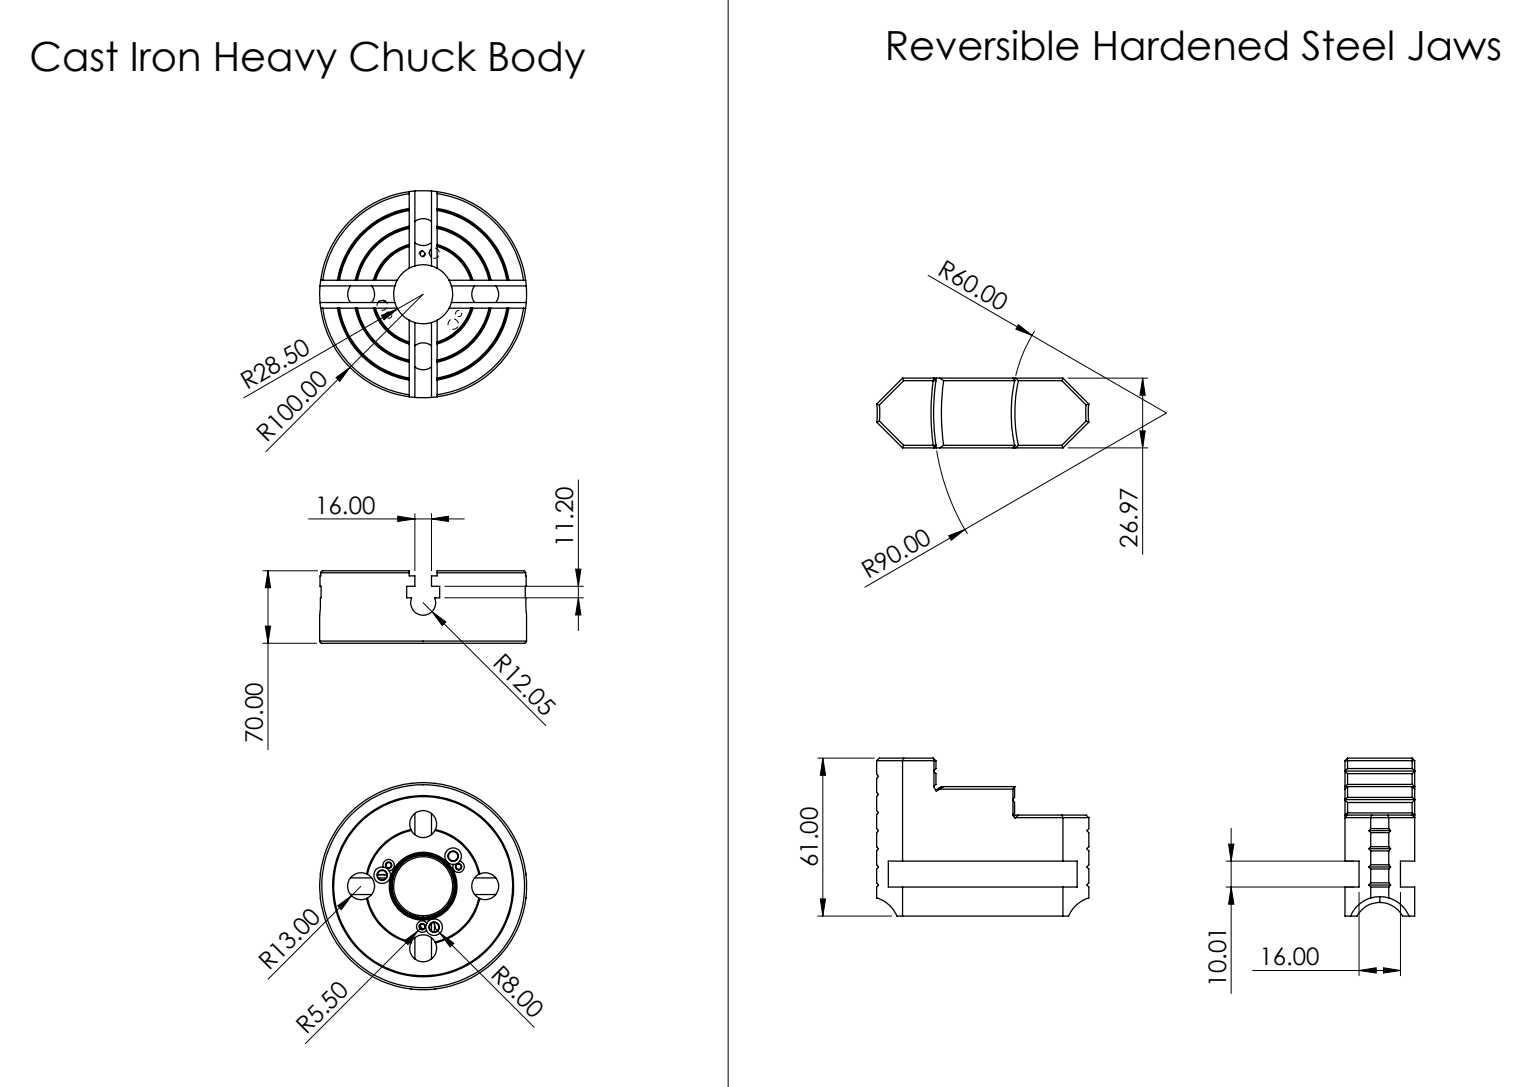
ISO-10303-21;
HEADER;
FILE_DESCRIPTION (('STEP AP214'),
    '1' );
FILE_NAME ('Cast Iron Heavy Chuck Body.step',
    '2026-10-09T08:48:44',
    ( '' ),
    ( '' ),
    'SwSTEP 2.0',
    'SolidWorks 2026',
    '' );
FILE_SCHEMA (( 'AUTOMOTIVE_DESIGN' ));
ENDSEC;

DATA;
#17=CARTESIAN_POINT ( 'NONE',  ( 3.210901138312283187, 2.729659904327170317, 0.5314960629921260393 ) ) ;
#22=EDGE_CURVE ( 'NONE', #75161, #32355, #82357, .T. ) ;
#61=ORIENTED_EDGE ( 'NONE', *, *, #30614, .T. ) ;
#78=FACE_OUTER_BOUND ( 'NONE', #30932, .T. ) ;
#83=ORIENTED_EDGE ( 'NONE', *, *, #43269, .T. ) ;
#95=CARTESIAN_POINT ( 'NONE',  ( 2.362204724409448620, 1.724409448818897461, 8.247593713802677664E-15 ) ) ;
#97=CARTESIAN_POINT ( 'NONE',  ( 3.935554666754304876, 1.075197191891656523, -0.1080298857917176142 ) ) ;
#98=EDGE_LOOP ( 'NONE', ( #67193, #53701, #56792, #76408 ) ) ;
#137=CARTESIAN_POINT ( 'NONE',  ( 1.067341128551216878, 1.212753000281105331, 0.3462674622822208836 ) ) ;
#152=CIRCLE ( 'NONE', #29714, 0.3149606299212598381 ) ;
#153=EDGE_CURVE ( 'NONE', #58154, #38787, #62911, .T. ) ;
#192=CIRCLE ( 'NONE', #6913, 0.3149606299212597826 ) ;
#213=ORIENTED_EDGE ( 'NONE', *, *, #72282, .F. ) ;
#238=EDGE_CURVE ( 'NONE', #62570, #82725, #55742, .T. ) ;
#251=AXIS2_PLACEMENT_3D ( 'NONE', #31198, #57691, #45055 ) ;
#278=EDGE_LOOP ( 'NONE', ( #70982, #45636, #76392, #46329 ) ) ;
#294=ORIENTED_EDGE ( 'NONE', *, *, #5614, .T. ) ;
#302=EDGE_CURVE ( 'NONE', #13567, #50475, #28771, .T. ) ;
#303=LINE ( 'NONE', #76901, #13349 ) ;
#312=VERTEX_POINT ( 'NONE', #80938 ) ;
#316=TOROIDAL_SURFACE ( 'NONE', #58028, 1.178877988035069047, 0.01968503937007873988 ) ;
#321=CARTESIAN_POINT ( 'NONE',  ( 2.165589143934496530, 1.494558157769224405, 0.4725443725032424380 ) ) ;
#334=CARTESIAN_POINT ( 'NONE',  ( -0.09693039542137318887, 1.072949718929360641, -1.590986883761158932 ) ) ;
#346=CARTESIAN_POINT ( 'NONE',  ( -1.024276469446319116, 1.664626768191372896, -0.4581463608586889835 ) ) ;
#368=ORIENTED_EDGE ( 'NONE', *, *, #43225, .F. ) ;
#369=CARTESIAN_POINT ( 'NONE',  ( 0.3149606299212637239, 2.165354330708661568, -1.076935383196056417 ) ) ;
#374=DIRECTION ( 'NONE',  ( 0.000000000000000000, -0.000000000000000000, 1.000000000000000000 ) ) ;
#377=CARTESIAN_POINT ( 'NONE',  ( 0.06179655389848991154, 1.065998012190817246, -3.936642156184892105 ) ) ;
#381=ORIENTED_EDGE ( 'NONE', *, *, #63426, .T. ) ;
#397=ORIENTED_EDGE ( 'NONE', *, *, #78869, .T. ) ;
#429=VECTOR ( 'NONE', #73458, 39.37007874015748143 ) ;
#436=DIRECTION ( 'NONE',  ( 0.000000000000000000, 1.000000000000000000, 0.000000000000000000 ) ) ;
#459=CARTESIAN_POINT ( 'NONE',  ( 0.4359958488159310086, 1.724409448818897461, 3.912791665790203766 ) ) ;
#472=CARTESIAN_POINT ( 'NONE',  ( -0.6299212598425164567, 2.165354330708661568, -0.9285414500055735321 ) ) ;
#483=CIRCLE ( 'NONE', #78489, 0.3149606299212597271 ) ;
#491=DIRECTION ( 'NONE',  ( 0.000000000000000000, 0.000000000000000000, -1.000000000000000000 ) ) ;
#502=CARTESIAN_POINT ( 'NONE',  ( -0.4477342634306575864, 1.379855024864608204, -2.114057166015708589 ) ) ;
#511=EDGE_CURVE ( 'NONE', #3191, #62716, #18015, .T. ) ;
#523=ORIENTED_EDGE ( 'NONE', *, *, #53975, .F. ) ;
#619=EDGE_LOOP ( 'NONE', ( #4517, #46542, #69561, #51297 ) ) ;
#623=DIRECTION ( 'NONE',  ( 0.000000000000000000, 1.000000000000000000, 0.000000000000000000 ) ) ;
#635=CARTESIAN_POINT ( 'NONE',  ( 0.1273213304869930951, 0.1377952755905511861, -1.680969278250197707 ) ) ;
#641=CARTESIAN_POINT ( 'NONE',  ( 0.000000000000000000, 2.677165354330708791, 0.000000000000000000 ) ) ;
#685=CARTESIAN_POINT ( 'NONE',  ( 0.4602852883866460076, 1.653403552777538366, 2.586150256253575197 ) ) ;
#697=ORIENTED_EDGE ( 'NONE', *, *, #58155, .F. ) ;
#698=ORIENTED_EDGE ( 'NONE', *, *, #49898, .F. ) ;
#712=VERTEX_POINT ( 'NONE', #12515 ) ;
#714=ORIENTED_EDGE ( 'NONE', *, *, #48541, .F. ) ;
#716=CONICAL_SURFACE ( 'NONE', #24907, 0.1771653543307085410, 1.029744258676653645 ) ;
#723=CARTESIAN_POINT ( 'NONE',  ( 3.224202737261815166, 2.716535433070866645, 0.5314960629921260393 ) ) ;
#725=AXIS2_PLACEMENT_3D ( 'NONE', #34776, #73071, #41496 ) ;
#733=EDGE_CURVE ( 'NONE', #7205, #57884, #50385, .T. ) ;
#741=CARTESIAN_POINT ( 'NONE',  ( -2.152447471807442891, 1.622068519643041551, 0.4668652553835654917 ) ) ;
#743=DIRECTION ( 'NONE',  ( 0.000000000000000000, 0.000000000000000000, 1.000000000000000000 ) ) ;
#754=CARTESIAN_POINT ( 'NONE',  ( 1.141392835773559211, 1.299212598425196985, 0.9642274814428540841 ) ) ;
#766=PLANE ( 'NONE',  #65364 ) ;
#772=DIRECTION ( 'NONE',  ( 0.000000000000000000, 0.000000000000000000, 1.000000000000000000 ) ) ;
#779=VECTOR ( 'NONE', #35095, 39.37007874015748143 ) ;
#790=ADVANCED_FACE ( 'NONE', ( #76083 ), #69761, .F. ) ;
#803=ORIENTED_EDGE ( 'NONE', *, *, #65634, .F. ) ;
#805=ORIENTED_EDGE ( 'NONE', *, *, #65450, .T. ) ;
#822=AXIS2_PLACEMENT_3D ( 'NONE', #34394, #67220, #78191 ) ;
#825=AXIS2_PLACEMENT_3D ( 'NONE', #7918, #52916, #78631 ) ;
#828=CARTESIAN_POINT ( 'NONE',  ( 2.750540364621160361, 1.199841186584418518, -0.3336616047370271065 ) ) ;
#858=CARTESIAN_POINT ( 'NONE',  ( -0.5314960629921122726, 2.755905511811024056, -3.937007874015763687 ) ) ;
#876=DIRECTION ( 'NONE',  ( -0.000000000000000000, -1.000000000000000000, 0.000000000000000000 ) ) ;
#884=AXIS2_PLACEMENT_3D ( 'NONE', #26992, #71617, #52655 ) ;
#886=AXIS2_PLACEMENT_3D ( 'NONE', #7786, #38921, #40179 ) ;
#890=EDGE_CURVE ( 'NONE', #78998, #7122, #78646, .T. ) ;
#901=CARTESIAN_POINT ( 'NONE',  ( 0.4359958488159797474, 1.724409448818897905, -2.094141031014984833 ) ) ;
#929=ORIENTED_EDGE ( 'NONE', *, *, #10585, .T. ) ;
#932=EDGE_LOOP ( 'NONE', ( #23051, #15115, #31365, #8595 ) ) ;
#945=CARTESIAN_POINT ( 'NONE',  ( -0.5314960629921398061, 2.687614851728676424, 3.900966923095589234 ) ) ;
#946=CONICAL_SURFACE ( 'NONE', #61424, 1.250000000000000000, 0.1221730476396033355 ) ;
#948=DIRECTION ( 'NONE',  ( -0.000000000000000000, -1.000000000000000000, -0.000000000000000000 ) ) ;
#950=AXIS2_PLACEMENT_3D ( 'NONE', #7471, #12953, #25977 ) ;
#962=DIRECTION ( 'NONE',  ( 0.000000000000000000, 0.000000000000000000, -1.000000000000000000 ) ) ;
#984=B_SPLINE_CURVE_WITH_KNOTS ( 'NONE', 3,
 ( #68449, #81500, #10385, #37680, #36449, #62954, #50304, #24225, #61714, #57026, #56618, #36863 ),
 .UNSPECIFIED., .F., .F.,
 ( 4, 2, 2, 2, 2, 4 ),
 ( 0.007992874908875213444, 0.009303755029337302043, 0.01061463514979939064, 0.01192551527026147924, 0.01258095533049252354, 0.01323639539072356784 ),
 .UNSPECIFIED. ) ;
#986=CARTESIAN_POINT ( 'NONE',  ( 1.019692277575655615, 1.459399361446979126, -0.4682193611689622892 ) ) ;
#989=CARTESIAN_POINT ( 'NONE',  ( 0.4116877677584974138, 1.299622705822838453, 3.915462153828698888 ) ) ;
#995=ADVANCED_FACE ( 'NONE', ( #71847 ), #78589, .F. ) ;
#1024=CARTESIAN_POINT ( 'NONE',  ( 4.821444151489972621E-16, 1.062992125984252745, 3.937007874015748143 ) ) ;
#1043=ORIENTED_EDGE ( 'NONE', *, *, #78852, .T. ) ;
#1046=DIRECTION ( 'NONE',  ( 0.000000000000000000, -0.000000000000000000, 1.000000000000000000 ) ) ;
#1047=DIRECTION ( 'NONE',  ( 1.492469013153037857E-17, -0.9925461516413219831, 0.1218693434051477398 ) ) ;
#1048=FACE_OUTER_BOUND ( 'NONE', #12186, .T. ) ;
#1052=CARTESIAN_POINT ( 'NONE',  ( 0.4711392887345147162, 1.601500657493326152, -3.908721069869979026 ) ) ;
#1055=VERTEX_POINT ( 'NONE', #7876 ) ;
#1092=FACE_OUTER_BOUND ( 'NONE', #21318, .T. ) ;
#1095=CARTESIAN_POINT ( 'NONE',  ( 0.000000000000000000, 2.755905511811024056, 0.000000000000000000 ) ) ;
#1124=ORIENTED_EDGE ( 'NONE', *, *, #39342, .F. ) ;
#1130=DIRECTION ( 'NONE',  ( 0.000000000000000000, -0.6427876096865366984, -0.7660444431189802339 ) ) ;
#1139=ORIENTED_EDGE ( 'NONE', *, *, #22849, .T. ) ;
#1159=ORIENTED_EDGE ( 'NONE', *, *, #69637, .F. ) ;
#1166=LINE ( 'NONE', #52475, #66762 ) ;
#1174=DIRECTION ( 'NONE',  ( -0.000000000000000000, 1.734723475976808327E-16, 1.000000000000000000 ) ) ;
#1187=B_SPLINE_CURVE_WITH_KNOTS ( 'NONE', 3,
 ( #54995, #8742, #74380, #67239 ),
 .UNSPECIFIED., .F., .F.,
 ( 4, 4 ),
 ( 0.1688788475280605661, 0.1702663099542993941 ),
 .UNSPECIFIED. ) ;
#1196=CARTESIAN_POINT ( 'NONE',  ( 3.937007874015748143, 2.559055118110236560, 0.5314960629921260393 ) ) ;
#1207=CARTESIAN_POINT ( 'NONE',  ( -3.937007874015748143, 1.537401574803149984, -2.901595197523589142E-16 ) ) ;
#1214=FACE_BOUND ( 'NONE', #26809, .T. ) ;
#1220=FACE_OUTER_BOUND ( 'NONE', #57084, .T. ) ;
#1221=EDGE_CURVE ( 'NONE', #16864, #33327, #33540, .T. ) ;
#1224=CARTESIAN_POINT ( 'NONE',  ( 0.4622706148242299307, 1.429654486764701193, -3.909775711958814348 ) ) ;
#1240=EDGE_CURVE ( 'NONE', #12200, #44534, #303, .T. ) ;
#1245=ORIENTED_EDGE ( 'NONE', *, *, #82772, .T. ) ;
#1248=CARTESIAN_POINT ( 'NONE',  ( 2.759994995438110443, 1.188885443925058238, 0.3231744412229853869 ) ) ;
#1287=DIRECTION ( 'NONE',  ( -1.000000000000000000, -0.000000000000000000, -0.000000000000000000 ) ) ;
#1306=DIRECTION ( 'NONE',  ( 0.000000000000000000, 0.000000000000000000, -1.000000000000000000 ) ) ;
#1318=CARTESIAN_POINT ( 'NONE',  ( 0.5314960629921156032, 0.000000000000000000, 0.9881811337016697117 ) ) ;
#1323=CARTESIAN_POINT ( 'NONE',  ( 1.348312163386739426, 1.062992125984252079, 0.7386866130305692613 ) ) ;
#1327=ORIENTED_EDGE ( 'NONE', *, *, #22709, .T. ) ;
#1330=ORIENTED_EDGE ( 'NONE', *, *, #56817, .F. ) ;
#1345=EDGE_LOOP ( 'NONE', ( #66456, #45202, #47720, #72344 ) ) ;
#1362=CARTESIAN_POINT ( 'NONE',  ( 3.915483736577200613, 1.300266479744685899, -0.4111838468780947276 ) ) ;
#1367=CARTESIAN_POINT ( 'NONE',  ( 0.6299212598425235621, 0.000000000000000000, -0.9285414500055687581 ) ) ;
#1370=EDGE_CURVE ( 'NONE', #22431, #62933, #19231, .T. ) ;
#1388=CARTESIAN_POINT ( 'NONE',  ( 0.5314960629921070545, 2.755905511811024056, 1.813482582612299110 ) ) ;
#1433=CARTESIAN_POINT ( 'NONE',  ( -0.4724922890202599146, 1.580837543196282446, -2.165463280039293892 ) ) ;
#1456=DIRECTION ( 'NONE',  ( -1.687538997430237941E-14, 0.000000000000000000, -1.000000000000000000 ) ) ;
#1457=CARTESIAN_POINT ( 'NONE',  ( -0.008542603271839102619, 1.062992125984252301, 2.874015748031496731 ) ) ;
#1465=ORIENTED_EDGE ( 'NONE', *, *, #46764, .T. ) ;
#1468=CARTESIAN_POINT ( 'NONE',  ( -1.074107865122115868, 1.191152302059476087, -0.3246720348184669591 ) ) ;
#1477=CARTESIAN_POINT ( 'NONE',  ( -0.5314960629921193780, 2.755905511811024056, -1.895394334970793793 ) ) ;
#1494=FACE_OUTER_BOUND ( 'NONE', #73999, .T. ) ;
#1523=CARTESIAN_POINT ( 'NONE',  ( 0.2491324880211018833, 1.133662664435919787, -1.613879522126778543 ) ) ;
#1535=ORIENTED_EDGE ( 'NONE', *, *, #67469, .T. ) ;
#1542=CIRCLE ( 'NONE', #5549, 0.2165354330708660069 ) ;
#1551=ORIENTED_EDGE ( 'NONE', *, *, #64100, .T. ) ;
#1553=ORIENTED_EDGE ( 'NONE', *, *, #33853, .T. ) ;
#1559=CARTESIAN_POINT ( 'NONE',  ( 1.019861537960135234, 1.617630162216313172, -0.4678516549211681474 ) ) ;
#1565=CARTESIAN_POINT ( 'NONE',  ( 0.4706608522957150820, 1.597527518877488450, 2.161121219943100691 ) ) ;
#1571=VERTEX_POINT ( 'NONE', #58153 ) ;
#1578=CARTESIAN_POINT ( 'NONE',  ( -2.094141031015012366, 1.724409448818897905, 0.4359958488159718093 ) ) ;
#1585=CARTESIAN_POINT ( 'NONE',  ( 1.141392835773559211, 1.299212598425196985, 1.318558190104271333 ) ) ;
#1601=CARTESIAN_POINT ( 'NONE',  ( 0.000000000000000000, 0.03937007874015747977, 0.000000000000000000 ) ) ;
#1618=CARTESIAN_POINT ( 'NONE',  ( 0.5314960629920926216, 2.755905511811024056, 3.184294706754636106 ) ) ;
#1630=CARTESIAN_POINT ( 'NONE',  ( 0.3567317632078913503, 1.224270319509463301, -3.920825516433590785 ) ) ;
#1634=ORIENTED_EDGE ( 'NONE', *, *, #46015, .T. ) ;
#1656=FACE_OUTER_BOUND ( 'NONE', #7657, .T. ) ;
#1689=DIRECTION ( 'NONE',  ( -3.491481338843132961E-15, -0.000000000000000000, 1.000000000000000000 ) ) ;
#1700=CIRCLE ( 'NONE', #48719, 3.937007874015748143 ) ;
#1705=ADVANCED_FACE ( 'NONE', ( #45099, #71223 ), #51837, .T. ) ;
#1707=EDGE_CURVE ( 'NONE', #26586, #5038, #58582, .T. ) ;
#1733=FACE_OUTER_BOUND ( 'NONE', #53462, .T. ) ;
#1736=ORIENTED_EDGE ( 'NONE', *, *, #32413, .F. ) ;
#1745=CARTESIAN_POINT ( 'NONE',  ( -0.4562819726585397584, 1.668167360224330098, -2.594269413088675424 ) ) ;
#1769=CARTESIAN_POINT ( 'NONE',  ( -0.5314960629921394730, 2.739927440807262915, 3.869764100875847213 ) ) ;
#1770=ADVANCED_FACE ( 'NONE', ( #38806 ), #5298, .F. ) ;
#1776=CARTESIAN_POINT ( 'NONE',  ( -2.362204724409448620, 1.724409448818897905, -2.474278114140802984E-14 ) ) ;
#1782=DIRECTION ( 'NONE',  ( -0.000000000000000000, 1.000000000000000000, 0.000000000000000000 ) ) ;
#1803=AXIS2_PLACEMENT_3D ( 'NONE', #45032, #46717, #40005 ) ;
#1807=CARTESIAN_POINT ( 'NONE',  ( 1.087314056648182925, 1.152187173028865974, -0.2773278579668389532 ) ) ;
#1818=CIRCLE ( 'NONE', #70341, 0.3149606299212598381 ) ;
#1836=DIRECTION ( 'NONE',  ( -0.000000000000000000, -1.000000000000000000, -0.000000000000000000 ) ) ;
#1837=ADVANCED_FACE ( 'NONE', ( #71639 ), #72478, .F. ) ;
#1862=EDGE_CURVE ( 'NONE', #53393, #21631, #12276, .T. ) ;
#1866=ORIENTED_EDGE ( 'NONE', *, *, #27189, .T. ) ;
#1871=DIRECTION ( 'NONE',  ( -0.000000000000000000, -1.000000000000000000, -0.000000000000000000 ) ) ;
#1874=VECTOR ( 'NONE', #6880, 39.37007874015748143 ) ;
#1876=CARTESIAN_POINT ( 'NONE',  ( 0.4615285972131335512, 1.648351240186696431, -3.909863522152617232 ) ) ;
#1888=ORIENTED_EDGE ( 'NONE', *, *, #11147, .T. ) ;
#1890=CARTESIAN_POINT ( 'NONE',  ( -1.854472803289052507, 2.716535433070866645, 0.5314960629921260393 ) ) ;
#1933=EDGE_CURVE ( 'NONE', #33346, #9070, #6605, .T. ) ;
#1935=AXIS2_PLACEMENT_3D ( 'NONE', #68198, #57178, #10937 ) ;
#1937=CARTESIAN_POINT ( 'NONE',  ( 0.2565672512708053188, 1.138339430604204061, -1.632951123234252400 ) ) ;
#1962=ORIENTED_EDGE ( 'NONE', *, *, #9565, .T. ) ;
#1987=CARTESIAN_POINT ( 'NONE',  ( 1.851299440327910162, 1.063968899401424251, 0.03484477857460829137 ) ) ;
#1994=CARTESIAN_POINT ( 'NONE',  ( -1.559171609364246924, 0.3937007874015747699, 0.4177787735906735578 ) ) ;
#2011=CARTESIAN_POINT ( 'NONE',  ( 0.4437451894543472664, 1.369490053320156830, -1.614267692121933440 ) ) ;
#2013=DIRECTION ( 'NONE',  ( 0.000000000000000000, 0.000000000000000000, -1.000000000000000000 ) ) ;
#2017=DIRECTION ( 'NONE',  ( 0.000000000000000000, -1.000000000000000000, 0.000000000000000000 ) ) ;
#2019=DIRECTION ( 'NONE',  ( -1.000000000000000000, -0.000000000000000000, -0.000000000000000000 ) ) ;
#2027=LINE ( 'NONE', #8344, #38709 ) ;
#2034=CARTESIAN_POINT ( 'NONE',  ( -3.884512598959606322, 2.725419031863056230, -0.5314960629921259283 ) ) ;
#2042=DIRECTION ( 'NONE',  ( 8.673617379884022653E-16, -1.000000000000000000, 3.028377322213053966E-30 ) ) ;
#2043=CARTESIAN_POINT ( 'NONE',  ( 3.873860110281697189, 2.736617272820978553, 0.5314960629921261503 ) ) ;
#2045=EDGE_LOOP ( 'NONE', ( #714, #16160, #27121, #63760 ) ) ;
#2046=AXIS2_PLACEMENT_3D ( 'NONE', #6092, #12837, #33442 ) ;
#2048=ORIENTED_EDGE ( 'NONE', *, *, #25941, .F. ) ;
#2067=CARTESIAN_POINT ( 'NONE',  ( 2.565164815102312534, 1.469861850861822861, 0.4698711669589720197 ) ) ;
#2075=CARTESIAN_POINT ( 'NONE',  ( -2.554262525012342966, 1.537401574803149984, -0.4744094488188975722 ) ) ;
#2108=CARTESIAN_POINT ( 'NONE',  ( 0.5314960629920850721, 2.687524476698321507, 3.900447471620236861 ) ) ;
#2120=EDGE_CURVE ( 'NONE', #49642, #43005, #35002, .T. ) ;
#2133=CARTESIAN_POINT ( 'NONE',  ( 1.348312163386739426, 0.2755905511811023723, 0.5221511799597032821 ) ) ;
#2139=DIRECTION ( 'NONE',  ( -3.491481338843133355E-15, -0.000000000000000000, 1.000000000000000000 ) ) ;
#2145=AXIS2_PLACEMENT_3D ( 'NONE', #68264, #30762, #4670 ) ;
#2167=ORIENTED_EDGE ( 'NONE', *, *, #61841, .T. ) ;
#2182=CARTESIAN_POINT ( 'NONE',  ( 0.5314960629920847390, 2.755905511811024056, 3.937007874015794773 ) ) ;
#2184=CARTESIAN_POINT ( 'NONE',  ( -0.3149606299212733829, 2.559055118110236560, 3.924389226575467404 ) ) ;
#2187=CARTESIAN_POINT ( 'NONE',  ( 3.936627864294173218, 1.066117803576733358, -0.06254616550773663131 ) ) ;
#2210=AXIS2_PLACEMENT_3D ( 'NONE', #55831, #54600, #81949 ) ;
#2211=CIRCLE ( 'NONE', #886, 0.5118110236220471121 ) ;
#2212=FACE_OUTER_BOUND ( 'NONE', #52049, .T. ) ;
#2226=CARTESIAN_POINT ( 'NONE',  ( 0.1077486724431487297, 1.075126265569047890, 3.935562984763014249 ) ) ;
#2265=AXIS2_PLACEMENT_3D ( 'NONE', #17616, #80218, #81040 ) ;
#2295=VERTEX_POINT ( 'NONE', #38416 ) ;
#2297=CARTESIAN_POINT ( 'NONE',  ( -1.035641998995818547, 1.340358236468215392, -0.4318304824445497458 ) ) ;
#2299=CARTESIAN_POINT ( 'NONE',  ( 0.4177787735907000366, 1.299212598425196985, -1.736336963694947944 ) ) ;
#2304=ORIENTED_EDGE ( 'NONE', *, *, #153, .T. ) ;
#2306=FACE_OUTER_BOUND ( 'NONE', #9636, .T. ) ;
#2322=CIRCLE ( 'NONE', #27852, 0.1190944881889763746 ) ;
#2368=ORIENTED_EDGE ( 'NONE', *, *, #32892, .F. ) ;
#2386=VERTEX_POINT ( 'NONE', #1388 ) ;
#2403=ORIENTED_EDGE ( 'NONE', *, *, #16301, .F. ) ;
#2406=DIRECTION ( 'NONE',  ( 0.000000000000000000, 0.000000000000000000, 1.000000000000000000 ) ) ;
#2408=CARTESIAN_POINT ( 'NONE',  ( 1.863753233923691965, 1.077434660671932942, -0.1173752429317785756 ) ) ;
#2415=CARTESIAN_POINT ( 'NONE',  ( 0.4498537592782897998, 0.000000000000000000, 2.118110236220472675 ) ) ;
#2416=EDGE_CURVE ( 'NONE', #61855, #9282, #51866, .T. ) ;
#2443=EDGE_LOOP ( 'NONE', ( #26697, #75686, #7352, #68019 ) ) ;
#2447=CIRCLE ( 'NONE', #37334, 3.267716535433071279 ) ;
#2456=CARTESIAN_POINT ( 'NONE',  ( 0.4741627488320241390, 1.554989095716459380, -2.554874958603176704 ) ) ;
#2469=ORIENTED_EDGE ( 'NONE', *, *, #21253, .T. ) ;
#2488=CARTESIAN_POINT ( 'NONE',  ( 2.647175254740889105, 1.326002914239470920, 0.4256865378621380591 ) ) ;
#2494=CARTESIAN_POINT ( 'NONE',  ( 0.3149606299212185934, 2.755905511811024056, 3.924389226575471845 ) ) ;
#2523=DIRECTION ( 'NONE',  ( -0.000000000000000000, -1.000000000000000000, -0.000000000000000000 ) ) ;
#2529=CARTESIAN_POINT ( 'NONE',  ( -2.131037067002753194, 1.408244132531263570, -0.4567322424080928478 ) ) ;
#2567=ORIENTED_EDGE ( 'NONE', *, *, #11147, .F. ) ;
#2585=VERTEX_POINT ( 'NONE', #45972 ) ;
#2601=LINE ( 'NONE', #79218, #82724 ) ;
#2606=CARTESIAN_POINT ( 'NONE',  ( 3.936638708481129623, 1.066027760652975553, 0.06186723695104996007 ) ) ;
#2614=VECTOR ( 'NONE', #59202, 39.37007874015748143 ) ;
#2618=PLANE ( 'NONE',  #39133 ) ;
#2660=CARTESIAN_POINT ( 'NONE',  ( 2.138346301250393822, 1.653225543546886112, -0.4603267246303516802 ) ) ;
#2665=ORIENTED_EDGE ( 'NONE', *, *, #46607, .T. ) ;
#2678=CARTESIAN_POINT ( 'NONE',  ( -0.4732023222440167043, 1.572318554836807936, -2.167187561710682608 ) ) ;
#2694=DIRECTION ( 'NONE',  ( 1.000000000000000000, -0.000000000000000000, -0.000000000000000000 ) ) ;
#2696=EDGE_LOOP ( 'NONE', ( #66226, #52117, #33223, #17176, #68911, #34788, #10944, #71203, #15875, #69962, #67305, #18404, #77329, #39611 ) ) ;
#2701=DIRECTION ( 'NONE',  ( -0.000000000000000000, -1.000000000000000000, -0.000000000000000000 ) ) ;
#2702=FACE_OUTER_BOUND ( 'NONE', #52644, .T. ) ;
#2718=DIRECTION ( 'NONE',  ( -0.000000000000000000, -1.000000000000000000, -0.000000000000000000 ) ) ;
#2735=ADVANCED_FACE ( 'NONE', ( #14444 ), #65368, .F. ) ;
#2747=DIRECTION ( 'NONE',  ( -0.000000000000000000, -1.000000000000000000, -0.000000000000000000 ) ) ;
#2750=CARTESIAN_POINT ( 'NONE',  ( -1.854472803289052507, 2.716535433070866645, 0.5314960629921260393 ) ) ;
#2780=VERTEX_POINT ( 'NONE', #27879 ) ;
#2800=CARTESIAN_POINT ( 'NONE',  ( -1.496204327613243068, 1.365504603163548047, 0.4422373666565095895 ) ) ;
#2804=CARTESIAN_POINT ( 'NONE',  ( 1.028575266362749208, 1.695109487299528261, -0.4485632242333315589 ) ) ;
#2805=DIRECTION ( 'NONE',  ( -0.8660254037844431485, 0.000000000000000000, 0.4999999999999918954 ) ) ;
#2816=FACE_BOUND ( 'NONE', #44463, .T. ) ;
#2819=LINE ( 'NONE', #34387, #49252 ) ;
#2863=VECTOR ( 'NONE', #13796, 39.37007874015748143 ) ;
#2874=CARTESIAN_POINT ( 'NONE',  ( 3.881211926161857395, 2.729373344522950884, 0.5314960629921260393 ) ) ;
#2876=EDGE_CURVE ( 'NONE', #59294, #78599, #21767, .T. ) ;
#2896=ORIENTED_EDGE ( 'NONE', *, *, #31624, .T. ) ;
#2899=DIRECTION ( 'NONE',  ( 0.000000000000000000, -1.000000000000000000, 0.000000000000000000 ) ) ;
#2905=CARTESIAN_POINT ( 'NONE',  ( 0.000000000000000000, 2.755905511811024056, 0.000000000000000000 ) ) ;
#2910=VERTEX_POINT ( 'NONE', #48057 ) ;
#2935=CARTESIAN_POINT ( 'NONE',  ( -1.313877454013331780, 0.2755905511811023723, 0.6792347910202041206 ) ) ;
#2940=CARTESIAN_POINT ( 'NONE',  ( -2.058022911372341834, 1.301102360844738515, -0.4123394245947631376 ) ) ;
#2964=DIRECTION ( 'NONE',  ( -0.000000000000000000, -1.000000000000000000, -0.000000000000000000 ) ) ;
#2967=AXIS2_PLACEMENT_3D ( 'NONE', #5229, #75124, #23343 ) ;
#2974=DIRECTION ( 'NONE',  ( 0.000000000000000000, 0.000000000000000000, -1.000000000000000000 ) ) ;
#2982=ORIENTED_EDGE ( 'NONE', *, *, #64100, .F. ) ;
#3013=CARTESIAN_POINT ( 'NONE',  ( -0.5314960629921371416, 2.742783271717982974, 3.197598480811213673 ) ) ;
#3034=DIRECTION ( 'NONE',  ( 0.000000000000000000, 0.000000000000000000, -1.000000000000000000 ) ) ;
#3066=CARTESIAN_POINT ( 'NONE',  ( 0.000000000000000000, 0.03937007874015747977, 0.000000000000000000 ) ) ;
#3113=LINE ( 'NONE', #40166, #43760 ) ;
#3121=VERTEX_POINT ( 'NONE', #48465 ) ;
#3126=CARTESIAN_POINT ( 'NONE',  ( 0.000000000000000000, 2.165354330708661568, 0.000000000000000000 ) ) ;
#3131=CARTESIAN_POINT ( 'NONE',  ( -1.313877454013331780, 0.2755905511811023723, 0.7983292792091805090 ) ) ;
#3178=CIRCLE ( 'NONE', #34119, 3.937007874015748143 ) ;
#3190=ORIENTED_EDGE ( 'NONE', *, *, #52265, .T. ) ;
#3191=VERTEX_POINT ( 'NONE', #81725 ) ;
#3209=EDGE_LOOP ( 'NONE', ( #41488, #68601, #43311, #7771, #25736, #17193, #15767, #68017 ) ) ;
#3212=CARTESIAN_POINT ( 'NONE',  ( -1.576474796205048490, 1.384328893707485131, 0.4490365374974934487 ) ) ;
#3226=EDGE_LOOP ( 'NONE', ( #28969, #55849, #31093, #69712 ) ) ;
#3243=AXIS2_PLACEMENT_3D ( 'NONE', #4335, #3934, #28352 ) ;
#3247=UNCERTAINTY_MEASURE_WITH_UNIT (LENGTH_MEASURE( 1.000000000000000082E-05 ), #79023, 'distance_accuracy_value', 'NONE');
#3261=CARTESIAN_POINT ( 'NONE',  ( 3.937007874015748143, 2.559055118110236560, 0.3149606299212599492 ) ) ;
#3293=VECTOR ( 'NONE', #63232, 39.37007874015748143 ) ;
#3304=EDGE_LOOP ( 'NONE', ( #4196, #61026, #70766 ) ) ;
#3314=CARTESIAN_POINT ( 'NONE',  ( 0.4744094488188940750, 1.537401574803149984, 1.016821367227985329 ) ) ;
#3319=EDGE_LOOP ( 'NONE', ( #38671, #58428, #41407 ) ) ;
#3348=CARTESIAN_POINT ( 'NONE',  ( -1.916165371950965257, 1.134815007188454627, -0.2514610820057113783 ) ) ;
#3376=CARTESIAN_POINT ( 'NONE',  ( 3.937007874015748143, 2.559055118110236560, -0.3149606299212596716 ) ) ;
#3377=VERTEX_POINT ( 'NONE', #75808 ) ;
#3381=CARTESIAN_POINT ( 'NONE',  ( 0.2893625497513035438, 1.161323636346416777, -1.436460574497700371 ) ) ;
#3387=FACE_OUTER_BOUND ( 'NONE', #20860, .T. ) ;
#3406=CARTESIAN_POINT ( 'NONE',  ( 0.1341302950245132075, 1.082049466318357300, -2.856398576552468427 ) ) ;
#3468=CARTESIAN_POINT ( 'NONE',  ( 1.895394334970792016, 2.755905511811024056, 0.5314960629921260393 ) ) ;
#3477=DIRECTION ( 'NONE',  ( 0.000000000000000000, 1.000000000000000000, -0.000000000000000000 ) ) ;
#3479=DIRECTION ( 'NONE',  ( -0.000000000000000000, 1.000000000000000000, -0.000000000000000000 ) ) ;
#3481=CARTESIAN_POINT ( 'NONE',  ( 1.348312163386739426, 1.062992125984252079, 0.7386866130305692613 ) ) ;
#3522=CIRCLE ( 'NONE', #25000, 0.1190944881889763746 ) ;
#3526=CONICAL_SURFACE ( 'NONE', #50531, 1.889763779527559251, 0.7853981633974500554 ) ;
#3527=DIRECTION ( 'NONE',  ( -1.000000000000000000, -8.326672684688674053E-16, 0.000000000000000000 ) ) ;
#3530=DIRECTION ( 'NONE',  ( -0.000000000000000000, -1.000000000000000000, -0.000000000000000000 ) ) ;
#3546=VECTOR ( 'NONE', #11617, 39.37007874015748143 ) ;
#3552=EDGE_CURVE ( 'NONE', #23894, #61368, #47286, .T. ) ;
#3574=CARTESIAN_POINT ( 'NONE',  ( 0.4698793137518422203, 1.469922167998567897, 2.159263675096192436 ) ) ;
#3583=AXIS2_PLACEMENT_3D ( 'NONE', #3131, #56113, #9860 ) ;
#3624=ORIENTED_EDGE ( 'NONE', *, *, #22798, .T. ) ;
#3629=CARTESIAN_POINT ( 'NONE',  ( 0.1406185367545949305, 0.1377952755905511861, -1.409564117849439802 ) ) ;
#3643=AXIS2_PLACEMENT_3D ( 'NONE', #28529, #34855, #29357 ) ;
#3645=CARTESIAN_POINT ( 'NONE',  ( 1.852066570651488719, 1.064797240280316748, -0.04222672046128581047 ) ) ;
#3652=CONICAL_SURFACE ( 'NONE', #14421, 3.307086614173228689, 0.7853981633974500554 ) ;
#3653=CIRCLE ( 'NONE', #62764, 1.122047244094488194 ) ;
#3676=CARTESIAN_POINT ( 'NONE',  ( -3.900966923095589678, 2.755905511811024056, -0.5314960629921260393 ) ) ;
#3698=CARTESIAN_POINT ( 'NONE',  ( -3.908814775713581824, 1.601606672327087644, 0.4703198478456566689 ) ) ;
#3729=LINE ( 'NONE', #15961, #52508 ) ;
#3737=ORIENTED_EDGE ( 'NONE', *, *, #58775, .T. ) ;
#3739=CARTESIAN_POINT ( 'NONE',  ( 0.000000000000000000, 1.724409448818897461, 0.000000000000000000 ) ) ;
#3757=CARTESIAN_POINT ( 'NONE',  ( -3.184294706754630777, 2.755905511811024056, -0.5314960629921260393 ) ) ;
#3761=CIRCLE ( 'NONE', #13197, 1.122047244094488194 ) ;
#3763=CARTESIAN_POINT ( 'NONE',  ( -1.854728618660363759, 1.067671560069311854, -0.06860298820093484184 ) ) ;
#3772=FACE_OUTER_BOUND ( 'NONE', #65740, .T. ) ;
#3774=EDGE_CURVE ( 'NONE', #41297, #24318, #70174, .T. ) ;
#3777=EDGE_CURVE ( 'NONE', #24500, #32357, #56713, .T. ) ;
#3790=CARTESIAN_POINT ( 'NONE',  ( -2.543486866223389153, 2.716535433070866645, 0.5314960629921260393 ) ) ;
#3791=ORIENTED_EDGE ( 'NONE', *, *, #67416, .F. ) ;
#3796=LINE ( 'NONE', #60621, #21602 ) ;
#3802=EDGE_CURVE ( 'NONE', #17115, #33549, #49990, .T. ) ;
#3805=ORIENTED_EDGE ( 'NONE', *, *, #36169, .T. ) ;
#3819=CARTESIAN_POINT ( 'NONE',  ( 0.4102808022082889416, 1.299212598425196985, -1.382164990278189398 ) ) ;
#3827=VECTOR ( 'NONE', #51170, 39.37007874015748143 ) ;
#3861=CARTESIAN_POINT ( 'NONE',  ( -0.4682236582119034263, 1.459426199372924948, -1.019690296884233849 ) ) ;
#3882=CARTESIAN_POINT ( 'NONE',  ( 0.000000000000000000, 2.755905511811024056, 0.000000000000000000 ) ) ;
#3893=EDGE_CURVE ( 'NONE', #60217, #66675, #29271, .T. ) ;
#3895=DIRECTION ( 'NONE',  ( 0.000000000000000000, -1.000000000000000000, 0.000000000000000000 ) ) ;
#3897=CARTESIAN_POINT ( 'NONE',  ( 2.130163876374006282, 1.668131542012052826, -0.4562955581495580781 ) ) ;
#3907=PLANE ( 'NONE',  #56060 ) ;
#3908=CARTESIAN_POINT ( 'NONE',  ( 0.5314960629921371416, 2.729659904327171205, -3.210901138312280523 ) ) ;
#3923=VECTOR ( 'NONE', #23902, 39.37007874015748143 ) ;
#3934=DIRECTION ( 'NONE',  ( -0.000000000000000000, -1.000000000000000000, 0.000000000000000000 ) ) ;
#3943=FACE_OUTER_BOUND ( 'NONE', #54517, .T. ) ;
#3955=DIRECTION ( 'NONE',  ( 0.000000000000000000, 1.000000000000000000, -8.673617379884024625E-16 ) ) ;
#3987=CARTESIAN_POINT ( 'NONE',  ( 0.4725553370316598056, 1.494684982616659275, 2.165615670503216794 ) ) ;
#4040=CARTESIAN_POINT ( 'NONE',  ( -0.5314960629921324786, 2.716535433070866645, 1.854472803289050509 ) ) ;
#4041=DIRECTION ( 'NONE',  ( 0.000000000000000000, -1.000000000000000000, -1.408710688920637755E-15 ) ) ;
#4042=CARTESIAN_POINT ( 'NONE',  ( 0.9285414500055708675, 0.000000000000000000, 0.6299212598425202314 ) ) ;
#4078=CARTESIAN_POINT ( 'NONE',  ( 3.197598479107677694, 2.742783273398275767, -0.5314960629921260393 ) ) ;
#4095=AXIS2_PLACEMENT_3D ( 'NONE', #22085, #78520, #66295 ) ;
#4102=EDGE_CURVE ( 'NONE', #59692, #37337, #74231, .T. ) ;
#4111=ORIENTED_EDGE ( 'NONE', *, *, #15570, .T. ) ;
#4112=EDGE_CURVE ( 'NONE', #40260, #33327, #71513, .T. ) ;
#4129=DIRECTION ( 'NONE',  ( 0.000000000000000000, -1.000000000000000000, 0.000000000000000000 ) ) ;
#4135=DIRECTION ( 'NONE',  ( 1.047444401652940007E-14, -0.000000000000000000, -1.000000000000000000 ) ) ;
#4140=VERTEX_POINT ( 'NONE', #23240 ) ;
#4142=DIRECTION ( 'NONE',  ( -3.491481338843132961E-15, -0.000000000000000000, 1.000000000000000000 ) ) ;
#4143=ORIENTED_EDGE ( 'NONE', *, *, #24144, .T. ) ;
#4145=DIRECTION ( 'NONE',  ( 0.000000000000000000, 1.000000000000000000, -0.000000000000000000 ) ) ;
#4149=CARTESIAN_POINT ( 'NONE',  ( -0.06215213303350786145, 1.066820816534554961, 3.936548056194433265 ) ) ;
#4176=ADVANCED_FACE ( 'NONE', ( #74192 ), #33900, .T. ) ;
#4189=FACE_OUTER_BOUND ( 'NONE', #46215, .T. ) ;
#4195=DIRECTION ( 'NONE',  ( -0.000000000000000000, -1.000000000000000000, -0.000000000000000000 ) ) ;
#4196=ORIENTED_EDGE ( 'NONE', *, *, #45967, .F. ) ;
#4211=EDGE_LOOP ( 'NONE', ( #5382, #28024, #47075, #2567 ) ) ;
#4225=EDGE_LOOP ( 'NONE', ( #17684, #71836, #29859, #26567, #54119, #10477, #4938, #19031, #39331, #65925, #4973, #83294, #3190, #37449 ) ) ;
#4257=CARTESIAN_POINT ( 'NONE',  ( 0.5314960629920847390, 2.755905511811024056, 3.937007874015794773 ) ) ;
#4264=CARTESIAN_POINT ( 'NONE',  ( -2.869792031447830905, 1.067551433859863952, -0.06782095098395297950 ) ) ;
#4265=EDGE_CURVE ( 'NONE', #40586, #9070, #17368, .T. ) ;
#4271=EDGE_CURVE ( 'NONE', #27584, #5989, #60717, .T. ) ;
#4286=CARTESIAN_POINT ( 'NONE',  ( -0.5314960629921171575, 2.742784562772121681, -2.516666329989062145 ) ) ;
#4298=CARTESIAN_POINT ( 'NONE',  ( -1.701219675563209410, 1.179744462059445720, 0.3117399229855621900 ) ) ;
#4299=CARTESIAN_POINT ( 'NONE',  ( -0.5314960629921350321, 2.755905511811024056, 2.583694225513478937 ) ) ;
#4335=CARTESIAN_POINT ( 'NONE',  ( -1.313877454013331780, 0.2755905511811023723, 0.7983292792091805090 ) ) ;
#4337=CIRCLE ( 'NONE', #36587, 2.165354330708661568 ) ;
#4340=ORIENTED_EDGE ( 'NONE', *, *, #63554, .F. ) ;
#4344=CARTESIAN_POINT ( 'NONE',  ( -1.024573275495623381, 1.664102502641003678, 0.4574570760746348719 ) ) ;
#4345=DIRECTION ( 'NONE',  ( 0.000000000000000000, -1.000000000000000000, 1.408710688920637755E-15 ) ) ;
#4348=CARTESIAN_POINT ( 'NONE',  ( 0.4498537592782897998, 0.000000000000000000, -2.118110236220472675 ) ) ;
#4371=ADVANCED_FACE ( 'NONE', ( #22007, #80105 ), #73783, .T. ) ;
#4380=CARTESIAN_POINT ( 'NONE',  ( -0.4581164262379261443, 1.664773289199195538, -1.024290093949186131 ) ) ;
#4386=EDGE_CURVE ( 'NONE', #15857, #38086, #25224, .T. ) ;
#4394=CARTESIAN_POINT ( 'NONE',  ( 0.000000000000000000, 0.000000000000000000, 0.000000000000000000 ) ) ;
#4397=EDGE_CURVE ( 'NONE', #61855, #58782, #63453, .T. ) ;
#4399=EDGE_LOOP ( 'NONE', ( #74766, #18773, #7781, #26371, #1245, #28539, #69012, #59812, #71586, #59665 ) ) ;
#4418=EDGE_CURVE ( 'NONE', #39102, #22351, #4337, .T. ) ;
#4425=CARTESIAN_POINT ( 'NONE',  ( 0.6299212598425235621, 1.724409448818898127, -0.9285414500055687581 ) ) ;
#4434=AXIS2_PLACEMENT_3D ( 'NONE', #45455, #876, #27360 ) ;
#4444=VERTEX_POINT ( 'NONE', #29554 ) ;
#4452=FACE_OUTER_BOUND ( 'NONE', #4211, .T. ) ;
#4453=PLANE ( 'NONE',  #33840 ) ;
#4465=DIRECTION ( 'NONE',  ( -0.000000000000000000, 1.000000000000000000, -0.000000000000000000 ) ) ;
#4483=B_SPLINE_CURVE_WITH_KNOTS ( 'NONE', 3,
 ( #44127, #70221, #12577, #38234, #63912, #6248, #51680, #38654 ),
 .UNSPECIFIED., .F., .F.,
 ( 4, 2, 2, 4 ),
 ( 0.05229140441945555329, 0.05473522118133025000, 0.05595712956226760182, 0.05717903794320495364 ),
 .UNSPECIFIED. ) ;
#4484=EDGE_CURVE ( 'NONE', #65458, #3121, #22831, .T. ) ;
#4490=CARTESIAN_POINT ( 'NONE',  ( 3.184294706754630777, 2.755905511811024056, -0.5314960629921260393 ) ) ;
#4501=FACE_OUTER_BOUND ( 'NONE', #77542, .T. ) ;
#4517=ORIENTED_EDGE ( 'NONE', *, *, #74844, .F. ) ;
#4519=ORIENTED_EDGE ( 'NONE', *, *, #38868, .F. ) ;
#4533=ORIENTED_EDGE ( 'NONE', *, *, #25905, .F. ) ;
#4567=AXIS2_PLACEMENT_3D ( 'NONE', #22833, #22009, #68296 ) ;
#4577=DIRECTION ( 'NONE',  ( 0.000000000000000000, 1.000000000000000000, 0.000000000000000000 ) ) ;
#4594=CARTESIAN_POINT ( 'NONE',  ( -3.908320185825792326, 1.537401574803149984, 0.4744094488188970171 ) ) ;
#4600=ORIENTED_EDGE ( 'NONE', *, *, #43269, .F. ) ;
#4601=CIRCLE ( 'NONE', #44948, 3.937007874015748143 ) ;
#4606=FACE_OUTER_BOUND ( 'NONE', #8364, .T. ) ;
#4613=ORIENTED_EDGE ( 'NONE', *, *, #4271, .F. ) ;
#4628=CARTESIAN_POINT ( 'NONE',  ( 1.912049360642951330E-20, 1.062992125984252745, -2.874015748031495843 ) ) ;
#4631=ORIENTED_EDGE ( 'NONE', *, *, #45026, .F. ) ;
#4634=ORIENTED_EDGE ( 'NONE', *, *, #66088, .F. ) ;
#4664=LINE ( 'NONE', #50100, #18420 ) ;
#4667=CARTESIAN_POINT ( 'NONE',  ( -2.554262525012222174, 1.537401574803149984, 0.4744094488188970171 ) ) ;
#4670=DIRECTION ( 'NONE',  ( -1.224646799147349509E-16, 0.000000000000000000, -1.000000000000000000 ) ) ;
#4673=ADVANCED_FACE ( 'NONE', ( #68294 ), #15109, .F. ) ;
#4686=CARTESIAN_POINT ( 'NONE',  ( 0.3635331417845804602, 1.231226750417219851, -2.000933467513867470 ) ) ;
#4697=EDGE_CURVE ( 'NONE', #75845, #16450, #47346, .T. ) ;
#4702=CARTESIAN_POINT ( 'NONE',  ( -1.667080261987974543, 1.152314991887330997, 0.2771243236687696010 ) ) ;
#4705=DIRECTION ( 'NONE',  ( 1.049727191138618079E-16, -0.5150380749100549327, 0.8571673007021117785 ) ) ;
#4711=EDGE_LOOP ( 'NONE', ( #70240, #18438, #36585, #7340 ) ) ;
#4728=LINE ( 'NONE', #37953, #11362 ) ;
#4746=CARTESIAN_POINT ( 'NONE',  ( 3.911381074053594809, 1.694895442417441167, -0.4486550326265806854 ) ) ;
#4753=CARTESIAN_POINT ( 'NONE',  ( -1.031215834252966479, 1.709707895510313325, 0.4423016570855548002 ) ) ;
#4754=DIRECTION ( 'NONE',  ( 0.000000000000000000, -1.000000000000000000, -0.000000000000000000 ) ) ;
#4757=CARTESIAN_POINT ( 'NONE',  ( 3.937007874015748143, 1.724409448818897905, 0.4359958488159722534 ) ) ;
#4773=FACE_OUTER_BOUND ( 'NONE', #39205, .T. ) ;
#4780=DIRECTION ( 'NONE',  ( -0.000000000000000000, -1.000000000000000000, -0.000000000000000000 ) ) ;
#4788=CARTESIAN_POINT ( 'NONE',  ( 2.630268417803937719, 1.724409448818898127, 0.4359958488159723644 ) ) ;
#4801=CARTESIAN_POINT ( 'NONE',  ( 0.1179898944395467303, 1.077592634160696505, 1.863899027365439443 ) ) ;
#4804=ADVANCED_FACE ( 'NONE', ( #77070 ), #316, .F. ) ;
#4820=CARTESIAN_POINT ( 'NONE',  ( -0.5314960629921196000, 2.729664732663033888, -1.840814918237481113 ) ) ;
#4827=ADVANCED_FACE ( 'NONE', ( #44227 ), #70330, .T. ) ;
#4854=ORIENTED_EDGE ( 'NONE', *, *, #63459, .F. ) ;
#4855=CARTESIAN_POINT ( 'NONE',  ( 0.000000000000000000, 0.04488074079120789317, 0.000000000000000000 ) ) ;
#4856=AXIS2_PLACEMENT_3D ( 'NONE', #56095, #4345, #75067 ) ;
#4859=LINE ( 'NONE', #68024, #26333 ) ;
#4860=CARTESIAN_POINT ( 'NONE',  ( 1.141392835773559211, 0.3937007874015748254, 1.318558190104271333 ) ) ;
#4866=EDGE_CURVE ( 'NONE', #23166, #80344, #43250, .T. ) ;
#4880=VERTEX_POINT ( 'NONE', #69917 ) ;
#4897=AXIS2_PLACEMENT_3D ( 'NONE', #65315, #53901, #45919 ) ;
#4899=AXIS2_PLACEMENT_3D ( 'NONE', #46645, #47054, #52534 ) ;
#4924=CARTESIAN_POINT ( 'NONE',  ( 0.1656725442894022571, 1.091696002692744250, 2.847499275411782715 ) ) ;
#4925=CARTESIAN_POINT ( 'NONE',  ( -3.912791665790199769, 1.724409448818897905, 0.4359958488159718093 ) ) ;
#4934=B_SPLINE_CURVE_WITH_KNOTS ( 'NONE', 3,
 ( #32380, #7980, #44991, #52145 ),
 .UNSPECIFIED., .F., .F.,
 ( 4, 4 ),
 ( 0.1307222445546316614, 0.1321409493595269991 ),
 .UNSPECIFIED. ) ;
#4938=ORIENTED_EDGE ( 'NONE', *, *, #80939, .F. ) ;
#4953=AXIS2_PLACEMENT_3D ( 'NONE', #39750, #27536, #65446 ) ;
#4954=EDGE_LOOP ( 'NONE', ( #61444, #23136, #36130, #74334 ) ) ;
#4956=AXIS2_PLACEMENT_3D ( 'NONE', #30902, #44748, #12384 ) ;
#4959=CARTESIAN_POINT ( 'NONE',  ( -0.3149606299212459048, 2.559055118110236560, -3.924389226575469625 ) ) ;
#4962=CARTESIAN_POINT ( 'NONE',  ( 2.543486866223389153, 2.716535433070866645, -0.5314960629921260393 ) ) ;
#4964=CARTESIAN_POINT ( 'NONE',  ( -0.4422811034547447506, 1.709755814870675072, -3.912091310349552931 ) ) ;
#4966=CARTESIAN_POINT ( 'NONE',  ( -0.6299212598425059095, 2.165354330708661568, -3.937007874015764131 ) ) ;
#4970=EDGE_CURVE ( 'NONE', #14187, #15098, #5125, .T. ) ;
#4971=CARTESIAN_POINT ( 'NONE',  ( 3.908320185825792770, 1.506033013147133115, 0.4744094488188977388 ) ) ;
#4973=ORIENTED_EDGE ( 'NONE', *, *, #14716, .T. ) ;
#4982=CARTESIAN_POINT ( 'NONE',  ( -0.4323474733757479704, 1.341489562532706792, 3.913201052770269861 ) ) ;
#5000=CARTESIAN_POINT ( 'NONE',  ( -2.170146923806675510, 1.537401574803149984, 0.4744094488188970171 ) ) ;
#5013=VECTOR ( 'NONE', #6228, 39.37007874015748143 ) ;
#5020=CARTESIAN_POINT ( 'NONE',  ( -3.935120607642087709, 1.078895829074301593, -0.1227907875732516252 ) ) ;
#5031=CARTESIAN_POINT ( 'NONE',  ( 0.000000000000000000, 0.03937007874015747977, 0.000000000000000000 ) ) ;
#5034=DIRECTION ( 'NONE',  ( 0.000000000000000000, -0.000000000000000000, 1.000000000000000000 ) ) ;
#5038=VERTEX_POINT ( 'NONE', #75837 ) ;
#5047=CARTESIAN_POINT ( 'NONE',  ( -6.686372609646914991E-25, 1.062992125984252745, 1.850393700787401619 ) ) ;
#5050=CARTESIAN_POINT ( 'NONE',  ( 0.5314960629921294810, 2.559055118110236560, -0.9881811337016621621 ) ) ;
#5061=ADVANCED_FACE ( 'NONE', ( #82971 ), #81751, .F. ) ;
#5084=FACE_OUTER_BOUND ( 'NONE', #51511, .T. ) ;
#5085=DIMENSIONAL_EXPONENTS ( 1.000000000000000000, 0.000000000000000000, 0.000000000000000000, 0.000000000000000000, 0.000000000000000000, 0.000000000000000000, 0.000000000000000000 ) ;
#5091=CARTESIAN_POINT ( 'NONE',  ( -2.565212732165802478, 1.469708627452555261, 0.4698506773045482698 ) ) ;
#5105=CARTESIAN_POINT ( 'NONE',  ( 0.4436778669133205066, 1.368715629171030512, -1.030622242485704110 ) ) ;
#5108=DIRECTION ( 'NONE',  ( -0.000000000000000000, -1.000000000000000000, -0.000000000000000000 ) ) ;
#5113=CARTESIAN_POINT ( 'NONE',  ( -0.4256046601534574925, 1.327241662710675119, -3.913942542435401961 ) ) ;
#5125=LINE ( 'NONE', #24062, #9694 ) ;
#5129=VECTOR ( 'NONE', #11670, 39.37007874015748143 ) ;
#5154=ORIENTED_EDGE ( 'NONE', *, *, #20936, .T. ) ;
#5158=EDGE_CURVE ( 'NONE', #80251, #12202, #35238, .T. ) ;
#5167=DIRECTION ( 'NONE',  ( 0.000000000000000000, 0.000000000000000000, -1.000000000000000000 ) ) ;
#5171=EDGE_LOOP ( 'NONE', ( #79814, #50362, #35809, #23877 ) ) ;
#5174=DIRECTION ( 'NONE',  ( -1.000000000000000000, -0.000000000000000000, -0.000000000000000000 ) ) ;
#5193=CARTESIAN_POINT ( 'NONE',  ( -0.4744094488189045666, 1.537401574803149984, 2.170146923806632877 ) ) ;
#5200=CARTESIAN_POINT ( 'NONE',  ( 0.000000000000000000, 2.165354330708661568, 0.000000000000000000 ) ) ;
#5208=CARTESIAN_POINT ( 'NONE',  ( 1.115258233734506055, 1.079260963165236342, 0.1241637467760029201 ) ) ;
#5211=CARTESIAN_POINT ( 'NONE',  ( 0.4744094488188841385, 1.506018186285911442, 3.908320185825793658 ) ) ;
#5229=CARTESIAN_POINT ( 'NONE',  ( 0.000000000000000000, 0.07874015748031502893, 0.000000000000000000 ) ) ;
#5237=CARTESIAN_POINT ( 'NONE',  ( -0.4024773509250166303, 1.285781980195177532, 1.047418557759479008 ) ) ;
#5266=ORIENTED_EDGE ( 'NONE', *, *, #64961, .F. ) ;
#5273=CARTESIAN_POINT ( 'NONE',  ( 3.264097702071373064, 2.755905511811024056, -0.5314960629921260393 ) ) ;
#5284=ORIENTED_EDGE ( 'NONE', *, *, #20936, .F. ) ;
#5287=PLANE ( 'NONE',  #33955 ) ;
#5296=DIRECTION ( 'NONE',  ( 0.000000000000000000, 1.000000000000000000, -0.000000000000000000 ) ) ;
#5298=CONICAL_SURFACE ( 'NONE', #34865, 0.1190944881889763746, 0.8726646259971682085 ) ;
#5299=CARTESIAN_POINT ( 'NONE',  ( -0.5314960629921371416, 2.755905511811024056, 3.184294706754628557 ) ) ;
#5310=EDGE_CURVE ( 'NONE', #63414, #42276, #8047, .T. ) ;
#5330=CYLINDRICAL_SURFACE ( 'NONE', #2210, 0.1771653543307085410 ) ;
#5335=CARTESIAN_POINT ( 'NONE',  ( 0.2422408962274362754, 1.129482473309794788, -1.586876790830786588 ) ) ;
#5349=ORIENTED_EDGE ( 'NONE', *, *, #50488, .F. ) ;
#5361=VERTEX_POINT ( 'NONE', #32445 ) ;
#5363=ORIENTED_EDGE ( 'NONE', *, *, #18680, .T. ) ;
#5370=DIRECTION ( 'NONE',  ( -0.000000000000000000, -1.000000000000000000, -0.000000000000000000 ) ) ;
#5382=ORIENTED_EDGE ( 'NONE', *, *, #53323, .T. ) ;
#5388=CARTESIAN_POINT ( 'NONE',  ( -0.1528522289550877378, 1.087215528301579193, 3.934144666135135360 ) ) ;
#5407=CARTESIAN_POINT ( 'NONE',  ( 0.5314960629920991719, 2.729656616209943376, 2.556891461833393553 ) ) ;
#5413=MECHANICAL_DESIGN_GEOMETRIC_PRESENTATION_REPRESENTATION('',(#56467),#14986);
#5426=CARTESIAN_POINT ( 'NONE',  ( 1.150409065943327258, 0.000000000000000000, 0.8265612839971842041 ) ) ;
#5428=ADVANCED_FACE ( 'NONE', ( #34125 ), #17812, .F. ) ;
#5431=CARTESIAN_POINT ( 'NONE',  ( 0.000000000000000000, 1.929133858267716661, 2.362204724409448620 ) ) ;
#5432=VERTEX_POINT ( 'NONE', #52633 ) ;
#5433=EDGE_CURVE ( 'NONE', #40470, #7361, #16503, .T. ) ;
#5434=DIRECTION ( 'NONE',  ( 1.000000000000000000, 0.000000000000000000, 3.455050906509825972E-15 ) ) ;
#5439=DIRECTION ( 'NONE',  ( 0.000000000000000000, -1.000000000000000000, 0.000000000000000000 ) ) ;
#5448=ORIENTED_EDGE ( 'NONE', *, *, #50835, .F. ) ;
#5461=ORIENTED_EDGE ( 'NONE', *, *, #20213, .F. ) ;
#5463=ORIENTED_EDGE ( 'NONE', *, *, #40392, .T. ) ;
#5465=CARTESIAN_POINT ( 'NONE',  ( 2.857004350179362273, 1.081388112195868390, -0.1351566381870096811 ) ) ;
#5477=AXIS2_PLACEMENT_3D ( 'NONE', #24719, #17608, #62623 ) ;
#5495=CARTESIAN_POINT ( 'NONE',  ( 0.4702623840880357786, 1.602034772339061552, -1.018747574612956619 ) ) ;
#5518=LINE ( 'NONE', #6759, #49471 ) ;
#5549=AXIS2_PLACEMENT_3D ( 'NONE', #58593, #52269, #962 ) ;
#5558=DIRECTION ( 'NONE',  ( 0.000000000000000000, 1.000000000000000000, 0.000000000000000000 ) ) ;
#5559=ORIENTED_EDGE ( 'NONE', *, *, #30484, .F. ) ;
#5574=DIRECTION ( 'NONE',  ( 0.000000000000000000, 0.000000000000000000, 1.000000000000000000 ) ) ;
#5600=CARTESIAN_POINT ( 'NONE',  ( 3.937007874015748143, 2.755905511811024056, -0.5314960629921260393 ) ) ;
#5614=EDGE_CURVE ( 'NONE', #25547, #69342, #35597, .T. ) ;
#5615=CARTESIAN_POINT ( 'NONE',  ( 1.116867003146159609, 1.075369016579923676, 0.1087923042922196853 ) ) ;
#5632=ORIENTED_EDGE ( 'NONE', *, *, #56851, .T. ) ;
#5644=CARTESIAN_POINT ( 'NONE',  ( -0.2386152867011636369, 1.127078383925389504, 1.096469326408681999 ) ) ;
#5662=CARTESIAN_POINT ( 'NONE',  ( -0.5314960629921348101, 2.729661060880496759, 2.530077729939674835 ) ) ;
#5673=VERTEX_POINT ( 'NONE', #9926 ) ;
#5678=CARTESIAN_POINT ( 'NONE',  ( 0.000000000000000000, 0.4374015748031496176, 0.000000000000000000 ) ) ;
#5688=CARTESIAN_POINT ( 'NONE',  ( 1.912049360642951330E-20, 1.062992125984252745, -2.874015748031495843 ) ) ;
#5705=AXIS2_PLACEMENT_3D ( 'NONE', #56863, #24473, #63605 ) ;
#5718=FACE_OUTER_BOUND ( 'NONE', #76006, .T. ) ;
#5722=ORIENTED_EDGE ( 'NONE', *, *, #11555, .F. ) ;
#5735=CARTESIAN_POINT ( 'NONE',  ( 0.2639696576368102954, 1.142922413699645645, 2.800935327256448559 ) ) ;
#5750=ORIENTED_EDGE ( 'NONE', *, *, #47538, .T. ) ;
#5752=CIRCLE ( 'NONE', #66284, 3.937007874015748143 ) ;
#5765=ORIENTED_EDGE ( 'NONE', *, *, #70822, .F. ) ;
#5767=ORIENTED_EDGE ( 'NONE', *, *, #27454, .T. ) ;
#5777=PLANE ( 'NONE',  #79402 ) ;
#5786=ORIENTED_EDGE ( 'NONE', *, *, #51527, .T. ) ;
#5806=AXIS2_PLACEMENT_3D ( 'NONE', #82537, #44206, #38321 ) ;
#5821=CARTESIAN_POINT ( 'NONE',  ( 0.5314960629921349211, 2.716535433070866645, -2.543486866223387377 ) ) ;
#5830=FACE_OUTER_BOUND ( 'NONE', #54401, .T. ) ;
#5836=ORIENTED_EDGE ( 'NONE', *, *, #82874, .F. ) ;
#5837=LINE ( 'NONE', #64334, #33788 ) ;
#5845=DIRECTION ( 'NONE',  ( 0.000000000000000000, 0.000000000000000000, -1.000000000000000000 ) ) ;
#5862=CARTESIAN_POINT ( 'NONE',  ( 0.4117837489889513702, 1.301386200251873682, -2.666378553117691563 ) ) ;
#5865=ORIENTED_EDGE ( 'NONE', *, *, #47465, .F. ) ;
#5872=ADVANCED_FACE ( 'NONE', ( #78018 ), #39702, .F. ) ;
#5874=VECTOR ( 'NONE', #57715, 39.37007874015748143 ) ;
#5896=EDGE_CURVE ( 'NONE', #82375, #62933, #50042, .T. ) ;
#5902=CARTESIAN_POINT ( 'NONE',  ( -2.630268417803964809, 1.724409448818898127, -0.4359958488159723089 ) ) ;
#5905=CARTESIAN_POINT ( 'NONE',  ( -2.723203318070452017, 1.231544801320239024, 0.3638227417423900434 ) ) ;
#5917=CARTESIAN_POINT ( 'NONE',  ( 0.3564806704966359541, 1.223997042866947993, -1.063963581927926283 ) ) ;
#5922=CARTESIAN_POINT ( 'NONE',  ( 0.3336463653988042677, 1.199832043049261721, -1.973860402524058255 ) ) ;
#5927=CARTESIAN_POINT ( 'NONE',  ( -0.3133043865842751186, 1.179792816808425737, -3.924584650684677101 ) ) ;
#5943=DIRECTION ( 'NONE',  ( 0.000000000000000000, 1.000000000000000000, 0.000000000000000000 ) ) ;
#5958=DIRECTION ( 'NONE',  ( 0.000000000000000000, 1.000000000000000000, 0.000000000000000000 ) ) ;
#5968=CARTESIAN_POINT ( 'NONE',  ( -0.5314960629921325896, 2.729653112494254685, 1.868118600343975588 ) ) ;
#5972=ORIENTED_EDGE ( 'NONE', *, *, #23961, .T. ) ;
#5981=( GEOMETRIC_REPRESENTATION_CONTEXT ( 3 ) GLOBAL_UNCERTAINTY_ASSIGNED_CONTEXT ( ( #3247 ) ) GLOBAL_UNIT_ASSIGNED_CONTEXT ( ( #79023, #60050, #39867 ) ) REPRESENTATION_CONTEXT ( 'NONE', 'WORKASPACE' ) );
#5985=DIRECTION ( 'NONE',  ( -0.000000000000000000, -1.000000000000000000, -0.000000000000000000 ) ) ;
#5989=VERTEX_POINT ( 'NONE', #7299 ) ;
#5997=EDGE_CURVE ( 'NONE', #76797, #34953, #68869, .T. ) ;
#6014=CARTESIAN_POINT ( 'NONE',  ( -0.06791843738634079086, 1.067571514150118084, 1.854636000526581840 ) ) ;
#6019=FACE_OUTER_BOUND ( 'NONE', #57602, .T. ) ;
#6026=B_SPLINE_CURVE_WITH_KNOTS ( 'NONE', 3,
 ( #57440, #70078, #25868, #12431 ),
 .UNSPECIFIED., .F., .F.,
 ( 4, 4 ),
 ( 0.0005422360305776403313, 0.001226984380451624388 ),
 .UNSPECIFIED. ) ;
#6028=CARTESIAN_POINT ( 'NONE',  ( 2.586063147568535836, 1.653225543546883891, 0.4603267246303527904 ) ) ;
#6058=CARTESIAN_POINT ( 'NONE',  ( 3.908721163486909234, 1.601505345183718676, 0.4711385086307711689 ) ) ;
#6084=ORIENTED_EDGE ( 'NONE', *, *, #80096, .F. ) ;
#6086=ORIENTED_EDGE ( 'NONE', *, *, #79452, .T. ) ;
#6087=CARTESIAN_POINT ( 'NONE',  ( 0.4177787735906999811, 1.312623414240995157, -1.714017618091133288 ) ) ;
#6092=CARTESIAN_POINT ( 'NONE',  ( 0.000000000000000000, 2.755905511811024056, 0.000000000000000000 ) ) ;
#6112=CARTESIAN_POINT ( 'NONE',  ( 1.348312163386739426, 0.2755905511811023723, 0.7386866130305692613 ) ) ;
#6132=DIRECTION ( 'NONE',  ( 0.000000000000000000, -1.000000000000000000, 0.000000000000000000 ) ) ;
#6136=ORIENTED_EDGE ( 'NONE', *, *, #67416, .T. ) ;
#6151=CARTESIAN_POINT ( 'NONE',  ( 0.4255991402441264837, 1.325803004855074407, 2.647315919250823768 ) ) ;
#6164=ORIENTED_EDGE ( 'NONE', *, *, #35750, .T. ) ;
#6175=EDGE_CURVE ( 'NONE', #34953, #76797, #13784, .T. ) ;
#6178=ORIENTED_EDGE ( 'NONE', *, *, #57803, .T. ) ;
#6196=ORIENTED_EDGE ( 'NONE', *, *, #40336, .F. ) ;
#6204=DIRECTION ( 'NONE',  ( 0.000000000000000000, 0.000000000000000000, 1.000000000000000000 ) ) ;
#6206=VECTOR ( 'NONE', #59638, 39.37007874015748143 ) ;
#6210=CIRCLE ( 'NONE', #35856, 0.5118110236220471121 ) ;
#6225=AXIS2_PLACEMENT_3D ( 'NONE', #17119, #4465, #30548 ) ;
#6228=DIRECTION ( 'NONE',  ( 1.000000000000000000, -0.000000000000000000, -0.000000000000000000 ) ) ;
#6243=CARTESIAN_POINT ( 'NONE',  ( -3.936548249448418080, 1.066819220836087379, -0.06211919455352141878 ) ) ;
#6248=CARTESIAN_POINT ( 'NONE',  ( -0.4735970878719478194, 1.569539909699054325, 1.017201612406801070 ) ) ;
#6250=ORIENTED_EDGE ( 'NONE', *, *, #56357, .F. ) ;
#6251=CYLINDRICAL_SURFACE ( 'NONE', #29748, 0.4744094488188972947 ) ;
#6259=LINE ( 'NONE', #83288, #50328 ) ;
#6260=AXIS2_PLACEMENT_3D ( 'NONE', #33780, #45971, #52701 ) ;
#6265=VERTEX_POINT ( 'NONE', #36285 ) ;
#6284=ORIENTED_EDGE ( 'NONE', *, *, #53723, .F. ) ;
#6287=CARTESIAN_POINT ( 'NONE',  ( 2.847313777101087240, 1.091897865355356601, -0.1662078246829617190 ) ) ;
#6314=CARTESIAN_POINT ( 'NONE',  ( -2.554262525012342966, 1.554943921348592273, -0.4744094488188976277 ) ) ;
#6316=EDGE_CURVE ( 'NONE', #27965, #69251, #40309, .T. ) ;
#6327=VECTOR ( 'NONE', #46784, 39.37007874015748143 ) ;
#6328=VECTOR ( 'NONE', #58066, 39.37007874015748143 ) ;
#6347=CARTESIAN_POINT ( 'NONE',  ( -0.1528381195902957790, 1.087211650537911245, -3.934145130003242397 ) ) ;
#6368=VERTEX_POINT ( 'NONE', #35462 ) ;
#6384=CARTESIAN_POINT ( 'NONE',  ( 0.5314960629921294810, 2.755905511811024056, -0.9881811337016621621 ) ) ;
#6385=CARTESIAN_POINT ( 'NONE',  ( -0.5314960629921325896, 2.742776589945747467, 1.881759001202176318 ) ) ;
#6386=VERTEX_POINT ( 'NONE', #11032 ) ;
#6391=EDGE_CURVE ( 'NONE', #80751, #26586, #62364, .T. ) ;
#6404=CARTESIAN_POINT ( 'NONE',  ( 3.934067344273005418, 1.088024857645069288, -0.1528641246056967884 ) ) ;
#6405=ORIENTED_EDGE ( 'NONE', *, *, #83038, .F. ) ;
#6414=B_SPLINE_CURVE_WITH_KNOTS ( 'NONE', 3,
 ( #60719, #61961, #73363, #22426, #23241, #54816, #73785, #2660, #3897, #42595, #16539, #53980 ),
 .UNSPECIFIED., .F., .F.,
 ( 4, 2, 2, 2, 2, 4 ),
 ( 0.05454303362711762637, 0.05585633982237121070, 0.05651299291999801327, 0.05716964601762482279, 0.05848295221287842793, 0.05979625840813203308 ),
 .UNSPECIFIED. ) ;
#6432=CARTESIAN_POINT ( 'NONE',  ( -0.4255991402441413052, 1.325803004855072187, 2.077093529568096120 ) ) ;
#6437=DIRECTION ( 'NONE',  ( 0.000000000000000000, 0.000000000000000000, -1.000000000000000000 ) ) ;
#6445=CARTESIAN_POINT ( 'NONE',  ( 1.022505811683676713, 1.428663316172101627, 0.4620424953995453943 ) ) ;
#6475=DIRECTION ( 'NONE',  ( 0.000000000000000000, -1.000000000000000000, 0.000000000000000000 ) ) ;
#6477=EDGE_CURVE ( 'NONE', #8202, #1055, #56763, .T. ) ;
#6503=ORIENTED_EDGE ( 'NONE', *, *, #83098, .F. ) ;
#6506=B_SPLINE_CURVE_WITH_KNOTS ( 'NONE', 3,
 ( #5193, #57762, #37997, #38415, #19057, #82225, #18246, #37586, #64096, #56523, #25363, #6432, #70834, #64511, #18651, #13182, #38832, #11521, #75907, #51026, #76725, #57344, #31267, #6848, #26202, #25779, #6014, #82629, #69170, #24943 ),
 .UNSPECIFIED., .F., .F.,
 ( 4, 2, 2, 2, 2, 2, 2, 2, 2, 2, 2, 2, 2, 2, 4 ),
 ( 0.01323639539072392693, 0.01388240907739107452, 0.01452842276405822385, 0.01582045013739251382, 0.01711247751072680900, 0.01840450488406109725, 0.02098855963072968414, 0.02357261437739826757, 0.02486464175073256622, 0.02615666912406686487, 0.02744869649740116352, 0.02874072387073546564, 0.03132477861740406294, 0.03261680599073836506, 0.03390883336407266024 ),
 .UNSPECIFIED. ) ;
#6520=EDGE_LOOP ( 'NONE', ( #40258, #20988, #10021, #31875 ) ) ;
#6555=ORIENTED_EDGE ( 'NONE', *, *, #31362, .F. ) ;
#6570=LINE ( 'NONE', #32241, #39923 ) ;
#6596=ORIENTED_EDGE ( 'NONE', *, *, #26135, .F. ) ;
#6605=CIRCLE ( 'NONE', #56351, 1.122047244094488194 ) ;
#6615=ORIENTED_EDGE ( 'NONE', *, *, #78384, .T. ) ;
#6622=CARTESIAN_POINT ( 'NONE',  ( -0.4591639709769206878, 1.414133617986971458, 3.910145371492633970 ) ) ;
#6646=CARTESIAN_POINT ( 'NONE',  ( -1.559171609364246924, 0.3937007874015747699, 0.6156134192599649335 ) ) ;
#6668=EDGE_CURVE ( 'NONE', #20489, #78980, #42000, .T. ) ;
#6671=DIRECTION ( 'NONE',  ( -3.491481338843133355E-15, -0.000000000000000000, 1.000000000000000000 ) ) ;
#6676=CARTESIAN_POINT ( 'NONE',  ( 0.000000000000000000, 2.755905511811024056, 0.000000000000000000 ) ) ;
#6701=ORIENTED_EDGE ( 'NONE', *, *, #38498, .F. ) ;
#6705=CARTESIAN_POINT ( 'NONE',  ( 2.554854094587847513, 1.520093187801265566, -0.4741711390158123707 ) ) ;
#6733=CARTESIAN_POINT ( 'NONE',  ( -2.170146923806675510, 1.537401574803149984, 0.4744094488188970171 ) ) ;
#6736=CARTESIAN_POINT ( 'NONE',  ( 1.348312163386739426, 0.2755905511811023723, 0.5221511799597032821 ) ) ;
#6750=FACE_OUTER_BOUND ( 'NONE', #24618, .T. ) ;
#6759=CARTESIAN_POINT ( 'NONE',  ( -0.03443470937339728616, 0.2755905511811023723, -1.635441089090149402 ) ) ;
#6772=CARTESIAN_POINT ( 'NONE',  ( 0.4697362858027160915, 1.605934398054998935, -2.158929595217815578 ) ) ;
#6791=EDGE_CURVE ( 'NONE', #65941, #26273, #32031, .T. ) ;
#6793=AXIS2_PLACEMENT_3D ( 'NONE', #76903, #75265, #18017 ) ;
#6800=CARTESIAN_POINT ( 'NONE',  ( -0.3635064842674102237, 1.231191414405744977, -2.000903845782021850 ) ) ;
#6804=ORIENTED_EDGE ( 'NONE', *, *, #19351, .F. ) ;
#6815=VECTOR ( 'NONE', #51789, 39.37007874015748143 ) ;
#6848=CARTESIAN_POINT ( 'NONE',  ( -0.1656725442894096123, 1.091696002692741141, 1.876910173407116966 ) ) ;
#6852=CARTESIAN_POINT ( 'NONE',  ( -0.4469586986359131431, 1.697151583350148263, 2.112655059233961907 ) ) ;
#6860=CARTESIAN_POINT ( 'NONE',  ( 1.096606552046649030, 1.126456178498281613, -0.2390280536361044927 ) ) ;
#6863=DIRECTION ( 'NONE',  ( 0.000000000000000000, 1.000000000000000000, 0.000000000000000000 ) ) ;
#6880=DIRECTION ( 'NONE',  ( -0.000000000000000000, 1.000000000000000000, -0.000000000000000000 ) ) ;
#6913=AXIS2_PLACEMENT_3D ( 'NONE', #43870, #69569, #31251 ) ;
#6918=ORIENTED_EDGE ( 'NONE', *, *, #26633, .F. ) ;
#6920=VERTEX_POINT ( 'NONE', #69916 ) ;
#6933=VERTEX_POINT ( 'NONE', #57272 ) ;
#6934=CARTESIAN_POINT ( 'NONE',  ( -1.121710378714982248, 1.063787285278161798, -0.03163150153590546521 ) ) ;
#6941=EDGE_LOOP ( 'NONE', ( #43411, #49100, #7440, #82792 ) ) ;
#6942=DIRECTION ( 'NONE',  ( 0.000000000000000000, 0.000000000000000000, 1.000000000000000000 ) ) ;
#6944=EDGE_CURVE ( 'NONE', #44534, #71433, #82970, .T. ) ;
#6951=EDGE_CURVE ( 'NONE', #30815, #19015, #26558, .T. ) ;
#6971=AXIS2_PLACEMENT_3D ( 'NONE', #37107, #43811, #24474 ) ;
#6973=EDGE_CURVE ( 'NONE', #11714, #13837, #49389, .T. ) ;
#6986=EDGE_CURVE ( 'NONE', #30609, #61385, #59369, .T. ) ;
#6988=CARTESIAN_POINT ( 'NONE',  ( 0.4359958488159444423, 1.724409448818900570, 2.630268417803970138 ) ) ;
#6995=EDGE_CURVE ( 'NONE', #68098, #24318, #52632, .T. ) ;
#7002=VERTEX_POINT ( 'NONE', #472 ) ;
#7016=ORIENTED_EDGE ( 'NONE', *, *, #48672, .F. ) ;
#7018=ORIENTED_EDGE ( 'NONE', *, *, #79927, .T. ) ;
#7029=DIRECTION ( 'NONE',  ( -0.000000000000000000, -1.000000000000000000, -0.000000000000000000 ) ) ;
#7036=VERTEX_POINT ( 'NONE', #7195 ) ;
#7044=CARTESIAN_POINT ( 'NONE',  ( 0.000000000000000000, 2.755905511811024056, 0.000000000000000000 ) ) ;
#7088=CARTESIAN_POINT ( 'NONE',  ( 0.4177787735907000366, 1.299212598425196985, -1.382006255033530806 ) ) ;
#7091=ORIENTED_EDGE ( 'NONE', *, *, #28945, .T. ) ;
#7097=LINE ( 'NONE', #7525, #63291 ) ;
#7100=CARTESIAN_POINT ( 'NONE',  ( 0.1818635362617186391, 1.098419255088208812, -3.932883114322541118 ) ) ;
#7104=ORIENTED_EDGE ( 'NONE', *, *, #16133, .F. ) ;
#7122=VERTEX_POINT ( 'NONE', #58535 ) ;
#7124=CARTESIAN_POINT ( 'NONE',  ( 2.585397804484631745, 1.422882880004780581, -0.4606469518571244537 ) ) ;
#7150=EDGE_CURVE ( 'NONE', #49578, #9799, #39601, .T. ) ;
#7158=CARTESIAN_POINT ( 'NONE',  ( -2.554859668665151240, 1.520054044952884098, -0.4741688556381182251 ) ) ;
#7165=DIRECTION ( 'NONE',  ( 1.047444401652940007E-14, -0.000000000000000000, -1.000000000000000000 ) ) ;
#7188=ORIENTED_EDGE ( 'NONE', *, *, #6175, .F. ) ;
#7195=CARTESIAN_POINT ( 'NONE',  ( 0.5314960629921372526, 2.716535433070866645, -3.224202737261813834 ) ) ;
#7200=CARTESIAN_POINT ( 'NONE',  ( 0.000000000000000000, 2.165354330708661568, 0.000000000000000000 ) ) ;
#7205=VERTEX_POINT ( 'NONE', #13944 ) ;
#7223=CARTESIAN_POINT ( 'NONE',  ( -0.3811282389481102650, 1.253478596003495094, -2.019714574425724773 ) ) ;
#7224=ORIENTED_EDGE ( 'NONE', *, *, #62746, .F. ) ;
#7243=EDGE_LOOP ( 'NONE', ( #13850, #31758, #70154, #14288 ) ) ;
#7256=VECTOR ( 'NONE', #23687, 39.37007874015748143 ) ;
#7270=DIRECTION ( 'NONE',  ( -3.491481338843132961E-15, 0.000000000000000000, 1.000000000000000000 ) ) ;
#7273=AXIS2_PLACEMENT_3D ( 'NONE', #67879, #55219, #80926 ) ;
#7275=CARTESIAN_POINT ( 'NONE',  ( -0.4741686481756466343, 1.554815631980117185, 2.169549097624130951 ) ) ;
#7298=SHAPE_REPRESENTATION ( 'Cast Iron Heavy Chuck Body', ( #22098 ), #5981 ) ;
#7299=CARTESIAN_POINT ( 'NONE',  ( 0.9881811337016640495, 2.559055118110236560, 0.5314960629921260393 ) ) ;
#7310=AXIS2_PLACEMENT_3D ( 'NONE', #58276, #26719, #70497 ) ;
#7320=FACE_OUTER_BOUND ( 'NONE', #72274, .T. ) ;
#7326=AXIS2_PLACEMENT_3D ( 'NONE', #42206, #54000, #22028 ) ;
#7340=ORIENTED_EDGE ( 'NONE', *, *, #10682, .F. ) ;
#7352=ORIENTED_EDGE ( 'NONE', *, *, #40191, .F. ) ;
#7354=CARTESIAN_POINT ( 'NONE',  ( -1.057085711732377087, 1.247373137590361836, -0.3766906164242062038 ) ) ;
#7357=CARTESIAN_POINT ( 'NONE',  ( 3.937007874015748143, 1.724409448818897905, 0.4359958488159722534 ) ) ;
#7361=VERTEX_POINT ( 'NONE', #20668 ) ;
#7362=DIRECTION ( 'NONE',  ( -0.000000000000000000, -1.000000000000000000, -0.000000000000000000 ) ) ;
#7363=LINE ( 'NONE', #52374, #66737 ) ;
#7396=ORIENTED_EDGE ( 'NONE', *, *, #37360, .T. ) ;
#7406=EDGE_CURVE ( 'NONE', #19993, #64046, #31183, .T. ) ;
#7412=CARTESIAN_POINT ( 'NONE',  ( 1.033875059083676717, 1.724409448818897905, 0.4359958488159722534 ) ) ;
#7431=DIRECTION ( 'NONE',  ( 0.000000000000000000, 0.000000000000000000, -1.000000000000000000 ) ) ;
#7440=ORIENTED_EDGE ( 'NONE', *, *, #45360, .F. ) ;
#7444=VECTOR ( 'NONE', #36869, 39.37007874015748143 ) ;
#7454=DIRECTION ( 'NONE',  ( 0.000000000000000000, 0.000000000000000000, -1.000000000000000000 ) ) ;
#7460=ORIENTED_EDGE ( 'NONE', *, *, #27456, .F. ) ;
#7468=ADVANCED_FACE ( 'NONE', ( #14370 ), #65715, .F. ) ;
#7471=CARTESIAN_POINT ( 'NONE',  ( 1.403614904275686858E-14, 1.537401574803149984, -3.937007874015761910 ) ) ;
#7487=PRODUCT_DEFINITION_CONTEXT ( 'detailed design', #15402, 'design' ) ;
#7492=EDGE_CURVE ( 'NONE', #21709, #29467, #60600, .T. ) ;
#7495=CARTESIAN_POINT ( 'NONE',  ( 1.348312163386739426, 1.062992125984252079, 0.7386866130305692613 ) ) ;
#7510=VECTOR ( 'NONE', #60353, 39.37007874015748143 ) ;
#7515=CARTESIAN_POINT ( 'NONE',  ( -2.170146923806554273, 1.537401574803149984, -0.4744094488188975722 ) ) ;
#7525=CARTESIAN_POINT ( 'NONE',  ( 0.6299212598425100174, 0.000000000000000000, 0.9285414500055778619 ) ) ;
#7528=CARTESIAN_POINT ( 'NONE',  ( 0.4262761708485561241, 1.326877055403132388, -3.913880873785005488 ) ) ;
#7529=CYLINDRICAL_SURFACE ( 'NONE', #4899, 0.4744094488188972947 ) ;
#7531=EDGE_CURVE ( 'NONE', #82661, #79084, #3796, .T. ) ;
#7535=ORIENTED_EDGE ( 'NONE', *, *, #66936, .T. ) ;
#7550=AXIS2_PLACEMENT_3D ( 'NONE', #1994, #7901, #34816 ) ;
#7553=VECTOR ( 'NONE', #36566, 39.37007874015748143 ) ;
#7555=CARTESIAN_POINT ( 'NONE',  ( 2.822823420596364929, 1.118719813955008524, 0.2236424093447139938 ) ) ;
#7562=CARTESIAN_POINT ( 'NONE',  ( 0.4359958488159797474, 1.724409448818897905, -2.094141031014984833 ) ) ;
#7608=CONICAL_SURFACE ( 'NONE', #58717, 1.968503937007874072, 0.7853981633974500554 ) ;
#7611=AXIS2_PLACEMENT_3D ( 'NONE', #53753, #2017, #16316 ) ;
#7613=CIRCLE ( 'NONE', #61371, 0.5118110236220471121 ) ;
#7615=CARTESIAN_POINT ( 'NONE',  ( 1.141392835773559211, 0.3937007874015747699, 1.141392835773562764 ) ) ;
#7620=CARTESIAN_POINT ( 'NONE',  ( 1.854472803289052507, 2.716535433070866645, 0.5314960629921260393 ) ) ;
#7639=ORIENTED_EDGE ( 'NONE', *, *, #55316, .T. ) ;
#7642=ORIENTED_EDGE ( 'NONE', *, *, #21253, .F. ) ;
#7648=DIRECTION ( 'NONE',  ( 0.000000000000000000, 0.000000000000000000, -1.000000000000000000 ) ) ;
#7656=DIRECTION ( 'NONE',  ( 0.000000000000000000, 0.000000000000000000, -1.000000000000000000 ) ) ;
#7657=EDGE_LOOP ( 'NONE', ( #44643, #65213, #39862, #19626 ) ) ;
#7660=ORIENTED_EDGE ( 'NONE', *, *, #71659, .F. ) ;
#7678=AXIS2_PLACEMENT_3D ( 'NONE', #81376, #29594, #35088 ) ;
#7683=CARTESIAN_POINT ( 'NONE',  ( 2.142213561789876319, 0.02617651024168224372, -0.4623158380715471361 ) ) ;
#7688=DIRECTION ( 'NONE',  ( -0.000000000000000000, -1.000000000000000000, -0.000000000000000000 ) ) ;
#7703=CARTESIAN_POINT ( 'NONE',  ( 1.348312163386739426, 0.2755905511811023723, 0.7386866130305692613 ) ) ;
#7706=CARTESIAN_POINT ( 'NONE',  ( -0.4744094488189045666, 1.537401574803149984, 2.170146923806632877 ) ) ;
#7712=FACE_OUTER_BOUND ( 'NONE', #35981, .T. ) ;
#7731=CIRCLE ( 'NONE', #65534, 1.122047244094488194 ) ;
#7735=VECTOR ( 'NONE', #74110, 39.37007874015748143 ) ;
#7741=EDGE_CURVE ( 'NONE', #36894, #26552, #70016, .T. ) ;
#7751=CARTESIAN_POINT ( 'NONE',  ( 0.4744094488188940750, 1.506013545763978945, 1.016821367227985551 ) ) ;
#7771=ORIENTED_EDGE ( 'NONE', *, *, #49802, .T. ) ;
#7772=CYLINDRICAL_SURFACE ( 'NONE', #43520, 0.09842519685039351207 ) ;
#7775=CARTESIAN_POINT ( 'NONE',  ( -0.4567729623170651010, 1.408376684009858826, 2.593294524635601395 ) ) ;
#7781=ORIENTED_EDGE ( 'NONE', *, *, #37866, .F. ) ;
#7783=CARTESIAN_POINT ( 'NONE',  ( -1.022510163891046098, 1.428599907254325618, -0.4620330969692038603 ) ) ;
#7786=CARTESIAN_POINT ( 'NONE',  ( 0.000000000000000000, 0.000000000000000000, -2.362204724409448620 ) ) ;
#7791=ORIENTED_EDGE ( 'NONE', *, *, #42337, .T. ) ;
#7798=EDGE_CURVE ( 'NONE', #74653, #57006, #16281, .T. ) ;
#7836=CARTESIAN_POINT ( 'NONE',  ( 1.016821367227983774, 1.553651517367183654, 0.4744094488188976277 ) ) ;
#7849=ORIENTED_EDGE ( 'NONE', *, *, #37212, .T. ) ;
#7858=EDGE_CURVE ( 'NONE', #28229, #61385, #152, .T. ) ;
#7861=ADVANCED_FACE ( 'NONE', ( #49220 ), #47568, .F. ) ;
#7875=CARTESIAN_POINT ( 'NONE',  ( -1.313877454013332224, 1.122131950691689140, 0.7983292792091805090 ) ) ;
#7876=CARTESIAN_POINT ( 'NONE',  ( -2.503252890251015828, 2.755905511811024056, -0.5314960629921260393 ) ) ;
#7878=DIRECTION ( 'NONE',  ( 1.047444401652940007E-14, -0.000000000000000000, -1.000000000000000000 ) ) ;
#7884=ORIENTED_EDGE ( 'NONE', *, *, #48595, .F. ) ;
#7888=EDGE_CURVE ( 'NONE', #13837, #1571, #55231, .T. ) ;
#7892=DIRECTION ( 'NONE',  ( -0.000000000000000000, -1.000000000000000000, -0.000000000000000000 ) ) ;
#7893=ADVANCED_FACE ( 'NONE', ( #73686 ), #47193, .T. ) ;
#7901=DIRECTION ( 'NONE',  ( -0.000000000000000000, -1.000000000000000000, -0.000000000000000000 ) ) ;
#7916=CARTESIAN_POINT ( 'NONE',  ( -0.4678516549211644837, 1.617630162216313172, -1.019861537960136566 ) ) ;
#7918=CARTESIAN_POINT ( 'NONE',  ( 0.000000000000000000, 0.000000000000000000, 0.000000000000000000 ) ) ;
#7940=DIRECTION ( 'NONE',  ( -0.000000000000000000, -1.000000000000000000, -0.000000000000000000 ) ) ;
#7955=EDGE_LOOP ( 'NONE', ( #82606, #18516, #31125, #82166 ) ) ;
#7968=ORIENTED_EDGE ( 'NONE', *, *, #9731, .T. ) ;
#7973=CARTESIAN_POINT ( 'NONE',  ( 2.808613111760720926, 1.134406187872319505, 0.2508088161067695276 ) ) ;
#7980=CARTESIAN_POINT ( 'NONE',  ( 0.5314960629921348101, 2.742784437388869900, -2.516666458167339471 ) ) ;
#8016=EDGE_CURVE ( 'NONE', #11783, #12200, #28217, .T. ) ;
#8032=DIRECTION ( 'NONE',  ( -0.000000000000000000, -1.000000000000000000, -0.000000000000000000 ) ) ;
#8043=ADVANCED_FACE ( 'NONE', ( #75741 ), #31100, .F. ) ;
#8047=LINE ( 'NONE', #72433, #37908 ) ;
#8054=ORIENTED_EDGE ( 'NONE', *, *, #7798, .T. ) ;
#8064=CARTESIAN_POINT ( 'NONE',  ( 0.04057826866093373203, 1.064724180150604216, -1.477648957518036710 ) ) ;
#8072=CARTESIAN_POINT ( 'NONE',  ( -0.4734688692632945672, 1.503144958756605698, -2.167784222423876805 ) ) ;
#8073=ORIENTED_EDGE ( 'NONE', *, *, #52442, .T. ) ;
#8088=CARTESIAN_POINT ( 'NONE',  ( -0.5314960629921395840, 2.716830163678111365, 3.890345922373657839 ) ) ;
#8114=DIRECTION ( 'NONE',  ( 0.000000000000000000, 1.000000000000000000, 0.000000000000000000 ) ) ;
#8117=ADVANCED_FACE ( 'NONE', ( #24782 ), #42899, .F. ) ;
#8126=CARTESIAN_POINT ( 'NONE',  ( -3.937007874015748143, 1.537401574803149984, -2.901595197523589142E-16 ) ) ;
#8142=CARTESIAN_POINT ( 'NONE',  ( 1.403614904275686858E-14, 1.537401574803149984, -3.937007874015761910 ) ) ;
#8161=CARTESIAN_POINT ( 'NONE',  ( 4.194656359284241426E-16, 0.03937007874015747977, 3.405511811023621771 ) ) ;
#8178=ORIENTED_EDGE ( 'NONE', *, *, #42409, .T. ) ;
#8184=CARTESIAN_POINT ( 'NONE',  ( -0.4741693035498695252, 1.520070061304625408, 2.554858552206048738 ) ) ;
#8191=ORIENTED_EDGE ( 'NONE', *, *, #7492, .F. ) ;
#8192=AXIS2_PLACEMENT_3D ( 'NONE', #30838, #56094, #62415 ) ;
#8199=EDGE_CURVE ( 'NONE', #32861, #44548, #39071, .T. ) ;
#8202=VERTEX_POINT ( 'NONE', #69827 ) ;
#8215=AXIS2_PLACEMENT_3D ( 'NONE', #23552, #79591, #61860 ) ;
#8250=LINE ( 'NONE', #40231, #37397 ) ;
#8252=VECTOR ( 'NONE', #78653, 39.37007874015748143 ) ;
#8262=ORIENTED_EDGE ( 'NONE', *, *, #22956, .T. ) ;
#8263=ORIENTED_EDGE ( 'NONE', *, *, #80947, .F. ) ;
#8295=CARTESIAN_POINT ( 'NONE',  ( 0.5314960629921394730, 2.736617272820978108, -3.873860110281695412 ) ) ;
#8302=CARTESIAN_POINT ( 'NONE',  ( 1.857294464233405273, 1.070443199938752699, 0.08545185031211080529 ) ) ;
#8303=ADVANCED_FACE ( 'NONE', ( #68593 ), #12176, .F. ) ;
#8315=DIRECTION ( 'NONE',  ( 1.408710688920637755E-15, -1.000000000000000000, 4.918487082195260922E-30 ) ) ;
#8318=COLOUR_RGB ( '', 0.72549020, 0.75294118, 0.79215686) ;
#8327=CARTESIAN_POINT ( 'NONE',  ( 0.4492688262921352149, 1.384998324914241019, -1.544058616794434791 ) ) ;
#8333=FACE_OUTER_BOUND ( 'NONE', #43661, .T. ) ;
#8344=CARTESIAN_POINT ( 'NONE',  ( -0.3149606299212460159, 2.755905511811024056, -3.924389226575469625 ) ) ;
#8350=CARTESIAN_POINT ( 'NONE',  ( 0.4670044181572728936, 1.622388320715301147, -2.571776478002881561 ) ) ;
#8356=ADVANCED_FACE ( 'NONE', ( #4606 ), #43094, .F. ) ;
#8360=CARTESIAN_POINT ( 'NONE',  ( 3.898836503597932435, 2.697992270790282365, 0.5314960629921259283 ) ) ;
#8364=EDGE_LOOP ( 'NONE', ( #21501, #34901, #37005 ) ) ;
#8379=EDGE_LOOP ( 'NONE', ( #39070, #16362, #34965, #30302 ) ) ;
#8381=EDGE_LOOP ( 'NONE', ( #22954, #58872, #54936, #35606 ) ) ;
#8384=CARTESIAN_POINT ( 'NONE',  ( -1.559171609364246924, 0.3937007874015748254, 0.4177787735906735578 ) ) ;
#8390=CARTESIAN_POINT ( 'NONE',  ( -3.937007874015748143, 2.165354330708661568, -0.3149606299212600047 ) ) ;
#8396=CARTESIAN_POINT ( 'NONE',  ( -2.554262525012223062, 1.546132656481030043, 0.4744094488188971837 ) ) ;
#8416=LINE ( 'NONE', #2935, #69540 ) ;
#8422=CARTESIAN_POINT ( 'NONE',  ( -1.850419646634100301, 1.063020117359136263, -0.01785754392578375524 ) ) ;
#8432=EDGE_CURVE ( 'NONE', #36021, #65941, #31015, .T. ) ;
#8448=ORIENTED_EDGE ( 'NONE', *, *, #24627, .T. ) ;
#8453=CARTESIAN_POINT ( 'NONE',  ( -1.076935383196057749, -5.463695987328518425E-17, 0.3149606299212591720 ) ) ;
#8460=EDGE_CURVE ( 'NONE', #5432, #36021, #7097, .T. ) ;
#8479=CARTESIAN_POINT ( 'NONE',  ( -0.5314960629921122726, 2.755905511811024056, -3.937007874015763687 ) ) ;
#8485=ORIENTED_EDGE ( 'NONE', *, *, #75428, .F. ) ;
#8502=CARTESIAN_POINT ( 'NONE',  ( -0.5314960629921395840, 2.729373344522950440, 3.881211926161856507 ) ) ;
#8505=CARTESIAN_POINT ( 'NONE',  ( 3.929929591340561856, 1.125488309886446991, 0.2373865333886654438 ) ) ;
#8508=DIRECTION ( 'NONE',  ( 0.000000000000000000, 0.000000000000000000, -1.000000000000000000 ) ) ;
#8523=ADVANCED_FACE ( 'NONE', ( #1220 ), #58434, .T. ) ;
#8527=CARTESIAN_POINT ( 'NONE',  ( -0.4498537592782897998, 0.000000000000000000, -2.118110236220472675 ) ) ;
#8550=AXIS2_PLACEMENT_3D ( 'NONE', #25731, #51392, #38368 ) ;
#8566=CARTESIAN_POINT ( 'NONE',  ( 3.861376881555339757, 2.746034003362845866, -0.5314960629921258173 ) ) ;
#8593=VERTEX_POINT ( 'NONE', #38817 ) ;
#8595=ORIENTED_EDGE ( 'NONE', *, *, #57961, .F. ) ;
#8599=DIRECTION ( 'NONE',  ( 0.000000000000000000, -1.000000000000000000, -0.000000000000000000 ) ) ;
#8600=CARTESIAN_POINT ( 'NONE',  ( -0.5314960629921294810, 0.000000000000000000, 0.9881811337016621621 ) ) ;
#8602=AXIS2_PLACEMENT_3D ( 'NONE', #33269, #1287, #20636 ) ;
#8609=CARTESIAN_POINT ( 'NONE',  ( -1.109428599580102537, 1.093625931280370001, -0.1684409714770037092 ) ) ;
#8618=DIRECTION ( 'NONE',  ( 0.8660254037844361541, 0.000000000000000000, 0.5000000000000043299 ) ) ;
#8644=FACE_OUTER_BOUND ( 'NONE', #51295, .T. ) ;
#8663=CONICAL_SURFACE ( 'NONE', #82613, 3.444881889763779625, 0.7853981633974500554 ) ;
#8674=DIRECTION ( 'NONE',  ( 0.000000000000000000, 0.000000000000000000, -1.000000000000000000 ) ) ;
#8676=EDGE_CURVE ( 'NONE', #26273, #44534, #27067, .T. ) ;
#8677=ORIENTED_EDGE ( 'NONE', *, *, #14300, .F. ) ;
#8695=VERTEX_POINT ( 'NONE', #64495 ) ;
#8702=PLANE ( 'NONE',  #14134 ) ;
#8710=CARTESIAN_POINT ( 'NONE',  ( 0.5314960629921394730, 2.739927440807262915, -3.869764100875847213 ) ) ;
#8716=CARTESIAN_POINT ( 'NONE',  ( 1.854617417371074772, 1.067551433859868615, -0.06782095098398562005 ) ) ;
#8726=AXIS2_PLACEMENT_3D ( 'NONE', #13333, #65093, #7431 ) ;
#8742=CARTESIAN_POINT ( 'NONE',  ( -2.556891458315154519, 2.729656612766095947, 0.5314960629921260393 ) ) ;
#8746=DIRECTION ( 'NONE',  ( -0.000000000000000000, -1.000000000000000000, -0.000000000000000000 ) ) ;
#8748=FACE_OUTER_BOUND ( 'NONE', #40960, .T. ) ;
#8761=CARTESIAN_POINT ( 'NONE',  ( -3.900966923095589678, 2.687614851728675092, -0.5314960629921259283 ) ) ;
#8771=CARTESIAN_POINT ( 'NONE',  ( 3.831845081856512181, 2.755400581649067426, 0.5314960629921259283 ) ) ;
#8773=ORIENTED_EDGE ( 'NONE', *, *, #25189, .F. ) ;
#8774=VECTOR ( 'NONE', #29278, 39.37007874015748143 ) ;
#8790=ORIENTED_EDGE ( 'NONE', *, *, #44899, .T. ) ;
#8795=CARTESIAN_POINT ( 'NONE',  ( -1.491404278319911736, 1.136671166205875716, 0.2539434599294014827 ) ) ;
#8801=DIRECTION ( 'NONE',  ( 0.000000000000000000, -8.673617379884024625E-16, 1.000000000000000000 ) ) ;
#8806=ORIENTED_EDGE ( 'NONE', *, *, #13185, .T. ) ;
#8843=CARTESIAN_POINT ( 'NONE',  ( 0.000000000000000000, 0.04488074079120461107, -1.244489337948955221 ) ) ;
#8859=DIRECTION ( 'NONE',  ( -0.000000000000000000, -1.000000000000000000, -0.000000000000000000 ) ) ;
#8865=DIRECTION ( 'NONE',  ( 0.000000000000000000, 0.000000000000000000, -1.000000000000000000 ) ) ;
#8868=CARTESIAN_POINT ( 'NONE',  ( 0.000000000000000000, 2.755905511811024056, 0.000000000000000000 ) ) ;
#8869=CARTESIAN_POINT ( 'NONE',  ( -0.5314960629921122726, 2.755905511811024056, -3.937007874015763687 ) ) ;
#8884=DIRECTION ( 'NONE',  ( 0.000000000000000000, 0.000000000000000000, -1.000000000000000000 ) ) ;
#8893=ORIENTED_EDGE ( 'NONE', *, *, #15339, .T. ) ;
#8898=CIRCLE ( 'NONE', #66700, 0.1190944881889763746 ) ;
#8910=ADVANCED_FACE ( 'NONE', ( #65350 ), #16332, .F. ) ;
#8916=EDGE_CURVE ( 'NONE', #64866, #31453, #1542, .T. ) ;
#8920=CARTESIAN_POINT ( 'NONE',  ( -0.4623158380715545746, 0.02617651024168223331, 2.142213561789874543 ) ) ;
#8926=CARTESIAN_POINT ( 'NONE',  ( -0.5314960629921122726, 2.755905511811024056, -3.937007874015763687 ) ) ;
#8942=DIRECTION ( 'NONE',  ( 0.000000000000000000, -1.000000000000000000, -0.000000000000000000 ) ) ;
#8954=VECTOR ( 'NONE', #38090, 39.37007874015748143 ) ;
#8974=EDGE_CURVE ( 'NONE', #41616, #66374, #33355, .T. ) ;
#8979=ORIENTED_EDGE ( 'NONE', *, *, #57961, .T. ) ;
#8993=DIRECTION ( 'NONE',  ( 0.000000000000000000, 0.000000000000000000, 1.000000000000000000 ) ) ;
#8994=CIRCLE ( 'NONE', #6260, 3.228346456692913424 ) ;
#9011=CARTESIAN_POINT ( 'NONE',  ( -3.937007874015748143, 1.537401574803149984, 0.4744094488188970171 ) ) ;
#9018=DIRECTION ( 'NONE',  ( -0.8660254037844433705, 0.000000000000000000, 0.4999999999999920064 ) ) ;
#9035=DIRECTION ( 'NONE',  ( 0.000000000000000000, 0.000000000000000000, -1.000000000000000000 ) ) ;
#9042=DIRECTION ( 'NONE',  ( -0.000000000000000000, 1.000000000000000000, -0.000000000000000000 ) ) ;
#9050=VECTOR ( 'NONE', #11045, 39.37007874015748143 ) ;
#9052=CARTESIAN_POINT ( 'NONE',  ( 0.000000000000000000, 1.724409448818897905, 0.000000000000000000 ) ) ;
#9057=ADVANCED_FACE ( 'NONE', ( #55583 ), #73744, .F. ) ;
#9068=CARTESIAN_POINT ( 'NONE',  ( 1.403614904275686858E-14, 1.537401574803149984, -3.937007874015761910 ) ) ;
#9070=VERTEX_POINT ( 'NONE', #21965 ) ;
#9114=VERTEX_POINT ( 'NONE', #80065 ) ;
#9117=CARTESIAN_POINT ( 'NONE',  ( -1.600194884102785764, 1.375860811871311373, 0.4460756753617342030 ) ) ;
#9118=AXIS2_PLACEMENT_3D ( 'NONE', #80440, #66551, #8884 ) ;
#9125=CARTESIAN_POINT ( 'NONE',  ( -1.076935383196057305, 2.559055118110236560, -0.3149606299212599492 ) ) ;
#9136=CARTESIAN_POINT ( 'NONE',  ( 0.000000000000000000, 0.000000000000000000, 0.000000000000000000 ) ) ;
#9138=CARTESIAN_POINT ( 'NONE',  ( 1.882930639362819347, 1.098283573398303403, -0.1802708669123839202 ) ) ;
#9160=EDGE_CURVE ( 'NONE', #28368, #3377, #48571, .T. ) ;
#9162=CARTESIAN_POINT ( 'NONE',  ( -3.937007874015748143, 1.537401574803149984, -2.901595197523589142E-16 ) ) ;
#9169=EDGE_LOOP ( 'NONE', ( #16679, #10460, #9228, #11234 ) ) ;
#9181=FACE_BOUND ( 'NONE', #58252, .T. ) ;
#9189=CARTESIAN_POINT ( 'NONE',  ( -3.908320185825792326, 1.537401574803149984, 0.4744094488188970171 ) ) ;
#9211=ORIENTED_EDGE ( 'NONE', *, *, #61964, .F. ) ;
#9214=CARTESIAN_POINT ( 'NONE',  ( 2.869792031447826908, 1.067551433859866616, 0.06782095098396989652 ) ) ;
#9225=ORIENTED_EDGE ( 'NONE', *, *, #69615, .T. ) ;
#9228=ORIENTED_EDGE ( 'NONE', *, *, #53323, .F. ) ;
#9254=ADVANCED_FACE ( 'NONE', ( #22383 ), #52586, .F. ) ;
#9256=CARTESIAN_POINT ( 'NONE',  ( 0.5314960629920859603, 2.755905511811024056, 3.821484228344198986 ) ) ;
#9265=DIRECTION ( 'NONE',  ( 1.000000000000000000, 0.000000000000000000, -0.000000000000000000 ) ) ;
#9275=LINE ( 'NONE', #41257, #44043 ) ;
#9282=VERTEX_POINT ( 'NONE', #60268 ) ;
#9290=DIRECTION ( 'NONE',  ( 0.000000000000000000, -1.000000000000000000, 0.000000000000000000 ) ) ;
#9309=CARTESIAN_POINT ( 'NONE',  ( 0.1180926326102879620, 1.077616795999332133, -2.860488110875698542 ) ) ;
#9368=CARTESIAN_POINT ( 'NONE',  ( 0.5314960629921396951, 2.755905511811024056, -3.937007874015760578 ) ) ;
#9376=EDGE_CURVE ( 'NONE', #51564, #6368, #44798, .T. ) ;
#9379=CARTESIAN_POINT ( 'NONE',  ( -1.713362436456637550, 1.196869643373675407, 0.3303709977379641893 ) ) ;
#9381=CARTESIAN_POINT ( 'NONE',  ( 0.000000000000000000, 0.000000000000000000, 0.000000000000000000 ) ) ;
#9399=EDGE_CURVE ( 'NONE', #78980, #67465, #35125, .T. ) ;
#9416=CARTESIAN_POINT ( 'NONE',  ( -0.2248261898302304773, 1.118407866122133276, -2.823087432092973081 ) ) ;
#9418=DIRECTION ( 'NONE',  ( -3.491481338843132961E-15, -0.000000000000000000, 1.000000000000000000 ) ) ;
#9419=EDGE_CURVE ( 'NONE', #44018, #69029, #41725, .T. ) ;
#9421=ORIENTED_EDGE ( 'NONE', *, *, #16548, .F. ) ;
#9426=DIRECTION ( 'NONE',  ( 0.000000000000000000, 0.000000000000000000, -1.000000000000000000 ) ) ;
#9427=LINE ( 'NONE', #72984, #81312 ) ;
#9428=CARTESIAN_POINT ( 'NONE',  ( -0.03443470937339728616, 0.2755905511811023723, -1.537015892239756099 ) ) ;
#9434=ORIENTED_EDGE ( 'NONE', *, *, #69637, .T. ) ;
#9437=DIRECTION ( 'NONE',  ( 0.000000000000000000, -1.000000000000000000, 0.000000000000000000 ) ) ;
#9440=DIRECTION ( 'NONE',  ( -0.000000000000000000, -1.000000000000000000, 0.000000000000000000 ) ) ;
#9443=CARTESIAN_POINT ( 'NONE',  ( 0.000000000000000000, 2.755905511811024056, 0.000000000000000000 ) ) ;
#9450=CARTESIAN_POINT ( 'NONE',  ( 2.557182324916567495, 1.572090529166660922, -0.4732185887570796723 ) ) ;
#9472=ADVANCED_FACE ( 'NONE', ( #15667 ), #2618, .F. ) ;
#9473=CARTESIAN_POINT ( 'NONE',  ( -1.291027602697912169, 0.1377952755905511861, 0.5830028338522512676 ) ) ;
#9493=CARTESIAN_POINT ( 'NONE',  ( 4.218763579739897660E-16, 0.000000000000000000, 3.444881889763779625 ) ) ;
#9504=VERTEX_POINT ( 'NONE', #15250 ) ;
#9513=CARTESIAN_POINT ( 'NONE',  ( 3.924389226575468737, 2.755905511811024056, 0.3149606299212598381 ) ) ;
#9516=AXIS2_PLACEMENT_3D ( 'NONE', #49779, #62840, #9838 ) ;
#9524=ORIENTED_EDGE ( 'NONE', *, *, #65450, .F. ) ;
#9529=CARTESIAN_POINT ( 'NONE',  ( 1.854472803289052507, 2.716535433070866645, -0.5314960629921260393 ) ) ;
#9532=ADVANCED_FACE ( 'NONE', ( #16497 ), #28274, .F. ) ;
#9540=VECTOR ( 'NONE', #69101, 39.37007874015748143 ) ;
#9565=EDGE_CURVE ( 'NONE', #9606, #7036, #30669, .T. ) ;
#9604=EDGE_LOOP ( 'NONE', ( #75883, #39629, #28440, #67089, #1139, #78158 ) ) ;
#9606=VERTEX_POINT ( 'NONE', #29514 ) ;
#9628=EDGE_CURVE ( 'NONE', #56091, #63201, #69474, .T. ) ;
#9636=EDGE_LOOP ( 'NONE', ( #65638, #34482, #32642, #31123 ) ) ;
#9637=AXIS2_PLACEMENT_3D ( 'NONE', #22880, #28780, #47296 ) ;
#9658=DIRECTION ( 'NONE',  ( 0.000000000000000000, -1.601283208593975810E-15, -1.000000000000000000 ) ) ;
#9667=CARTESIAN_POINT ( 'NONE',  ( 0.5314960629920849611, 2.697625129285034618, 3.898413161119336223 ) ) ;
#9694=VECTOR ( 'NONE', #5943, 39.37007874015748143 ) ;
#9696=CARTESIAN_POINT ( 'NONE',  ( 0.2981046825593872684, 1.168156273747579688, -1.428012540953041976 ) ) ;
#9706=EDGE_LOOP ( 'NONE', ( #61651, #70902, #69739, #73099, #58548, #48638, #35177 ) ) ;
#9709=VERTEX_POINT ( 'NONE', #42955 ) ;
#9715=CARTESIAN_POINT ( 'NONE',  ( -0.4741708390789116656, 1.554782515222133510, -2.554855015577685240 ) ) ;
#9720=CARTESIAN_POINT ( 'NONE',  ( 0.06818963398612189197, 1.067605756753703172, -2.869741741654902256 ) ) ;
#9726=ORIENTED_EDGE ( 'NONE', *, *, #5310, .F. ) ;
#9731=EDGE_CURVE ( 'NONE', #65535, #64697, #30334, .T. ) ;
#9752=DIRECTION ( 'NONE',  ( -1.000000000000000000, 0.000000000000000000, -3.491481338843132961E-15 ) ) ;
#9775=CARTESIAN_POINT ( 'NONE',  ( -2.630268417803885317, 1.724409448818897905, 0.4359958488159718093 ) ) ;
#9792=CARTESIAN_POINT ( 'NONE',  ( 0.000000000000000000, 2.165354330708661568, 0.000000000000000000 ) ) ;
#9793=DIRECTION ( 'NONE',  ( -0.000000000000000000, -1.000000000000000000, -0.000000000000000000 ) ) ;
#9799=VERTEX_POINT ( 'NONE', #33148 ) ;
#9806=CARTESIAN_POINT ( 'NONE',  ( -0.01585754980764347150, 1.062992125984252745, 1.122047244094488638 ) ) ;
#9822=ADVANCED_FACE ( 'NONE', ( #5084 ), #17730, .F. ) ;
#9830=CARTESIAN_POINT ( 'NONE',  ( -0.6299212598425230070, 0.000000000000000000, 0.9285414500055690912 ) ) ;
#9834=VERTEX_POINT ( 'NONE', #43358 ) ;
#9835=ORIENTED_EDGE ( 'NONE', *, *, #67540, .T. ) ;
#9838=DIRECTION ( 'NONE',  ( 0.000000000000000000, 0.000000000000000000, -1.000000000000000000 ) ) ;
#9839=CARTESIAN_POINT ( 'NONE',  ( -3.237502116762790205, 2.729657714433391114, -0.5314960629921260393 ) ) ;
#9847=VECTOR ( 'NONE', #27578, 39.37007874015748143 ) ;
#9850=ORIENTED_EDGE ( 'NONE', *, *, #10428, .F. ) ;
#9852=CARTESIAN_POINT ( 'NONE',  ( -1.044082653748674261, 1.299084363779800411, 0.4113579841234183410 ) ) ;
#9854=DIRECTION ( 'NONE',  ( 0.000000000000000000, 0.000000000000000000, 1.000000000000000000 ) ) ;
#9857=CARTESIAN_POINT ( 'NONE',  ( 1.840814949217404406, 2.729664702882089067, 0.5314960629921260393 ) ) ;
#9859=CARTESIAN_POINT ( 'NONE',  ( -1.559171609364246924, 0.3937007874015748254, 0.4177787735906735578 ) ) ;
#9860=DIRECTION ( 'NONE',  ( 0.000000000000000000, 0.000000000000000000, -1.000000000000000000 ) ) ;
#9887=CARTESIAN_POINT ( 'NONE',  ( 0.2642730939577003224, 1.143123705106234622, 1.923655279115566996 ) ) ;
#9892=VERTEX_POINT ( 'NONE', #81711 ) ;
#9901=DIRECTION ( 'NONE',  ( -0.000000000000000000, -1.000000000000000000, -0.000000000000000000 ) ) ;
#9926=CARTESIAN_POINT ( 'NONE',  ( 1.016821367227983552, 1.537401574803149984, 0.4744094488188975722 ) ) ;
#9937=DIRECTION ( 'NONE',  ( 0.000000000000000000, -0.5150380749100564870, -0.8571673007021107793 ) ) ;
#9951=VERTEX_POINT ( 'NONE', #71031 ) ;
#9953=B_SPLINE_CURVE_WITH_KNOTS ( 'NONE', 3,
 ( #3757, #37797, #48772, #62656 ),
 .UNSPECIFIED., .F., .F.,
 ( 4, 4 ),
 ( 0.2160131946215620991, 0.2174264745397616883 ),
 .UNSPECIFIED. ) ;
#9958=CARTESIAN_POINT ( 'NONE',  ( 1.915796337058191412, 1.134406187872327054, -0.2508088161067802413 ) ) ;
#9959=EDGE_CURVE ( 'NONE', #19993, #312, #74981, .T. ) ;
#9964=DIRECTION ( 'NONE',  ( -0.000000000000000000, -1.000000000000000000, 0.000000000000000000 ) ) ;
#9965=CARTESIAN_POINT ( 'NONE',  ( -0.4359958488159811907, 1.724409448818897905, 2.630268417803910186 ) ) ;
#9991=PLANE ( 'NONE',  #42565 ) ;
#9992=DIRECTION ( 'NONE',  ( 0.000000000000000000, 1.000000000000000000, 0.000000000000000000 ) ) ;
#10021=ORIENTED_EDGE ( 'NONE', *, *, #15160, .F. ) ;
#10025=AXIS2_PLACEMENT_3D ( 'NONE', #641, #7362, #20827 ) ;
#10031=EDGE_CURVE ( 'NONE', #76587, #75749, #43153, .T. ) ;
#10035=VERTEX_POINT ( 'NONE', #37480 ) ;
#10045=CIRCLE ( 'NONE', #57050, 1.122047244094488194 ) ;
#10047=LINE ( 'NONE', #61380, #41761 ) ;
#10055=EDGE_LOOP ( 'NONE', ( #66268, #12524, #70904, #21274 ) ) ;
#10082=DIRECTION ( 'NONE',  ( 1.000000000000000000, 0.000000000000000000, 3.491481338843135327E-15 ) ) ;
#10103=PLANE ( 'NONE',  #29293 ) ;
#10108=AXIS2_PLACEMENT_3D ( 'NONE', #15336, #41001, #28361 ) ;
#10112=ORIENTED_EDGE ( 'NONE', *, *, #43446, .F. ) ;
#10125=ORIENTED_EDGE ( 'NONE', *, *, #38297, .F. ) ;
#10140=DIRECTION ( 'NONE',  ( -3.491481338843132961E-15, -0.000000000000000000, 1.000000000000000000 ) ) ;
#10144=ORIENTED_EDGE ( 'NONE', *, *, #22709, .F. ) ;
#10175=CARTESIAN_POINT ( 'NONE',  ( 0.5314960629921372526, 2.716535433070866645, -3.224202737261813834 ) ) ;
#10182=CARTESIAN_POINT ( 'NONE',  ( -0.3251038240001069002, 1.191559816073523237, -1.073976752645962041 ) ) ;
#10213=CARTESIAN_POINT ( 'NONE',  ( -1.627024087650608131, 1.136692823381468598, 0.2539777673203736374 ) ) ;
#10218=VECTOR ( 'NONE', #68138, 39.37007874015748143 ) ;
#10222=ORIENTED_EDGE ( 'NONE', *, *, #16744, .T. ) ;
#10238=DIRECTION ( 'NONE',  ( -0.000000000000000000, -1.000000000000000000, -0.000000000000000000 ) ) ;
#10256=ORIENTED_EDGE ( 'NONE', *, *, #82229, .T. ) ;
#10257=CIRCLE ( 'NONE', #68057, 0.5118110236220472231 ) ;
#10260=AXIS2_PLACEMENT_3D ( 'NONE', #1601, #65991, #2013 ) ;
#10262=CARTESIAN_POINT ( 'NONE',  ( -1.017211938244154013, 1.569780109764696396, 0.4735748448513866782 ) ) ;
#10263=CARTESIAN_POINT ( 'NONE',  ( 2.554262525012302110, 1.537401574803149984, 0.4744094488188975722 ) ) ;
#10265=CARTESIAN_POINT ( 'NONE',  ( -0.03443470937339728616, 0.000000000000000000, -1.537015892239756099 ) ) ;
#10273=CARTESIAN_POINT ( 'NONE',  ( -1.084117400955593835, 1.161042249202826504, 0.2904890618464239238 ) ) ;
#10274=SHAPE_DEFINITION_REPRESENTATION ( #58731, #7298 ) ;
#10278=CARTESIAN_POINT ( 'NONE',  ( 1.854472803289052507, 2.716535433070866645, 0.5314960629921260393 ) ) ;
#10289=CARTESIAN_POINT ( 'NONE',  ( 2.554262525012262586, 1.537401574803149984, -0.4744094488188970171 ) ) ;
#10296=EDGE_CURVE ( 'NONE', #69029, #37547, #42495, .T. ) ;
#10303=CARTESIAN_POINT ( 'NONE',  ( -3.937007874015748143, 2.755905511811024056, -0.5314960629921260393 ) ) ;
#10311=CARTESIAN_POINT ( 'NONE',  ( 0.3234312996134217078, 1.189126250296160592, 1.964625460076719898 ) ) ;
#10314=CARTESIAN_POINT ( 'NONE',  ( 1.524059884292196751E-16, 0.04488074079120461107, 1.244489337948955221 ) ) ;
#10316=VERTEX_POINT ( 'NONE', #2415 ) ;
#10320=CIRCLE ( 'NONE', #57319, 2.637795275590551380 ) ;
#10321=DIRECTION ( 'NONE',  ( 0.000000000000000000, 1.000000000000000000, -0.000000000000000000 ) ) ;
#10373=ADVANCED_FACE ( 'NONE', ( #66812 ), #14290, .F. ) ;
#10381=CARTESIAN_POINT ( 'NONE',  ( 0.000000000000000000, 0.4374015748031496176, 0.000000000000000000 ) ) ;
#10383=AXIS2_PLACEMENT_3D ( 'NONE', #16024, #14780, #66116 ) ;
#10385=CARTESIAN_POINT ( 'NONE',  ( 2.112655059233934818, 1.697151583350148263, 0.4469586986359062042 ) ) ;
#10387=LINE ( 'NONE', #36044, #22396 ) ;
#10392=CARTESIAN_POINT ( 'NONE',  ( -0.4417575354491581896, 1.710976477253047801, 2.620897244026389572 ) ) ;
#10428=EDGE_CURVE ( 'NONE', #50308, #75749, #17721, .T. ) ;
#10439=AXIS2_PLACEMENT_3D ( 'NONE', #61565, #5958, #45913 ) ;
#10444=VERTEX_POINT ( 'NONE', #73112 ) ;
#10452=ADVANCED_FACE ( 'NONE', ( #79032 ), #78612, .F. ) ;
#10458=EDGE_LOOP ( 'NONE', ( #13975, #70018, #81969, #35058 ) ) ;
#10460=ORIENTED_EDGE ( 'NONE', *, *, #32216, .F. ) ;
#10476=FACE_OUTER_BOUND ( 'NONE', #13157, .T. ) ;
#10477=ORIENTED_EDGE ( 'NONE', *, *, #54568, .T. ) ;
#10483=CARTESIAN_POINT ( 'NONE',  ( -0.01548373826924297550, 1.062992125984252079, 3.937007874015748143 ) ) ;
#10511=DIRECTION ( 'NONE',  ( 1.000000000000000000, 1.387778780781445676E-15, 0.000000000000000000 ) ) ;
#10521=FACE_BOUND ( 'NONE', #76585, .T. ) ;
#10527=DIRECTION ( 'NONE',  ( 0.000000000000000000, 0.000000000000000000, -1.000000000000000000 ) ) ;
#10536=CARTESIAN_POINT ( 'NONE',  ( 0.000000000000000000, 0.000000000000000000, 0.000000000000000000 ) ) ;
#10543=EDGE_LOOP ( 'NONE', ( #46039, #64264, #80035, #68202 ) ) ;
#10568=EDGE_CURVE ( 'NONE', #49988, #76797, #52483, .T. ) ;
#10585=EDGE_CURVE ( 'NONE', #55865, #40881, #20698, .T. ) ;
#10597=CARTESIAN_POINT ( 'NONE',  ( -2.784923006909794996, 1.160811571118585572, 0.2889173282905625473 ) ) ;
#10630=DIRECTION ( 'NONE',  ( 0.000000000000000000, 0.000000000000000000, -1.000000000000000000 ) ) ;
#10631=DIRECTION ( 'NONE',  ( 0.000000000000000000, 1.000000000000000000, 8.673617379884024625E-16 ) ) ;
#10645=CARTESIAN_POINT ( 'NONE',  ( -0.07858598928476964729, 1.069287512630840764, 1.119396547425128841 ) ) ;
#10659=VECTOR ( 'NONE', #42839, 39.37007874015748143 ) ;
#10668=CARTESIAN_POINT ( 'NONE',  ( -0.4426497960380713637, 1.366130357955172014, -2.619358585163587438 ) ) ;
#10674=VERTEX_POINT ( 'NONE', #68860 ) ;
#10677=CARTESIAN_POINT ( 'NONE',  ( 3.937007874015748143, 1.724409448818897905, -0.6299212598425196763 ) ) ;
#10682=EDGE_CURVE ( 'NONE', #69303, #2585, #11577, .T. ) ;
#10689=CARTESIAN_POINT ( 'NONE',  ( -1.115269913029420135, 1.079232407413005523, 0.1240654315417908660 ) ) ;
#10697=CARTESIAN_POINT ( 'NONE',  ( -3.908320185825792326, 1.537401574803149984, -0.4744094488188975722 ) ) ;
#10704=DIRECTION ( 'NONE',  ( -0.8660254037844432595, 0.000000000000000000, 0.4999999999999918954 ) ) ;
#10733=CARTESIAN_POINT ( 'NONE',  ( -2.169549097624052791, 1.554815631980116297, -0.4741686481756397509 ) ) ;
#10771=CARTESIAN_POINT ( 'NONE',  ( -1.313877454013331780, 0.2755905511811023723, 0.8967544760595740350 ) ) ;
#10775=CARTESIAN_POINT ( 'NONE',  ( -0.5314960629921323676, 2.755905511811024056, 1.813482582612291560 ) ) ;
#10776=CARTESIAN_POINT ( 'NONE',  ( -0.5314960629921146040, 2.755905511811024056, -3.264097702071374840 ) ) ;
#10785=VERTEX_POINT ( 'NONE', #61720 ) ;
#10787=DIRECTION ( 'NONE',  ( 0.000000000000000000, -1.000000000000000000, 0.000000000000000000 ) ) ;
#10814=CARTESIAN_POINT ( 'NONE',  ( -3.884611959489589594, 2.725289161120230563, 0.5314960629921258173 ) ) ;
#10817=ORIENTED_EDGE ( 'NONE', *, *, #57389, .F. ) ;
#10825=CYLINDRICAL_SURFACE ( 'NONE', #11580, 0.4744094488188972947 ) ;
#10832=CONICAL_SURFACE ( 'NONE', #5477, 3.228346456692913424, 0.7853981633974500554 ) ;
#10860=ORIENTED_EDGE ( 'NONE', *, *, #1370, .F. ) ;
#10869=FACE_OUTER_BOUND ( 'NONE', #932, .T. ) ;
#10876=CARTESIAN_POINT ( 'NONE',  ( -3.184294706754630777, 2.755905511811024056, 0.5314960629921260393 ) ) ;
#10884=CARTESIAN_POINT ( 'NONE',  ( -0.3772065495488707287, 1.248034150500769046, 3.918934030054451512 ) ) ;
#10898=ADVANCED_FACE ( 'NONE', ( #22592 ), #75601, .F. ) ;
#10899=CONICAL_SURFACE ( 'NONE', #37796, 0.1771653543307085410, 1.029744258676653645 ) ;
#10908=LINE ( 'NONE', #42873, #7553 ) ;
#10912=CARTESIAN_POINT ( 'NONE',  ( 0.000000000000000000, 0.03937007874015747977, 0.000000000000000000 ) ) ;
#10937=DIRECTION ( 'NONE',  ( 0.000000000000000000, -0.000000000000000000, 1.000000000000000000 ) ) ;
#10944=ORIENTED_EDGE ( 'NONE', *, *, #51527, .F. ) ;
#10950=DIRECTION ( 'NONE',  ( 0.000000000000000000, 0.000000000000000000, -1.000000000000000000 ) ) ;
#10955=CARTESIAN_POINT ( 'NONE',  ( 2.554262525012262586, 1.537401574803149984, -0.4744094488188970171 ) ) ;
#10995=CARTESIAN_POINT ( 'NONE',  ( -2.846947862837596599, 1.092324130688937744, -0.1650676745531605427 ) ) ;
#11009=CYLINDRICAL_SURFACE ( 'NONE', #5806, 0.4744094488188972947 ) ;
#11015=CYLINDRICAL_SURFACE ( 'NONE', #35683, 0.4744094488188972947 ) ;
#11032=CARTESIAN_POINT ( 'NONE',  ( -1.519422763189357539, 0.000000000000000000, 0.7302211324797359682 ) ) ;
#11033=CARTESIAN_POINT ( 'NONE',  ( 0.000000000000000000, 2.677165354330708791, 0.000000000000000000 ) ) ;
#11040=VERTEX_POINT ( 'NONE', #18748 ) ;
#11045=DIRECTION ( 'NONE',  ( 9.381338752702735711E-17, -0.6427876096865389188, 0.7660444431189783465 ) ) ;
#11056=CARTESIAN_POINT ( 'NONE',  ( 0.000000000000000000, 2.755905511811024056, 0.000000000000000000 ) ) ;
#11057=CARTESIAN_POINT ( 'NONE',  ( -0.5314960629921325896, 2.755905511811024056, 1.895394334970790018 ) ) ;
#11058=ORIENTED_EDGE ( 'NONE', *, *, #82624, .F. ) ;
#11073=AXIS2_PLACEMENT_3D ( 'NONE', #8142, #33807, #39276 ) ;
#11074=DIRECTION ( 'NONE',  ( 0.000000000000000000, 1.000000000000000000, -0.000000000000000000 ) ) ;
#11078=ORIENTED_EDGE ( 'NONE', *, *, #15825, .T. ) ;
#11099=EDGE_CURVE ( 'NONE', #77311, #65182, #3522, .T. ) ;
#11104=CARTESIAN_POINT ( 'NONE',  ( -3.910251735077579838, 1.664246877830559024, -0.4582626050727204858 ) ) ;
#11119=CARTESIAN_POINT ( 'NONE',  ( 1.102321318565061548, 1.111600770690012840, 0.2114527220942730157 ) ) ;
#11133=CARTESIAN_POINT ( 'NONE',  ( 0.1807843743677491344, 1.098495470880705538, 1.883124800463723991 ) ) ;
#11137=ORIENTED_EDGE ( 'NONE', *, *, #76918, .T. ) ;
#11147=EDGE_CURVE ( 'NONE', #58782, #51415, #50310, .T. ) ;
#11150=CARTESIAN_POINT ( 'NONE',  ( -0.4744094488189006809, 1.506132068098321675, 1.016821367227982220 ) ) ;
#11151=CARTESIAN_POINT ( 'NONE',  ( 3.912088859918621431, 1.709704544164725615, 0.4423030945488138355 ) ) ;
#11172=AXIS2_PLACEMENT_3D ( 'NONE', #35556, #28823, #62056 ) ;
#11181=VERTEX_POINT ( 'NONE', #26299 ) ;
#11193=AXIS2_PLACEMENT_3D ( 'NONE', #3376, #68188, #54710 ) ;
#11199=ORIENTED_EDGE ( 'NONE', *, *, #24920, .F. ) ;
#11208=DIRECTION ( 'NONE',  ( 0.000000000000000000, 0.000000000000000000, 1.000000000000000000 ) ) ;
#11230=CARTESIAN_POINT ( 'NONE',  ( -3.870235431238101764, 2.740199102106095186, 0.5314960629921260393 ) ) ;
#11232=CONICAL_SURFACE ( 'NONE', #19260, 3.228346456692913424, 0.7853981633974500554 ) ;
#11234=ORIENTED_EDGE ( 'NONE', *, *, #4397, .F. ) ;
#11248=CARTESIAN_POINT ( 'NONE',  ( 0.4698424923132817899, 1.469648236684818476, 2.565231856145545830 ) ) ;
#11261=ORIENTED_EDGE ( 'NONE', *, *, #75321, .F. ) ;
#11289=AXIS2_PLACEMENT_3D ( 'NONE', #46326, #65295, #21910 ) ;
#11293=ORIENTED_EDGE ( 'NONE', *, *, #75428, .T. ) ;
#11296=VERTEX_POINT ( 'NONE', #57857 ) ;
#11298=CARTESIAN_POINT ( 'NONE',  ( 0.6299212598425341092, 1.724409448818898127, -3.937007874015759690 ) ) ;
#11302=CARTESIAN_POINT ( 'NONE',  ( -0.4029579088642626372, 1.286547554808001648, 3.916341449869456426 ) ) ;
#11321=CARTESIAN_POINT ( 'NONE',  ( -2.113943251734124118, 1.379671404989104122, 0.4476723508032736110 ) ) ;
#11333=EDGE_CURVE ( 'NONE', #66374, #21108, #81518, .T. ) ;
#11339=CARTESIAN_POINT ( 'NONE',  ( -3.934129746973768160, 1.087346627047580006, 0.1532148504152880952 ) ) ;
#11341=B_SPLINE_CURVE_WITH_KNOTS ( 'NONE', 3,
 ( #11057, #6385, #5968, #69541 ),
 .UNSPECIFIED., .F., .F.,
 ( 4, 4 ),
 ( 1.009076915740197753E-06, 0.001443158937089476486 ),
 .UNSPECIFIED. ) ;
#11356=DIRECTION ( 'NONE',  ( -3.491481338843132961E-15, -0.000000000000000000, 1.000000000000000000 ) ) ;
#11360=ORIENTED_EDGE ( 'NONE', *, *, #34082, .T. ) ;
#11362=VECTOR ( 'NONE', #75456, 39.37007874015748143 ) ;
#11364=ORIENTED_EDGE ( 'NONE', *, *, #22547, .F. ) ;
#11374=CARTESIAN_POINT ( 'NONE',  ( 0.4426658557721722120, 1.366171107244630534, -2.619331181873139069 ) ) ;
#11406=ADVANCED_FACE ( 'NONE', ( #57032 ), #82727, .F. ) ;
#11412=DIRECTION ( 'NONE',  ( 1.000000000000000000, 0.000000000000000000, -0.000000000000000000 ) ) ;
#11415=CARTESIAN_POINT ( 'NONE',  ( -2.593354744918267230, 1.408268389154264222, -0.4567427728026662304 ) ) ;
#11418=CARTESIAN_POINT ( 'NONE',  ( -0.05603898182074958101, 1.066283915671629945, -1.446447749318907183 ) ) ;
#11425=CIRCLE ( 'NONE', #20850, 3.937007874015748143 ) ;
#11430=CARTESIAN_POINT ( 'NONE',  ( 0.3760314581298215830, 1.247744516244858604, -1.057212048078999933 ) ) ;
#11433=FACE_OUTER_BOUND ( 'NONE', #60132, .T. ) ;
#11438=CARTESIAN_POINT ( 'NONE',  ( -0.4682706818399092197, 1.459764456743772199, -3.909061641404189658 ) ) ;
#11458=ORIENTED_EDGE ( 'NONE', *, *, #35860, .F. ) ;
#11463=LINE ( 'NONE', #18192, #9050 ) ;
#11476=CARTESIAN_POINT ( 'NONE',  ( -0.08519462842575996342, 1.070400731138068995, -1.857255144359619470 ) ) ;
#11483=CONICAL_SURFACE ( 'NONE', #59842, 2.165354330708661568, 0.7853981633974500554 ) ;
#11506=FILL_AREA_STYLE_COLOUR ( '', #8318 ) ;
#11521=CARTESIAN_POINT ( 'NONE',  ( -0.3003296953576023443, 1.169860122871907882, 1.947534171620900922 ) ) ;
#11535=CARTESIAN_POINT ( 'NONE',  ( 1.120401492038572977, 1.066895646367433503, -0.06275413064580409594 ) ) ;
#11555=EDGE_CURVE ( 'NONE', #45807, #60217, #35784, .T. ) ;
#11577=CIRCLE ( 'NONE', #29050, 3.937007874015748143 ) ;
#11580=AXIS2_PLACEMENT_3D ( 'NONE', #73981, #68078, #16327 ) ;
#11599=ORIENTED_EDGE ( 'NONE', *, *, #73594, .F. ) ;
#11600=CARTESIAN_POINT ( 'NONE',  ( 0.000000000000000000, 2.559055118110236560, 0.000000000000000000 ) ) ;
#11601=CIRCLE ( 'NONE', #73426, 0.3149606299212597271 ) ;
#11606=DIRECTION ( 'NONE',  ( -0.000000000000000000, 1.000000000000000000, -0.000000000000000000 ) ) ;
#11607=CARTESIAN_POINT ( 'NONE',  ( -0.6299212598425059095, 2.165354330708661568, -3.937007874015764131 ) ) ;
#11617=DIRECTION ( 'NONE',  ( -3.491481338843132961E-15, -0.000000000000000000, 1.000000000000000000 ) ) ;
#11623=DIRECTION ( 'NONE',  ( 0.000000000000000000, 1.000000000000000000, -0.000000000000000000 ) ) ;
#11624=ADVANCED_FACE ( 'NONE', ( #72177 ), #57252, .F. ) ;
#11625=CARTESIAN_POINT ( 'NONE',  ( -3.937007874015748143, 2.559055118110236560, 0.3149606299212596716 ) ) ;
#11630=EDGE_CURVE ( 'NONE', #33945, #30219, #10257, .T. ) ;
#11648=CARTESIAN_POINT ( 'NONE',  ( -3.821484228344193657, 2.755905511811024056, 0.5314960629921260393 ) ) ;
#11656=AXIS2_PLACEMENT_3D ( 'NONE', #8390, #34055, #8801 ) ;
#11666=CARTESIAN_POINT ( 'NONE',  ( 0.3304432287027126991, 1.196939817260626926, -1.404940052879173118 ) ) ;
#11670=DIRECTION ( 'NONE',  ( 0.000000000000000000, -1.000000000000000000, 0.000000000000000000 ) ) ;
#11696=ORIENTED_EDGE ( 'NONE', *, *, #80626, .F. ) ;
#11698=VECTOR ( 'NONE', #9418, 39.37007874015748143 ) ;
#11714=VERTEX_POINT ( 'NONE', #1890 ) ;
#11716=LINE ( 'NONE', #18437, #61434 ) ;
#11717=ORIENTED_EDGE ( 'NONE', *, *, #27675, .T. ) ;
#11723=DIRECTION ( 'NONE',  ( 0.000000000000000000, 0.000000000000000000, -1.000000000000000000 ) ) ;
#11732=ADVANCED_FACE ( 'NONE', ( #15355 ), #40597, .F. ) ;
#11762=CARTESIAN_POINT ( 'NONE',  ( 0.000000000000000000, 2.755905511811024056, 0.000000000000000000 ) ) ;
#11766=DIRECTION ( 'NONE',  ( -0.000000000000000000, -1.000000000000000000, -0.000000000000000000 ) ) ;
#11767=ORIENTED_EDGE ( 'NONE', *, *, #63922, .F. ) ;
#11768=CARTESIAN_POINT ( 'NONE',  ( 0.000000000000000000, 2.677165354330708791, 0.000000000000000000 ) ) ;
#11771=B_SPLINE_CURVE_WITH_KNOTS ( 'NONE', 3,
 ( #77512, #34560, #33725, #65731, #66135, #21098, #73280, #72450, #28654, #14799, #46757, #41285, #22750, #78774, #80024, #8064, #28235, #61051, #66971, #21925, #35386, #72031 ),
 .UNSPECIFIED., .F., .F.,
 ( 4, 2, 2, 2, 2, 2, 2, 2, 2, 2, 4 ),
 ( 0.002118322035362868189, 0.002486146450160856784, 0.002853970864958844944, 0.003589619694554808255, 0.004325268524150771565, 0.005060917353746734876, 0.005796566183342697319, 0.006532215012938659762, 0.006900039427736632744, 0.007267863842534605726, 0.008003512672130536076 ),
 .UNSPECIFIED. ) ;
#11783=VERTEX_POINT ( 'NONE', #78920 ) ;
#11796=EDGE_LOOP ( 'NONE', ( #61593, #52239, #30726, #27108 ) ) ;
#11818=VECTOR ( 'NONE', #21480, 39.37007874015748143 ) ;
#11832=CARTESIAN_POINT ( 'NONE',  ( -2.856580783922622047, 1.081851677178485405, -0.1334749385307413549 ) ) ;
#11844=CARTESIAN_POINT ( 'NONE',  ( 0.3461855724062893880, 1.212665435597622965, -1.067367761115870728 ) ) ;
#11847=CARTESIAN_POINT ( 'NONE',  ( 2.154527559055117170, 0.03937007874015747977, 0.4677827689124997024 ) ) ;
#11852=CARTESIAN_POINT ( 'NONE',  ( -0.4591627418635558788, 1.414127833138721035, -3.910145517416460770 ) ) ;
#11865=CARTESIAN_POINT ( 'NONE',  ( -2.142213561789879428, 0.02617651024168221943, 0.4623158380715322036 ) ) ;
#11867=LINE ( 'NONE', #17772, #46636 ) ;
#11889=DIRECTION ( 'NONE',  ( 0.000000000000000000, 0.000000000000000000, -1.000000000000000000 ) ) ;
#11906=CYLINDRICAL_SURFACE ( 'NONE', #29173, 0.09842519685039351207 ) ;
#11917=SURFACE_STYLE_USAGE ( .BOTH. , #24527 ) ;
#11941=ADVANCED_FACE ( 'NONE', ( #2306 ), #30424, .F. ) ;
#11964=EDGE_CURVE ( 'NONE', #48318, #67810, #7363, .T. ) ;
#11975=CARTESIAN_POINT ( 'NONE',  ( -0.2771898661223743954, 1.152090366371692154, 1.087348617264907169 ) ) ;
#11993=DIRECTION ( 'NONE',  ( 0.000000000000000000, 1.000000000000000000, 0.000000000000000000 ) ) ;
#12003=ORIENTED_EDGE ( 'NONE', *, *, #21276, .T. ) ;
#12006=CARTESIAN_POINT ( 'NONE',  ( -2.154527559055123831, 0.03937007874015747977, 0.4677827689124697264 ) ) ;
#12012=DIRECTION ( 'NONE',  ( -0.000000000000000000, -1.000000000000000000, -8.673617379884024625E-16 ) ) ;
#12039=B_SPLINE_CURVE_WITH_KNOTS ( 'NONE', 3,
 ( #9529, #41100, #60037, #15439 ),
 .UNSPECIFIED., .F., .F.,
 ( 4, 4 ),
 ( 0.05078239113848836972, 0.05222574548756768464 ),
 .UNSPECIFIED. ) ;
#12050=B_SPLINE_CURVE_WITH_KNOTS ( 'NONE', 3,
 ( #62486, #4820, #30498, #56161 ),
 .UNSPECIFIED., .F., .F.,
 ( 4, 4 ),
 ( 1.009931976291010463E-06, 0.001444423380196054128 ),
 .UNSPECIFIED. ) ;
#12052=PLANE ( 'NONE',  #17062 ) ;
#12069=CARTESIAN_POINT ( 'NONE',  ( 0.4741706889230142830, 1.520077057622761574, 2.554855216661410910 ) ) ;
#12073=DIRECTION ( 'NONE',  ( -3.491481338843132961E-15, -0.000000000000000000, 1.000000000000000000 ) ) ;
#12083=ORIENTED_EDGE ( 'NONE', *, *, #52130, .T. ) ;
#12096=EDGE_LOOP ( 'NONE', ( #26023, #79408, #34061, #29889 ) ) ;
#12106=CARTESIAN_POINT ( 'NONE',  ( -1.559171609364246924, 0.3937007874015748254, 0.4177787735906735578 ) ) ;
#12117=ORIENTED_EDGE ( 'NONE', *, *, #46853, .T. ) ;
#12124=EDGE_CURVE ( 'NONE', #55951, #34868, #81815, .T. ) ;
#12134=ADVANCED_FACE ( 'NONE', ( #4773 ), #77544, .F. ) ;
#12143=ADVANCED_FACE ( 'NONE', ( #60780 ), #64067, .F. ) ;
#12144=CARTESIAN_POINT ( 'NONE',  ( 1.141392835773559211, 0.3937007874015748254, 0.8264322058523028147 ) ) ;
#12156=B_SPLINE_CURVE_WITH_KNOTS ( 'NONE', 3,
 ( #21634, #40578, #66259, #79315 ),
 .UNSPECIFIED., .F., .F.,
 ( 4, 4 ),
 ( 0.1818586053347995835, 0.1832800580269401680 ),
 .UNSPECIFIED. ) ;
#12168=CARTESIAN_POINT ( 'NONE',  ( 3.224202737261815166, 2.716535433070866645, -0.5314960629921260393 ) ) ;
#12171=CARTESIAN_POINT ( 'NONE',  ( 2.362204724409448620, 0.03937007874015751446, -0.5118110236220390075 ) ) ;
#12176=PLANE ( 'NONE',  #20287 ) ;
#12182=ADVANCED_FACE ( 'NONE', ( #48561 ), #7608, .F. ) ;
#12184=ORIENTED_EDGE ( 'NONE', *, *, #76206, .T. ) ;
#12186=EDGE_LOOP ( 'NONE', ( #63043, #81650, #52429, #62629 ) ) ;
#12196=B_SPLINE_CURVE_WITH_KNOTS ( 'NONE', 3,
 ( #39198, #21105, #27830, #28241 ),
 .UNSPECIFIED., .F., .F.,
 ( 4, 4 ),
 ( 0.07610408314619478143, 0.07753336624204336391 ),
 .UNSPECIFIED. ) ;
#12200=VERTEX_POINT ( 'NONE', #23306 ) ;
#12202=VERTEX_POINT ( 'NONE', #48976 ) ;
#12204=CARTESIAN_POINT ( 'NONE',  ( 0.9285414500055709786, 1.724409448818897905, -0.6299212598425196763 ) ) ;
#12235=CARTESIAN_POINT ( 'NONE',  ( -2.620897244026447304, 1.710976477253048245, -0.4417575354491495299 ) ) ;
#12238=CARTESIAN_POINT ( 'NONE',  ( -2.647175254740916639, 1.326002914239465147, -0.4256865378621351170 ) ) ;
#12253=DIRECTION ( 'NONE',  ( 1.000000000000000000, 0.000000000000000000, 3.455050906509825972E-15 ) ) ;
#12276=B_SPLINE_CURVE_WITH_KNOTS ( 'NONE', 3,
 ( #64905, #14827, #27430, #51413, #59007, #33754, #20293, #40487, #1362, #27014, #52676, #78383, #20714, #14417, #40070, #65757, #59416, #53091, #78803, #6404, #32074, #97, #2187, #34171, #81999, #2606, #30637, #27855, #28264, #41317, #79223, #8505, #28683, #79638, #53515, #62209, #81591, #34591, #30217, #24313, #47614, #73734, #17612, #49983, #55880, #62627, #4971, #21956 ),
 .UNSPECIFIED., .F., .F.,
 ( 4, 2, 2, 1, 2, 2, 2, 2, 2, 2, 2, 2, 2, 2, 2, 2, 2, 2, 2, 2, 2, 1, 2, 2, 4 ),
 ( 0.03770802486988159008, 0.04006421406960428144, 0.04124230866946564100, 0.04242040326932700056, 0.04359849786918835318, 0.04477659246904971274, 0.04713278166877243880, 0.04831087626863381224, 0.04948897086849517180, 0.05184516006821790479, 0.05302325466807927823, 0.05420134926794065167, 0.05655753846766339854, 0.05891372766738613848, 0.06009182226724750497, 0.06126991686710887841, 0.06362610606683162529, 0.06480420066669299872, 0.06598229526655435828, 0.06833848446627711903, 0.06951657906613849247, 0.07069467366599987979, 0.07187276826586125322, 0.07305086286572262666, 0.07540705206544537353 ),
 .UNSPECIFIED. ) ;
#12288=VECTOR ( 'NONE', #50504, 39.37007874015748143 ) ;
#12298=ORIENTED_EDGE ( 'NONE', *, *, #52130, .F. ) ;
#12317=ORIENTED_EDGE ( 'NONE', *, *, #69731, .T. ) ;
#12331=VECTOR ( 'NONE', #19551, 39.37007874015748143 ) ;
#12355=CARTESIAN_POINT ( 'NONE',  ( 2.563288228875796992, 1.597527518877483343, 0.4706608522957233531 ) ) ;
#12384=DIRECTION ( 'NONE',  ( 0.000000000000000000, 0.000000000000000000, 1.000000000000000000 ) ) ;
#12388=AXIS2_PLACEMENT_3D ( 'NONE', #56152, #10321, #49430 ) ;
#12418=DIRECTION ( 'NONE',  ( -0.000000000000000000, -1.000000000000000000, -0.000000000000000000 ) ) ;
#12420=DIRECTION ( 'NONE',  ( 0.000000000000000000, 0.000000000000000000, -1.000000000000000000 ) ) ;
#12431=CARTESIAN_POINT ( 'NONE',  ( 0.4177787735906999811, 1.312623414240995157, -1.714017618091133288 ) ) ;
#12436=CARTESIAN_POINT ( 'NONE',  ( -3.264097702071373064, 2.755905511811024056, -0.5314960629921260393 ) ) ;
#12441=VECTOR ( 'NONE', #62049, 39.37007874015749564 ) ;
#12458=CARTESIAN_POINT ( 'NONE',  ( 0.000000000000000000, 2.755905511811024056, 0.000000000000000000 ) ) ;
#12476=CARTESIAN_POINT ( 'NONE',  ( 0.4606233198248834704, 1.422786159591913568, 2.585446969423548680 ) ) ;
#12502=EDGE_CURVE ( 'NONE', #21089, #39954, #48151, .T. ) ;
#12515=CARTESIAN_POINT ( 'NONE',  ( 0.4744094488189065095, 1.537401574803149984, -2.554262525012259477 ) ) ;
#12517=CARTESIAN_POINT ( 'NONE',  ( 0.000000000000000000, 0.04488074079120789317, -1.244489337948954555 ) ) ;
#12524=ORIENTED_EDGE ( 'NONE', *, *, #24992, .F. ) ;
#12531=CARTESIAN_POINT ( 'NONE',  ( 2.169555354231010202, 1.520093187801265344, 0.4741711390158128703 ) ) ;
#12555=LINE ( 'NONE', #63889, #5013 ) ;
#12558=AXIS2_PLACEMENT_3D ( 'NONE', #11056, #79711, #22027 ) ;
#12564=CARTESIAN_POINT ( 'NONE',  ( 3.886287458032462006, 2.755905511811024056, -0.6299212598425196763 ) ) ;
#12572=CARTESIAN_POINT ( 'NONE',  ( -3.908320185825791437, 1.506315459106587040, 0.4744094488188971837 ) ) ;
#12577=CARTESIAN_POINT ( 'NONE',  ( -0.4580699644866061959, 1.664928367767637418, 1.024310904178314718 ) ) ;
#12580=CARTESIAN_POINT ( 'NONE',  ( 1.403614904275686858E-14, 1.537401574803149984, -3.937007874015761910 ) ) ;
#12586=CARTESIAN_POINT ( 'NONE',  ( 0.4177787735907000366, 1.299212598425196985, -1.559171609364239375 ) ) ;
#12593=VERTEX_POINT ( 'NONE', #55283 ) ;
#12595=ORIENTED_EDGE ( 'NONE', *, *, #57238, .F. ) ;
#12600=AXIS2_PLACEMENT_3D ( 'NONE', #15907, #47444, #41556 ) ;
#12610=ORIENTED_EDGE ( 'NONE', *, *, #51722, .F. ) ;
#12614=CARTESIAN_POINT ( 'NONE',  ( 2.808244076867902450, 1.134815007188468838, -0.2514610820057333607 ) ) ;
#12618=AXIS2_PLACEMENT_3D ( 'NONE', #67291, #62617, #55868 ) ;
#12663=EDGE_CURVE ( 'NONE', #23658, #62570, #6506, .T. ) ;
#12675=AXIS2_PLACEMENT_3D ( 'NONE', #38369, #62391, #62817 ) ;
#12709=LINE ( 'NONE', #75455, #5874 ) ;
#12714=VERTEX_POINT ( 'NONE', #30858 ) ;
#12722=CIRCLE ( 'NONE', #59763, 0.5118110236220471121 ) ;
#12726=CARTESIAN_POINT ( 'NONE',  ( 1.141392835773559211, 1.299212598425196985, 1.141392835773562764 ) ) ;
#12729=ORIENTED_EDGE ( 'NONE', *, *, #47818, .T. ) ;
#12739=VECTOR ( 'NONE', #1130, 39.37007874015748143 ) ;
#12757=DIRECTION ( 'NONE',  ( -0.000000000000000000, -1.000000000000000000, -0.000000000000000000 ) ) ;
#12761=ADVANCED_FACE ( 'NONE', ( #56933 ), #37178, .F. ) ;
#12763=CARTESIAN_POINT ( 'NONE',  ( -1.559171609364246924, 0.3937007874015747699, 0.2199441279213821265 ) ) ;
#12771=CARTESIAN_POINT ( 'NONE',  ( -1.313877454013331780, 1.062992125984252079, 0.7983292792091805090 ) ) ;
#12780=PLANE ( 'NONE',  #22503 ) ;
#12798=AXIS2_PLACEMENT_3D ( 'NONE', #44862, #25520, #79397 ) ;
#12813=DIRECTION ( 'NONE',  ( -0.000000000000000000, -1.000000000000000000, -0.000000000000000000 ) ) ;
#12836=PLANE ( 'NONE',  #74752 ) ;
#12837=DIRECTION ( 'NONE',  ( 0.000000000000000000, 1.000000000000000000, 0.000000000000000000 ) ) ;
#12846=DIRECTION ( 'NONE',  ( 0.000000000000000000, -1.000000000000000000, 0.000000000000000000 ) ) ;
#12855=DIRECTION ( 'NONE',  ( -0.000000000000000000, -1.000000000000000000, -0.000000000000000000 ) ) ;
#12909=ORIENTED_EDGE ( 'NONE', *, *, #30460, .T. ) ;
#12935=B_SPLINE_CURVE_WITH_KNOTS ( 'NONE', 3,
 ( #66013, #14262, #2456, #59265, #52525, #33189, #8350, #53363, #78231, #39920, #20565, #66848 ),
 .UNSPECIFIED., .F., .F.,
 ( 4, 2, 2, 2, 2, 4 ),
 ( 0.04729187226826446488, 0.04795755069747583560, 0.04862322912668719938, 0.04995458598510991305, 0.05128594284353263366, 0.05261729970195534734 ),
 .UNSPECIFIED. ) ;
#12943=CARTESIAN_POINT ( 'NONE',  ( 0.5314960629921393620, 2.755905511811024056, -3.821484228344191880 ) ) ;
#12944=ORIENTED_EDGE ( 'NONE', *, *, #82633, .T. ) ;
#12951=CARTESIAN_POINT ( 'NONE',  ( 2.170146923806594685, 1.528804020127597640, 0.4744094488188974612 ) ) ;
#12953=DIRECTION ( 'NONE',  ( -3.491481338843133355E-15, -0.000000000000000000, 1.000000000000000000 ) ) ;
#12965=CARTESIAN_POINT ( 'NONE',  ( -0.1092078379430496404, 1.075719315424584543, -1.514693649293256117 ) ) ;
#13007=EDGE_CURVE ( 'NONE', #25136, #58442, #83040, .T. ) ;
#13011=AXIS2_PLACEMENT_3D ( 'NONE', #63673, #53538, #52284 ) ;
#13012=AXIS2_PLACEMENT_3D ( 'NONE', #54652, #54233, #22263 ) ;
#13015=ORIENTED_EDGE ( 'NONE', *, *, #50027, .F. ) ;
#13017=VERTEX_POINT ( 'NONE', #31685 ) ;
#13075=AXIS2_PLACEMENT_3D ( 'NONE', #48356, #74054, #30245 ) ;
#13087=EDGE_CURVE ( 'NONE', #24482, #66439, #24541, .T. ) ;
#13095=FACE_OUTER_BOUND ( 'NONE', #35506, .T. ) ;
#13113=B_SPLINE_CURVE_WITH_KNOTS ( 'NONE', 3,
 ( #2750, #75830, #21682, #41045 ),
 .UNSPECIFIED., .F., .F.,
 ( 4, 4 ),
 ( 0.06998245282297338443, 0.07142600748853988879 ),
 .UNSPECIFIED. ) ;
#13121=EDGE_CURVE ( 'NONE', #8593, #5432, #42563, .T. ) ;
#13124=DIRECTION ( 'NONE',  ( 0.000000000000000000, 0.000000000000000000, -1.000000000000000000 ) ) ;
#13126=CARTESIAN_POINT ( 'NONE',  ( 0.4177787735907000366, 0.3937007874015747699, -1.559171609364239375 ) ) ;
#13135=CARTESIAN_POINT ( 'NONE',  ( -0.4117837489889357716, 1.301386200251876124, -2.058030895701184804 ) ) ;
#13136=ORIENTED_EDGE ( 'NONE', *, *, #27456, .T. ) ;
#13153=CARTESIAN_POINT ( 'NONE',  ( -0.5314960629921394730, 2.736617272820978108, 3.873860110281695412 ) ) ;
#13155=DIRECTION ( 'NONE',  ( 0.000000000000000000, -1.000000000000000000, 0.000000000000000000 ) ) ;
#13157=EDGE_LOOP ( 'NONE', ( #41189, #28473, #58016, #54435 ) ) ;
#13163=CARTESIAN_POINT ( 'NONE',  ( 3.937007874015748143, 1.537401574803149984, 0.4744094488188975722 ) ) ;
#13174=CARTESIAN_POINT ( 'NONE',  ( 0.000000000000000000, 2.755905511811024056, 0.000000000000000000 ) ) ;
#13182=CARTESIAN_POINT ( 'NONE',  ( -0.3334193678581739984, 1.199601195606727844, 1.973660451468200350 ) ) ;
#13185=EDGE_CURVE ( 'NONE', #66439, #51179, #8994, .T. ) ;
#13194=ADVANCED_FACE ( 'NONE', ( #2212 ), #39249, .F. ) ;
#13197=AXIS2_PLACEMENT_3D ( 'NONE', #83272, #30265, #57581 ) ;
#13211=B_SPLINE_CURVE_WITH_KNOTS ( 'NONE', 3,
 ( #17415, #48539, #9839, #30012 ),
 .UNSPECIFIED., .F., .F.,
 ( 4, 4 ),
 ( 0.1191888912451262300, 0.1206125572960974335 ),
 .UNSPECIFIED. ) ;
#13237=ADVANCED_FACE ( 'NONE', ( #26630 ), #46586, .T. ) ;
#13252=VERTEX_POINT ( 'NONE', #71666 ) ;
#13254=VERTEX_POINT ( 'NONE', #20740 ) ;
#13259=CARTESIAN_POINT ( 'NONE',  ( 2.362204724409448620, 1.929133858267716661, 8.247593713802677664E-15 ) ) ;
#13268=CARTESIAN_POINT ( 'NONE',  ( -1.116861235539043928, 1.075383049963962279, -0.1088361571701338959 ) ) ;
#13314=CARTESIAN_POINT ( 'NONE',  ( 1.348312163386739426, 0.2755905511811023723, 0.8371118098809627872 ) ) ;
#13326=ORIENTED_EDGE ( 'NONE', *, *, #56357, .T. ) ;
#13333=CARTESIAN_POINT ( 'NONE',  ( 0.000000000000000000, 1.724409448818897905, 0.000000000000000000 ) ) ;
#13342=EDGE_LOOP ( 'NONE', ( #70918, #67919, #78918, #48210 ) ) ;
#13343=LINE ( 'NONE', #32687, #32780 ) ;
#13349=VECTOR ( 'NONE', #58792, 39.37007874015748143 ) ;
#13350=DIRECTION ( 'NONE',  ( -0.000000000000000000, -1.000000000000000000, -0.000000000000000000 ) ) ;
#13360=ORIENTED_EDGE ( 'NONE', *, *, #67540, .F. ) ;
#13367=DIRECTION ( 'NONE',  ( 0.000000000000000000, 0.000000000000000000, -1.000000000000000000 ) ) ;
#13400=LINE ( 'NONE', #12564, #64996 ) ;
#13408=CARTESIAN_POINT ( 'NONE',  ( -3.915497197276881280, 1.300040739893603359, -0.4110563714168837257 ) ) ;
#13414=ORIENTED_EDGE ( 'NONE', *, *, #25974, .F. ) ;
#13428=ORIENTED_EDGE ( 'NONE', *, *, #6791, .T. ) ;
#13430=ORIENTED_EDGE ( 'NONE', *, *, #40727, .T. ) ;
#13446=ORIENTED_EDGE ( 'NONE', *, *, #70713, .F. ) ;
#13459=CARTESIAN_POINT ( 'NONE',  ( -2.558921551581103682, 1.580736828574225594, 0.4725026149319433433 ) ) ;
#13476=DIRECTION ( 'NONE',  ( -3.491481338843132961E-15, -0.000000000000000000, 1.000000000000000000 ) ) ;
#13479=CARTESIAN_POINT ( 'NONE',  ( 3.197598474799423496, 2.742783277647742324, 0.5314960629921260393 ) ) ;
#13485=EDGE_CURVE ( 'NONE', #44548, #7361, #74807, .T. ) ;
#13503=CARTESIAN_POINT ( 'NONE',  ( 0.000000000000000000, 0.03937007874015751446, -2.362204724409448620 ) ) ;
#13508=DIRECTION ( 'NONE',  ( 0.000000000000000000, 0.000000000000000000, -1.000000000000000000 ) ) ;
#13517=DIRECTION ( 'NONE',  ( 1.000000000000000000, -0.000000000000000000, -0.000000000000000000 ) ) ;
#13535=DIRECTION ( 'NONE',  ( 1.000000000000000000, -0.000000000000000000, -0.000000000000000000 ) ) ;
#13546=ORIENTED_EDGE ( 'NONE', *, *, #8916, .F. ) ;
#13549=EDGE_LOOP ( 'NONE', ( #81596, #34769, #54072, #38979 ) ) ;
#13567=VERTEX_POINT ( 'NONE', #67432 ) ;
#13569=ORIENTED_EDGE ( 'NONE', *, *, #57395, .T. ) ;
#13599=CARTESIAN_POINT ( 'NONE',  ( -0.9285414500055708675, 1.724409448818898127, -0.6299212598425202314 ) ) ;
#13621=AXIS2_PLACEMENT_3D ( 'NONE', #65768, #7688, #71235 ) ;
#13645=CARTESIAN_POINT ( 'NONE',  ( -0.4697243008124643016, 1.606021484273580935, -2.158901635429134380 ) ) ;
#13659=AXIS2_PLACEMENT_3D ( 'NONE', #26280, #51941, #64179 ) ;
#13664=EDGE_CURVE ( 'NONE', #64696, #15345, #51655, .T. ) ;
#13667=ORIENTED_EDGE ( 'NONE', *, *, #40392, .F. ) ;
#13670=DIRECTION ( 'NONE',  ( 0.000000000000000000, 0.000000000000000000, -1.000000000000000000 ) ) ;
#13717=ADVANCED_FACE ( 'NONE', ( #19983 ), #45633, .F. ) ;
#13729=DIRECTION ( 'NONE',  ( 0.000000000000000000, 0.000000000000000000, -1.000000000000000000 ) ) ;
#13734=CARTESIAN_POINT ( 'NONE',  ( 1.017216587056826160, 1.569965579892641738, 0.4735649329124862472 ) ) ;
#13746=ORIENTED_EDGE ( 'NONE', *, *, #14676, .F. ) ;
#13747=ORIENTED_EDGE ( 'NONE', *, *, #79456, .T. ) ;
#13774=DIRECTION ( 'NONE',  ( -1.000000000000000000, -0.000000000000000000, -0.000000000000000000 ) ) ;
#13781=EDGE_LOOP ( 'NONE', ( #58003, #26326, #69661, #11364 ) ) ;
#13784=CIRCLE ( 'NONE', #52746, 0.1771653543307085410 ) ;
#13788=CARTESIAN_POINT ( 'NONE',  ( 0.000000000000000000, 1.724409448818897461, 0.000000000000000000 ) ) ;
#13796=DIRECTION ( 'NONE',  ( 9.381338752702759131E-17, -0.6427876096865364763, 0.7660444431189804559 ) ) ;
#13813=ADVANCED_FACE ( 'NONE', ( #52782 ), #78491, .F. ) ;
#13821=CARTESIAN_POINT ( 'NONE',  ( -2.543486866223389153, 2.716535433070866645, -0.5314960629921260393 ) ) ;
#13830=CYLINDRICAL_SURFACE ( 'NONE', #62758, 0.4744094488188972947 ) ;
#13837=VERTEX_POINT ( 'NONE', #83235 ) ;
#13850=ORIENTED_EDGE ( 'NONE', *, *, #34274, .T. ) ;
#13866=ORIENTED_EDGE ( 'NONE', *, *, #4866, .F. ) ;
#13869=CARTESIAN_POINT ( 'NONE',  ( 2.759487654322811956, 1.189595890467133987, -0.3229789317950513272 ) ) ;
#13882=CARTESIAN_POINT ( 'NONE',  ( 0.000000000000000000, 0.000000000000000000, -1.289370078740159409 ) ) ;
#13897=CIRCLE ( 'NONE', #67668, 0.09842519685039351207 ) ;
#13904=CARTESIAN_POINT ( 'NONE',  ( -2.554262525012342966, 1.537401574803149984, -0.4744094488188975722 ) ) ;
#13912=DIRECTION ( 'NONE',  ( 0.000000000000000000, -0.5150380749100564870, -0.8571673007021107793 ) ) ;
#13935=CARTESIAN_POINT ( 'NONE',  ( 1.895394334970792016, 2.755905511811024056, 0.5314960629921260393 ) ) ;
#13944=CARTESIAN_POINT ( 'NONE',  ( 3.886287458032462006, 1.724409448818898127, 0.6299212598425202314 ) ) ;
#13957=ORIENTED_EDGE ( 'NONE', *, *, #57885, .T. ) ;
#13975=ORIENTED_EDGE ( 'NONE', *, *, #5896, .T. ) ;
#13989=CARTESIAN_POINT ( 'NONE',  ( -0.4744094488188832504, 1.537401574803149984, -3.937007874015763687 ) ) ;
#13991=CARTESIAN_POINT ( 'NONE',  ( 1.141392835773559211, 0.3937007874015748254, 1.141392835773562764 ) ) ;
#13996=CARTESIAN_POINT ( 'NONE',  ( -2.583694225513480713, 2.755905511811024056, -0.5314960629921260393 ) ) ;
#14003=VECTOR ( 'NONE', #77498, 39.37007874015748143 ) ;
#14017=CARTESIAN_POINT ( 'NONE',  ( 0.5314960629920925106, 2.742783273398276656, 3.197598479107681690 ) ) ;
#14018=DIRECTION ( 'NONE',  ( 1.000000000000000000, -0.000000000000000000, -0.000000000000000000 ) ) ;
#14029=CARTESIAN_POINT ( 'NONE',  ( 1.023944627548813768, 1.412952001865432239, -0.4588836347674642990 ) ) ;
#14043=ADVANCED_FACE ( 'NONE', ( #77764 ), #18447, .F. ) ;
#14047=EDGE_CURVE ( 'NONE', #64696, #712, #61293, .T. ) ;
#14051=DIRECTION ( 'NONE',  ( 0.000000000000000000, -1.387778780781445676E-15, -1.000000000000000000 ) ) ;
#14058=AXIS2_PLACEMENT_3D ( 'NONE', #9859, #60779, #8618 ) ;
#14094=CARTESIAN_POINT ( 'NONE',  ( -0.4744094488189057879, 1.528788477448867367, 2.554262525012262142 ) ) ;
#14095=DIRECTION ( 'NONE',  ( -0.000000000000000000, -1.000000000000000000, -0.000000000000000000 ) ) ;
#14103=CARTESIAN_POINT ( 'NONE',  ( -1.016821367227983108, 1.506045768764721515, -0.4744094488188973502 ) ) ;
#14105=LINE ( 'NONE', #39757, #69388 ) ;
#14106=CARTESIAN_POINT ( 'NONE',  ( -3.937007874015748143, 2.755905511811024056, 0.5314960629921260393 ) ) ;
#14134=AXIS2_PLACEMENT_3D ( 'NONE', #21736, #60863, #2805 ) ;
#14144=ORIENTED_EDGE ( 'NONE', *, *, #21499, .F. ) ;
#14158=CARTESIAN_POINT ( 'NONE',  ( 0.4725026149319347391, 1.580736828574228703, 2.558921551581183174 ) ) ;
#14170=ORIENTED_EDGE ( 'NONE', *, *, #75948, .T. ) ;
#14176=FACE_OUTER_BOUND ( 'NONE', #30818, .T. ) ;
#14187=VERTEX_POINT ( 'NONE', #56217 ) ;
#14197=DIRECTION ( 'NONE',  ( 0.000000000000000000, -0.5150380749100561539, -0.8571673007021108903 ) ) ;
#14212=CARTESIAN_POINT ( 'NONE',  ( 2.153082335389886026, 1.453547212638085062, 0.4672029448317644440 ) ) ;
#14220=CARTESIAN_POINT ( 'NONE',  ( -0.5314960629921373636, 2.742781055772889331, 3.250800393950209699 ) ) ;
#14243=DIRECTION ( 'NONE',  ( 0.000000000000000000, -1.000000000000000000, 0.000000000000000000 ) ) ;
#14252=VECTOR ( 'NONE', #41812, 39.37007874015748143 ) ;
#14262=CARTESIAN_POINT ( 'NONE',  ( 0.4744094488189063985, 1.546135192374304523, -2.554262525012259033 ) ) ;
#14270=CARTESIAN_POINT ( 'NONE',  ( 0.4494645459842863122, 1.384795284186596254, -3.911270042648091305 ) ) ;
#14276=ORIENTED_EDGE ( 'NONE', *, *, #61363, .T. ) ;
#14288=ORIENTED_EDGE ( 'NONE', *, *, #11333, .F. ) ;
#14290=CONICAL_SURFACE ( 'NONE', #7550, 0.1978346456692914035, 0.8726646259971700959 ) ;
#14291=ORIENTED_EDGE ( 'NONE', *, *, #54265, .F. ) ;
#14294=AXIS2_PLACEMENT_3D ( 'NONE', #24136, #81410, #23727 ) ;
#14296=CARTESIAN_POINT ( 'NONE',  ( -1.531218781212690727, 1.129506115079992101, 0.2422809976808260046 ) ) ;
#14300=EDGE_CURVE ( 'NONE', #9114, #59294, #10387, .T. ) ;
#14303=PLANE ( 'NONE',  #11656 ) ;
#14314=B_SPLINE_CURVE_WITH_KNOTS ( 'NONE', 3,
 ( #26298, #39340, #57446, #65027 ),
 .UNSPECIFIED., .F., .F.,
 ( 4, 4 ),
 ( 0.07138240964905806507, 0.07282471043319424520 ),
 .UNSPECIFIED. ) ;
#14348=CARTESIAN_POINT ( 'NONE',  ( 0.03416814150274168765, 1.063911309852949794, -1.851246078702575959 ) ) ;
#14370=FACE_OUTER_BOUND ( 'NONE', #3226, .T. ) ;
#14371=CARTESIAN_POINT ( 'NONE',  ( 0.000000000000000000, 2.755905511811024056, 0.000000000000000000 ) ) ;
#14387=CARTESIAN_POINT ( 'NONE',  ( -0.4359958488159628165, 1.724409448818897905, -2.630268417803939940 ) ) ;
#14394=EDGE_CURVE ( 'NONE', #53376, #51564, #10320, .T. ) ;
#14412=LINE ( 'NONE', #20286, #53021 ) ;
#14414=DIRECTION ( 'NONE',  ( 0.000000000000000000, -1.000000000000000000, 0.000000000000000000 ) ) ;
#14417=CARTESIAN_POINT ( 'NONE',  ( 3.924543106786416935, 1.180793272576371677, -0.3132714499646157003 ) ) ;
#14418=AXIS2_PLACEMENT_3D ( 'NONE', #47530, #66494, #79552 ) ;
#14421=AXIS2_PLACEMENT_3D ( 'NONE', #35503, #73821, #48949 ) ;
#14444=FACE_OUTER_BOUND ( 'NONE', #43248, .T. ) ;
#14490=CARTESIAN_POINT ( 'NONE',  ( -1.559171609364246924, 0.000000000000000000, 0.4177787735906735578 ) ) ;
#14514=CARTESIAN_POINT ( 'NONE',  ( -0.4698793137518578189, 1.469922167998565676, 2.565145773722669720 ) ) ;
#14550=CARTESIAN_POINT ( 'NONE',  ( 2.530077748780002800, 2.729661042438510155, 0.5314960629921260393 ) ) ;
#14563=FACE_OUTER_BOUND ( 'NONE', #79729, .T. ) ;
#14565=ORIENTED_EDGE ( 'NONE', *, *, #11099, .F. ) ;
#14604=ORIENTED_EDGE ( 'NONE', *, *, #5896, .F. ) ;
#14629=CARTESIAN_POINT ( 'NONE',  ( 2.159244633716622008, 1.469861850861822639, -0.4698711669589714646 ) ) ;
#14653=CARTESIAN_POINT ( 'NONE',  ( 0.4479262672266381418, 1.381097145630199030, -1.587474637006627276 ) ) ;
#14676=EDGE_CURVE ( 'NONE', #29189, #27377, #70760, .T. ) ;
#14677=CARTESIAN_POINT ( 'NONE',  ( -3.821484228344193657, 2.755905511811024056, -0.5314960629921260393 ) ) ;
#14682=DIRECTION ( 'NONE',  ( -0.000000000000000000, -1.000000000000000000, 8.673617379884024625E-16 ) ) ;
#14688=VECTOR ( 'NONE', #14197, 39.37007874015748854 ) ;
#14690=ORIENTED_EDGE ( 'NONE', *, *, #15825, .F. ) ;
#14706=EDGE_LOOP ( 'NONE', ( #45487, #73905, #13746, #44416, #61695, #47509 ) ) ;
#14711=CARTESIAN_POINT ( 'NONE',  ( 2.619510771202491206, 1.365902157108384696, 0.4425616331406697634 ) ) ;
#14716=EDGE_CURVE ( 'NONE', #19641, #33945, #68112, .T. ) ;
#14729=EDGE_CURVE ( 'NONE', #37337, #59692, #26524, .T. ) ;
#14751=CARTESIAN_POINT ( 'NONE',  ( -0.5314960629921127166, 2.755905511811024056, -3.821484228344195433 ) ) ;
#14776=EDGE_LOOP ( 'NONE', ( #71085, #23283, #68737, #39508 ) ) ;
#14780=DIRECTION ( 'NONE',  ( 0.000000000000000000, 1.000000000000000000, 0.000000000000000000 ) ) ;
#14790=ORIENTED_EDGE ( 'NONE', *, *, #58775, .F. ) ;
#14793=ORIENTED_EDGE ( 'NONE', *, *, #18368, .F. ) ;
#14799=CARTESIAN_POINT ( 'NONE',  ( 0.05682587177516690985, 1.066401174101865301, -1.556166698229688228 ) ) ;
#14811=ORIENTED_EDGE ( 'NONE', *, *, #76605, .F. ) ;
#14827=CARTESIAN_POINT ( 'NONE',  ( 3.908320185825792770, 1.506432478651347662, -0.4744094488188970171 ) ) ;
#14830=CARTESIAN_POINT ( 'NONE',  ( -0.4498537592782897998, 0.000000000000000000, 2.118110236220472675 ) ) ;
#14843=CARTESIAN_POINT ( 'NONE',  ( 1.374111566022513293E-16, 1.062992125984252745, -1.122047244094488194 ) ) ;
#14850=CARTESIAN_POINT ( 'NONE',  ( -0.4623158380715545746, 0.02617651024168222984, -2.142213561789874543 ) ) ;
#14876=VECTOR ( 'NONE', #5174, 39.37007874015748143 ) ;
#14887=CARTESIAN_POINT ( 'NONE',  ( 3.892860353355074299, 2.712196231959916659, -0.5314960629921260393 ) ) ;
#14896=CARTESIAN_POINT ( 'NONE',  ( 0.03176189650790594426, 1.062992125984252301, 1.122047244094488194 ) ) ;
#14920=DIRECTION ( 'NONE',  ( -3.491481338843132961E-15, -0.000000000000000000, 1.000000000000000000 ) ) ;
#14923=CARTESIAN_POINT ( 'NONE',  ( 0.4575346093745696896, 1.663833025909975172, -3.910334573579572037 ) ) ;
#14927=VECTOR ( 'NONE', #46567, 39.37007874015748143 ) ;
#14929=DIRECTION ( 'NONE',  ( 0.000000000000000000, -1.000000000000000000, 0.000000000000000000 ) ) ;
#14936=ORIENTED_EDGE ( 'NONE', *, *, #30614, .F. ) ;
#14938=CARTESIAN_POINT ( 'NONE',  ( 1.141392835773559211, 0.3937007874015747699, 1.141392835773562764 ) ) ;
#14945=DIRECTION ( 'NONE',  ( 0.000000000000000000, 0.000000000000000000, -1.000000000000000000 ) ) ;
#14949=VECTOR ( 'NONE', #16026, 39.37007874015748143 ) ;
#14970=ORIENTED_EDGE ( 'NONE', *, *, #8199, .T. ) ;
#14986=( GEOMETRIC_REPRESENTATION_CONTEXT ( 3 ) GLOBAL_UNCERTAINTY_ASSIGNED_CONTEXT ( ( #73122 ) ) GLOBAL_UNIT_ASSIGNED_CONTEXT ( ( #36337, #37571, #63245 ) ) REPRESENTATION_CONTEXT ( 'NONE', 'WORKASPACE' ) );
#14989=B_SPLINE_CURVE_WITH_KNOTS ( 'NONE', 3,
 ( #63853, #57110, #57528, #81587 ),
 .UNSPECIFIED., .F., .F.,
 ( 4, 4 ),
 ( 0.1000642744325473399, 0.1014879310549286484 ),
 .UNSPECIFIED. ) ;
#15017=CARTESIAN_POINT ( 'NONE',  ( -1.580526701345955409, 1.383198989551510216, 0.4486511340363580902 ) ) ;
#15031=CARTESIAN_POINT ( 'NONE',  ( 0.5314960629921395840, 2.748002881374839834, -3.856579543051779524 ) ) ;
#15038=CARTESIAN_POINT ( 'NONE',  ( 2.104898677616436231, 1.365902157108388248, -0.4425616331406706516 ) ) ;
#15061=CARTESIAN_POINT ( 'NONE',  ( 0.4469741871781334752, 1.378378501333950679, -1.594259055605391939 ) ) ;
#15063=DIRECTION ( 'NONE',  ( 1.047444401652940007E-14, -0.000000000000000000, -1.000000000000000000 ) ) ;
#15083=PLANE ( 'NONE',  #40519 ) ;
#15084=ADVANCED_FACE ( 'NONE', ( #82934 ), #73586, .F. ) ;
#15090=EDGE_CURVE ( 'NONE', #53614, #19971, #15477, .T. ) ;
#15093=CARTESIAN_POINT ( 'NONE',  ( 0.000000000000000000, 2.165354330708661568, 0.000000000000000000 ) ) ;
#15096=ORIENTED_EDGE ( 'NONE', *, *, #75806, .T. ) ;
#15098=VERTEX_POINT ( 'NONE', #33260 ) ;
#15109=CONICAL_SURFACE ( 'NONE', #24451, 1.968503937007874072, 0.7853981633974500554 ) ;
#15112=ADVANCED_FACE ( 'NONE', ( #18951 ), #66858, .T. ) ;
#15115=ORIENTED_EDGE ( 'NONE', *, *, #58440, .T. ) ;
#15126=CARTESIAN_POINT ( 'NONE',  ( -2.630268417803964809, 1.724409448818898127, -0.4359958488159723089 ) ) ;
#15158=CARTESIAN_POINT ( 'NONE',  ( -0.5314960629921123836, 2.729333734409945311, -3.881246834694717762 ) ) ;
#15160=EDGE_CURVE ( 'NONE', #64866, #59983, #26091, .T. ) ;
#15165=VECTOR ( 'NONE', #29234, 39.37007874015748143 ) ;
#15209=CARTESIAN_POINT ( 'NONE',  ( -0.4724973665168013537, 1.580780302271974636, -2.558933905385162078 ) ) ;
#15250=CARTESIAN_POINT ( 'NONE',  ( 0.5314960629921346991, 2.755905511811024056, -2.503252890251014495 ) ) ;
#15258=CARTESIAN_POINT ( 'NONE',  ( -0.2898037569319622531, 1.161479134785472045, -1.084046850253320926 ) ) ;
#15271=AXIS2_PLACEMENT_3D ( 'NONE', #47858, #9992, #53348 ) ;
#15277=DIRECTION ( 'NONE',  ( 0.000000000000000000, 0.000000000000000000, -1.000000000000000000 ) ) ;
#15285=CIRCLE ( 'NONE', #47523, 3.937007874015748143 ) ;
#15302=LINE ( 'NONE', #42194, #31850 ) ;
#15311=CARTESIAN_POINT ( 'NONE',  ( 0.1539941091832136288, 1.088406432939548640, 1.111532584200361606 ) ) ;
#15323=VECTOR ( 'NONE', #9937, 39.37007874015749564 ) ;
#15330=ORIENTED_EDGE ( 'NONE', *, *, #8460, .F. ) ;
#15335=DIRECTION ( 'NONE',  ( -0.000000000000000000, -1.000000000000000000, -0.000000000000000000 ) ) ;
#15336=CARTESIAN_POINT ( 'NONE',  ( 0.000000000000000000, 2.755905511811024056, 0.000000000000000000 ) ) ;
#15339=EDGE_CURVE ( 'NONE', #15857, #20906, #39989, .T. ) ;
#15342=CARTESIAN_POINT ( 'NONE',  ( 0.4479248917284270881, 1.694519753174063892, -3.911447006860421016 ) ) ;
#15345=VERTEX_POINT ( 'NONE', #44598 ) ;
#15348=CARTESIAN_POINT ( 'NONE',  ( 0.000000000000000000, 2.755905511811024056, 0.000000000000000000 ) ) ;
#15349=FACE_OUTER_BOUND ( 'NONE', #20817, .T. ) ;
#15355=FACE_OUTER_BOUND ( 'NONE', #71733, .T. ) ;
#15362=CARTESIAN_POINT ( 'NONE',  ( 0.000000000000000000, 2.755905511811024056, 0.000000000000000000 ) ) ;
#15380=CARTESIAN_POINT ( 'NONE',  ( 0.4177787735907000366, 0.3937007874015748254, -1.382006255033530806 ) ) ;
#15383=DIRECTION ( 'NONE',  ( -0.000000000000000000, 1.000000000000000000, -0.000000000000000000 ) ) ;
#15398=CIRCLE ( 'NONE', #59717, 0.07874015748031502893 ) ;
#15401=LINE ( 'NONE', #60826, #68179 ) ;
#15402=APPLICATION_CONTEXT ( 'automotive_design' ) ;
#15439=CARTESIAN_POINT ( 'NONE',  ( 1.813482582612293559, 2.755905511811024056, -0.5314960629921260393 ) ) ;
#15443=EDGE_CURVE ( 'NONE', #51179, #31528, #53604, .T. ) ;
#15454=LENGTH_MEASURE_WITH_UNIT ( LENGTH_MEASURE( 0.02539999999999999897 ), #27231 );
#15456=DIRECTION ( 'NONE',  ( 1.000000000000000000, -0.000000000000000000, -0.000000000000000000 ) ) ;
#15466=AXIS2_PLACEMENT_3D ( 'NONE', #75989, #43558, #69668 ) ;
#15477=B_SPLINE_CURVE_WITH_KNOTS ( 'NONE', 3,
 ( #4667, #16920, #50103, #74575, #24842, #5091, #81717, #68261, #24027, #31160, #43365, #42557, #76213, #74988, #5905, #75800, #69479, #17333, #10597, #81302, #36655, #31577, #30340, #61923, #18142, #55590, #56827, #37894, #44194, #36253, #68657, #30759, #43776, #4264, #42963, #82524, #11832, #10995, #29927, #23616, #56006, #50509, #49285, #62330, #37485, #18549, #69884, #49695, #12238, #75390, #69065, #11415, #37070, #62755, #63159, #63570, #71977, #7158, #32829, #13904 ),
 .UNSPECIFIED., .F., .F.,
 ( 4, 2, 2, 2, 2, 2, 2, 2, 2, 2, 2, 2, 2, 2, 2, 2, 2, 2, 2, 2, 2, 2, 2, 2, 2, 2, 2, 2, 2, 4 ),
 ( 0.01323639539072430336, 0.01388181161316797210, 0.01452722783561164084, 0.01581806028049896964, 0.01710889272538629671, 0.01839972517027362378, 0.02098139006004827098, 0.02356305494982292165, 0.02485388739471023484, 0.02614471983959755497, 0.02743555228448487163, 0.02872638472937218829, 0.03130804961914681467, 0.03259888206403412786, 0.03388971450892144105, 0.03453513073136509071, 0.03518054695380875424, 0.03647137939869606049, 0.03776221184358337368, 0.03905304428847067993, 0.04034387673335799313, 0.04163470917824529938, 0.04421637406801992576, 0.04679803895779455908, 0.04937970384756918546, 0.05067053629245649865, 0.05196136873734381184, 0.05325220118223111809, 0.05389761740467478163, 0.05454303362711843822 ),
 .UNSPECIFIED. ) ;
#15501=CARTESIAN_POINT ( 'NONE',  ( -3.881211926161857395, 2.729373344522950884, -0.5314960629921260393 ) ) ;
#15512=VECTOR ( 'NONE', #82304, 39.37007874015748143 ) ;
#15514=VERTEX_POINT ( 'NONE', #6736 ) ;
#15517=ORIENTED_EDGE ( 'NONE', *, *, #64730, .T. ) ;
#15536=CARTESIAN_POINT ( 'NONE',  ( 0.000000000000000000, 2.755905511811024056, 0.000000000000000000 ) ) ;
#15543=CARTESIAN_POINT ( 'NONE',  ( 0.4573980430285805587, 1.664306849931878274, 1.024599542107852423 ) ) ;
#15548=ORIENTED_EDGE ( 'NONE', *, *, #33485, .T. ) ;
#15550=FACE_OUTER_BOUND ( 'NONE', #23579, .T. ) ;
#15551=ORIENTED_EDGE ( 'NONE', *, *, #64058, .T. ) ;
#15570=EDGE_CURVE ( 'NONE', #32472, #22014, #71555, .T. ) ;
#15572=CARTESIAN_POINT ( 'NONE',  ( -1.559171609364246924, 0.3937007874015748254, 0.1028181436694137613 ) ) ;
#15578=CARTESIAN_POINT ( 'NONE',  ( -2.165589143934456118, 1.494558157769223961, -0.4725443725032424380 ) ) ;
#15604=ORIENTED_EDGE ( 'NONE', *, *, #73594, .T. ) ;
#15607=EDGE_CURVE ( 'NONE', #77755, #21629, #45017, .T. ) ;
#15634=CARTESIAN_POINT ( 'NONE',  ( 0.000000000000000000, 2.165354330708661568, 0.000000000000000000 ) ) ;
#15640=ORIENTED_EDGE ( 'NONE', *, *, #8676, .T. ) ;
#15642=CIRCLE ( 'NONE', #30381, 1.122047244094488194 ) ;
#15667=FACE_OUTER_BOUND ( 'NONE', #60361, .T. ) ;
#15675=CARTESIAN_POINT ( 'NONE',  ( -0.3136911643361884883, 1.181168853316014955, -1.077377206225114126 ) ) ;
#15695=AXIS2_PLACEMENT_3D ( 'NONE', #7044, #71440, #6204 ) ;
#15710=DIRECTION ( 'NONE',  ( -1.000000000000000000, -0.000000000000000000, -0.000000000000000000 ) ) ;
#15715=EDGE_CURVE ( 'NONE', #55113, #37337, #32407, .T. ) ;
#15722=CARTESIAN_POINT ( 'NONE',  ( 1.403614904275686858E-14, 1.537401574803149984, -3.937007874015761910 ) ) ;
#15737=CIRCLE ( 'NONE', #21066, 2.559055118110236560 ) ;
#15748=CARTESIAN_POINT ( 'NONE',  ( -0.3811349131313276350, 1.253490138500164441, -2.704685859045969476 ) ) ;
#15750=DIRECTION ( 'NONE',  ( 1.408710688920637755E-15, -1.000000000000000000, 4.918487082195260922E-30 ) ) ;
#15754=ORIENTED_EDGE ( 'NONE', *, *, #79927, .F. ) ;
#15759=CARTESIAN_POINT ( 'NONE',  ( 0.4177787735907000366, 0.000000000000000000, -1.874132239285499324 ) ) ;
#15767=ORIENTED_EDGE ( 'NONE', *, *, #25250, .T. ) ;
#15775=CARTESIAN_POINT ( 'NONE',  ( 1.813482582612293559, 2.755905511811024056, 0.5314960629921260393 ) ) ;
#15784=CARTESIAN_POINT ( 'NONE',  ( 2.571698080334759329, 1.622209144264170844, -0.4670403427556020226 ) ) ;
#15794=CIRCLE ( 'NONE', #10439, 1.289370078740159409 ) ;
#15805=CARTESIAN_POINT ( 'NONE',  ( 0.01711285633636193751, 1.063222675620814295, 1.850607425301893372 ) ) ;
#15809=CARTESIAN_POINT ( 'NONE',  ( -2.362204724409448620, 1.724409448818898127, -0.5118110236220719811 ) ) ;
#15825=EDGE_CURVE ( 'NONE', #8695, #64186, #61408, .T. ) ;
#15857=VERTEX_POINT ( 'NONE', #78718 ) ;
#15860=DIRECTION ( 'NONE',  ( 0.000000000000000000, 0.000000000000000000, 1.000000000000000000 ) ) ;
#15861=CONICAL_SURFACE ( 'NONE', #75025, 0.1978346456692914035, 0.8726646259971700959 ) ;
#15874=CARTESIAN_POINT ( 'NONE',  ( 0.5314960629921395840, 2.725419031863056674, -3.884512598959603658 ) ) ;
#15875=ORIENTED_EDGE ( 'NONE', *, *, #58155, .T. ) ;
#15885=CARTESIAN_POINT ( 'NONE',  ( -0.5314960629921373636, 2.755905511811024056, 3.264097702071371288 ) ) ;
#15907=CARTESIAN_POINT ( 'NONE',  ( 1.348312163386739426, 0.2755905511811023723, 0.7386866130305692613 ) ) ;
#15919=EDGE_CURVE ( 'NONE', #50774, #29467, #79972, .T. ) ;
#15930=DIRECTION ( 'NONE',  ( -1.000000000000000000, -9.738798461624180871E-16, -8.881784197001252323E-16 ) ) ;
#15936=EDGE_LOOP ( 'NONE', ( #78765, #66471, #13569, #11058 ) ) ;
#15961=CARTESIAN_POINT ( 'NONE',  ( 0.4359958488159307310, 1.724409448818897905, 3.937007874015793885 ) ) ;
#15966=VERTEX_POINT ( 'NONE', #34922 ) ;
#15969=ORIENTED_EDGE ( 'NONE', *, *, #14729, .T. ) ;
#15996=CARTESIAN_POINT ( 'NONE',  ( -2.169555354230969790, 1.520093187801265566, -0.4741711390158128703 ) ) ;
#16024=CARTESIAN_POINT ( 'NONE',  ( 0.000000000000000000, 2.755905511811024056, 0.000000000000000000 ) ) ;
#16026=DIRECTION ( 'NONE',  ( -0.000000000000000000, -1.000000000000000000, -0.000000000000000000 ) ) ;
#16033=ORIENTED_EDGE ( 'NONE', *, *, #56352, .F. ) ;
#16036=ORIENTED_EDGE ( 'NONE', *, *, #25941, .T. ) ;
#16042=CARTESIAN_POINT ( 'NONE',  ( -0.4670766846050908305, 1.622013716815570827, -2.571617139894965209 ) ) ;
#16080=CARTESIAN_POINT ( 'NONE',  ( 0.000000000000000000, 0.04488074079120461107, 0.000000000000000000 ) ) ;
#16089=DIRECTION ( 'NONE',  ( 0.000000000000000000, 0.000000000000000000, -1.000000000000000000 ) ) ;
#16117=CARTESIAN_POINT ( 'NONE',  ( -1.587201285915124771, 1.129514784140639883, 0.2422955380000797188 ) ) ;
#16119=CARTESIAN_POINT ( 'NONE',  ( -0.5314960629921349211, 2.716535433070866645, 2.543486866223387377 ) ) ;
#16121=DIRECTION ( 'NONE',  ( -0.000000000000000000, -1.000000000000000000, -0.000000000000000000 ) ) ;
#16130=DIRECTION ( 'NONE',  ( -3.491481338843133355E-15, -0.000000000000000000, 1.000000000000000000 ) ) ;
#16133=EDGE_CURVE ( 'NONE', #55951, #19971, #66080, .T. ) ;
#16141=EDGE_CURVE ( 'NONE', #62716, #33549, #8416, .T. ) ;
#16156=CARTESIAN_POINT ( 'NONE',  ( -0.4732434500808642697, 1.503067092966740459, -2.557121834200730248 ) ) ;
#16158=DIRECTION ( 'NONE',  ( -0.000000000000000000, 1.000000000000000000, -0.000000000000000000 ) ) ;
#16160=ORIENTED_EDGE ( 'NONE', *, *, #56352, .T. ) ;
#16165=DIRECTION ( 'NONE',  ( -3.491481338843132961E-15, -0.000000000000000000, 1.000000000000000000 ) ) ;
#16168=EDGE_CURVE ( 'NONE', #13017, #17581, #82941, .T. ) ;
#16170=DIRECTION ( 'NONE',  ( 0.000000000000000000, 0.000000000000000000, 1.000000000000000000 ) ) ;
#16176=EDGE_LOOP ( 'NONE', ( #40243, #24254 ) ) ;
#16178=CARTESIAN_POINT ( 'NONE',  ( -1.077419734549938779, 1.180567382142206467, 0.3141180532221660715 ) ) ;
#16186=DIRECTION ( 'NONE',  ( -0.000000000000000000, 1.000000000000000000, -0.000000000000000000 ) ) ;
#16194=DIRECTION ( 'NONE',  ( 0.000000000000000000, -1.000000000000000000, 0.000000000000000000 ) ) ;
#16216=CYLINDRICAL_SURFACE ( 'NONE', #74344, 0.4744094488188972947 ) ;
#16218=ORIENTED_EDGE ( 'NONE', *, *, #9376, .F. ) ;
#16257=AXIS2_PLACEMENT_3D ( 'NONE', #67503, #69151, #68740 ) ;
#16264=ORIENTED_EDGE ( 'NONE', *, *, #54110, .T. ) ;
#16267=CARTESIAN_POINT ( 'NONE',  ( 6.265965269058076312E-17, 1.062992125984252745, -1.850393700787401619 ) ) ;
#16273=B_SPLINE_CURVE_WITH_KNOTS ( 'NONE', 3,
 ( #77451, #6314, #25253, #50917, #78295, #26515, #58494, #70714, #70290, #33257, #12235, #5902 ),
 .UNSPECIFIED., .F., .F.,
 ( 4, 2, 2, 2, 2, 4 ),
 ( 0.05454303362711843822, 0.05585633982237198786, 0.05651299291999875574, 0.05716964601762552362, 0.05848295221287904549, 0.05979625840813256737 ),
 .UNSPECIFIED. ) ;
#16281=CIRCLE ( 'NONE', #75386, 3.858267716535433323 ) ;
#16285=DIRECTION ( 'NONE',  ( 0.000000000000000000, 0.000000000000000000, 1.000000000000000000 ) ) ;
#16301=EDGE_CURVE ( 'NONE', #60855, #19993, #80273, .T. ) ;
#16316=DIRECTION ( 'NONE',  ( 0.000000000000000000, 0.000000000000000000, -1.000000000000000000 ) ) ;
#16327=DIRECTION ( 'NONE',  ( 0.000000000000000000, 0.000000000000000000, 1.000000000000000000 ) ) ;
#16332=CONICAL_SURFACE ( 'NONE', #13621, 0.09842519685039351207, 1.029744258676652091 ) ;
#16362=ORIENTED_EDGE ( 'NONE', *, *, #13185, .F. ) ;
#16406=CARTESIAN_POINT ( 'NONE',  ( -3.908320185825792326, 1.537401574803149984, 0.4744094488188970171 ) ) ;
#16426=CARTESIAN_POINT ( 'NONE',  ( 1.016821367227983774, 1.537401574803149984, -0.4744094488188970171 ) ) ;
#16435=AXIS2_PLACEMENT_3D ( 'NONE', #81031, #36800, #16640 ) ;
#16437=CARTESIAN_POINT ( 'NONE',  ( 0.4744094488188886904, 1.528796061338913104, 2.554262525012302554 ) ) ;
#16440=CARTESIAN_POINT ( 'NONE',  ( 0.000000000000000000, 0.000000000000000000, 0.000000000000000000 ) ) ;
#16447=ORIENTED_EDGE ( 'NONE', *, *, #40694, .F. ) ;
#16450=VERTEX_POINT ( 'NONE', #74471 ) ;
#16468=VERTEX_POINT ( 'NONE', #43682 ) ;
#16480=DIRECTION ( 'NONE',  ( 1.047444401652940007E-14, -0.000000000000000000, -1.000000000000000000 ) ) ;
#16482=CARTESIAN_POINT ( 'NONE',  ( -0.5314960629921371416, 2.729659898468815182, 3.210901144249700412 ) ) ;
#16497=FACE_OUTER_BOUND ( 'NONE', #70374, .T. ) ;
#16503=CIRCLE ( 'NONE', #27228, 2.165354330708661568 ) ;
#16505=CARTESIAN_POINT ( 'NONE',  ( -0.1241822272904720692, 1.079268584176191093, -1.115255186249766384 ) ) ;
#16539=CARTESIAN_POINT ( 'NONE',  ( 2.103512204792505447, 1.710976477253049577, -0.4417575354491481421 ) ) ;
#16548=EDGE_CURVE ( 'NONE', #68098, #9892, #9953, .T. ) ;
#16552=CARTESIAN_POINT ( 'NONE',  ( -0.03177986912255784807, 1.063795733429741874, 1.121706799229931217 ) ) ;
#16574=CARTESIAN_POINT ( 'NONE',  ( -0.4698482617964682140, 1.469690627553818185, -2.565218379528205528 ) ) ;
#16583=DIRECTION ( 'NONE',  ( 0.000000000000000000, -1.000000000000000000, 0.000000000000000000 ) ) ;
#16585=CARTESIAN_POINT ( 'NONE',  ( 0.5314960629920917334, 2.755905511811024056, 3.264097702071378393 ) ) ;
#16589=CIRCLE ( 'NONE', #4434, 1.122047244094488194 ) ;
#16593=CARTESIAN_POINT ( 'NONE',  ( -1.109377953303970266, 1.093753137590900648, 0.1687621725689344154 ) ) ;
#16599=CARTESIAN_POINT ( 'NONE',  ( -3.937007874015748143, 2.559055118110236560, -0.5314960629921260393 ) ) ;
#16606=AXIS2_PLACEMENT_3D ( 'NONE', #31507, #24774, #76555 ) ;
#16640=DIRECTION ( 'NONE',  ( 0.000000000000000000, 0.000000000000000000, -1.000000000000000000 ) ) ;
#16649=DIRECTION ( 'NONE',  ( 0.000000000000000000, -0.6427876096865352551, -0.7660444431189814551 ) ) ;
#16650=CIRCLE ( 'NONE', #58244, 0.1978346456692914035 ) ;
#16664=AXIS2_PLACEMENT_3D ( 'NONE', #50570, #17793, #25315 ) ;
#16679=ORIENTED_EDGE ( 'NONE', *, *, #2416, .T. ) ;
#16681=ORIENTED_EDGE ( 'NONE', *, *, #63509, .F. ) ;
#16686=CARTESIAN_POINT ( 'NONE',  ( -0.5314960629921323676, 2.742788276420188520, 1.827151573187007161 ) ) ;
#16687=CARTESIAN_POINT ( 'NONE',  ( -3.908320185825792326, 1.537401574803149984, -0.4744094488188975722 ) ) ;
#16724=AXIS2_PLACEMENT_3D ( 'NONE', #3739, #56309, #67721 ) ;
#16744=EDGE_CURVE ( 'NONE', #6386, #50169, #34593, .T. ) ;
#16759=ORIENTED_EDGE ( 'NONE', *, *, #75818, .T. ) ;
#16765=CIRCLE ( 'NONE', #30142, 1.122047244094488194 ) ;
#16775=ORIENTED_EDGE ( 'NONE', *, *, #79045, .F. ) ;
#16794=CARTESIAN_POINT ( 'NONE',  ( -0.6299212598425059095, 1.724409448818897905, -3.937007874015764131 ) ) ;
#16811=ADVANCED_FACE ( 'NONE', ( #76749 ), #12780, .F. ) ;
#16832=DIRECTION ( 'NONE',  ( 1.408710688920637755E-15, -1.000000000000000000, 4.918487082195260922E-30 ) ) ;
#16847=CIRCLE ( 'NONE', #77259, 1.122047244094488194 ) ;
#16851=ORIENTED_EDGE ( 'NONE', *, *, #46574, .F. ) ;
#16856=CARTESIAN_POINT ( 'NONE',  ( 0.000000000000000000, 2.755905511811024056, 0.000000000000000000 ) ) ;
#16862=EDGE_CURVE ( 'NONE', #10444, #5673, #52304, .T. ) ;
#16864=VERTEX_POINT ( 'NONE', #33800 ) ;
#16867=ORIENTED_EDGE ( 'NONE', *, *, #3552, .T. ) ;
#16878=CARTESIAN_POINT ( 'NONE',  ( 0.01706770257043118549, 1.062992125984252301, -2.874015748031495399 ) ) ;
#16920=CARTESIAN_POINT ( 'NONE',  ( -2.554262525012223062, 1.528804020127598973, 0.4744094488188971281 ) ) ;
#16936=CARTESIAN_POINT ( 'NONE',  ( -0.02273980556643043910, 1.063502421567459111, -1.634061201692638132 ) ) ;
#16951=ADVANCED_FACE ( 'NONE', ( #33390 ), #20338, .F. ) ;
#16952=CARTESIAN_POINT ( 'NONE',  ( -1.645124945854690601, 1.142361046343763897, 0.2627170963995461572 ) ) ;
#16953=DIRECTION ( 'NONE',  ( 0.000000000000000000, -1.000000000000000000, 0.000000000000000000 ) ) ;
#16957=AXIS2_PLACEMENT_3D ( 'NONE', #38393, #77121, #56914 ) ;
#16961=ORIENTED_EDGE ( 'NONE', *, *, #22393, .T. ) ;
#16976=CARTESIAN_POINT ( 'NONE',  ( 0.4177787735907000366, 0.3937007874015747699, -1.559171609364239375 ) ) ;
#16996=AXIS2_PLACEMENT_3D ( 'NONE', #59951, #53625, #73003 ) ;
#16999=VECTOR ( 'NONE', #15063, 39.37007874015748143 ) ;
#17000=CIRCLE ( 'NONE', #27731, 3.937007874015748143 ) ;
#17012=CARTESIAN_POINT ( 'NONE',  ( -1.038160555197627399, 1.326112492113292518, 0.4258879071893178492 ) ) ;
#17035=CARTESIAN_POINT ( 'NONE',  ( 0.4256376116915605023, 1.327230063460893783, -1.689708071488565500 ) ) ;
#17041=LINE ( 'NONE', #55306, #12441 ) ;
#17048=CARTESIAN_POINT ( 'NONE',  ( 0.1656158939409557440, 1.092528437896314486, 1.877649196272271226 ) ) ;
#17057=AXIS2_PLACEMENT_3D ( 'NONE', #60684, #21555, #3034 ) ;
#17058=CARTESIAN_POINT ( 'NONE',  ( -2.129998074986464207, 1.668416680336017421, -0.4562095852119731343 ) ) ;
#17062=AXIS2_PLACEMENT_3D ( 'NONE', #12458, #26322, #18374 ) ;
#17069=CARTESIAN_POINT ( 'NONE',  ( 0.4177787735907000366, 0.3937007874015748254, -1.559171609364239375 ) ) ;
#17079=DIRECTION ( 'NONE',  ( -0.000000000000000000, -1.000000000000000000, -0.000000000000000000 ) ) ;
#17115=VERTEX_POINT ( 'NONE', #59878 ) ;
#17119=CARTESIAN_POINT ( 'NONE',  ( 0.000000000000000000, 0.4201155382560080032, 0.000000000000000000 ) ) ;
#17120=EDGE_CURVE ( 'NONE', #76587, #40450, #58068, .T. ) ;
#17125=AXIS2_PLACEMENT_3D ( 'NONE', #95, #25332, #51411 ) ;
#17126=CIRCLE ( 'NONE', #31859, 3.858267716535433323 ) ;
#17173=AXIS2_PLACEMENT_3D ( 'NONE', #37442, #37027, #10950 ) ;
#17176=ORIENTED_EDGE ( 'NONE', *, *, #57314, .F. ) ;
#17178=VERTEX_POINT ( 'NONE', #72104 ) ;
#17193=ORIENTED_EDGE ( 'NONE', *, *, #53241, .F. ) ;
#17202=CARTESIAN_POINT ( 'NONE',  ( 0.4478583149154592435, 1.694693813591205300, 1.028805191090655935 ) ) ;
#17208=ORIENTED_EDGE ( 'NONE', *, *, #71135, .T. ) ;
#17211=ORIENTED_EDGE ( 'NONE', *, *, #28505, .F. ) ;
#17239=AXIS2_PLACEMENT_3D ( 'NONE', #44939, #43293, #70216 ) ;
#17240=CARTESIAN_POINT ( 'NONE',  ( -2.077234194078065865, 1.326002914239481356, 0.4256865378621424445 ) ) ;
#17265=ORIENTED_EDGE ( 'NONE', *, *, #82913, .F. ) ;
#17271=DIRECTION ( 'NONE',  ( 0.000000000000000000, -1.000000000000000000, 0.000000000000000000 ) ) ;
#17333=CARTESIAN_POINT ( 'NONE',  ( -2.776658174029175363, 1.170105060311657619, 0.3006284332565994366 ) ) ;
#17336=DIRECTION ( 'NONE',  ( 0.000000000000000000, 0.000000000000000000, 1.000000000000000000 ) ) ;
#17346=CARTESIAN_POINT ( 'NONE',  ( 0.1085784267831624711, 1.075318549932396728, -1.116887896051823814 ) ) ;
#17348=EDGE_CURVE ( 'NONE', #77755, #58154, #69486, .T. ) ;
#17351=CARTESIAN_POINT ( 'NONE',  ( 0.4122598602536549084, 1.300945800302083288, -2.057903956725271488 ) ) ;
#17368=LINE ( 'NONE', #74609, #19103 ) ;
#17390=CARTESIAN_POINT ( 'NONE',  ( 0.4614150585118587666, 1.648843903847227566, 3.909876957777870476 ) ) ;
#17405=CARTESIAN_POINT ( 'NONE',  ( -0.4606671848300740169, 1.422950954677616897, -2.585357360710740515 ) ) ;
#17414=CARTESIAN_POINT ( 'NONE',  ( -1.028793376639876023, 1.694622884024324261, 0.4478856567166526470 ) ) ;
#17415=CARTESIAN_POINT ( 'NONE',  ( -3.264097702071373064, 2.755905511811024056, -0.5314960629921260393 ) ) ;
#17440=LINE ( 'NONE', #76327, #27672 ) ;
#17448=CARTESIAN_POINT ( 'NONE',  ( 1.084092808546051057, 1.161348697294517951, 0.2896277429123272351 ) ) ;
#17461=DIRECTION ( 'NONE',  ( 0.000000000000000000, -1.000000000000000000, 0.000000000000000000 ) ) ;
#17465=ORIENTED_EDGE ( 'NONE', *, *, #58706, .T. ) ;
#17477=CARTESIAN_POINT ( 'NONE',  ( -0.4589048803027434009, 1.413024577066673615, 1.023935092353904563 ) ) ;
#17478=CARTESIAN_POINT ( 'NONE',  ( 3.911446811352371711, 1.694514647449913092, 0.4479265895742980397 ) ) ;
#17496=DIRECTION ( 'NONE',  ( 0.000000000000000000, 1.000000000000000000, -0.000000000000000000 ) ) ;
#17509=CARTESIAN_POINT ( 'NONE',  ( -0.03443470937339728616, 1.062992125984252079, -1.537015892239756099 ) ) ;
#17514=DIRECTION ( 'NONE',  ( 0.000000000000000000, -1.000000000000000000, 0.000000000000000000 ) ) ;
#17522=ORIENTED_EDGE ( 'NONE', *, *, #70814, .T. ) ;
#17524=DIRECTION ( 'NONE',  ( 1.000000000000000000, 0.000000000000000000, 3.455050906509825972E-15 ) ) ;
#17552=CARTESIAN_POINT ( 'NONE',  ( -3.831929248781927200, 2.755905511811024056, 0.5314960629921259283 ) ) ;
#17555=ORIENTED_EDGE ( 'NONE', *, *, #4697, .T. ) ;
#17581=VERTEX_POINT ( 'NONE', #45351 ) ;
#17583=ORIENTED_EDGE ( 'NONE', *, *, #66595, .T. ) ;
#17606=CARTESIAN_POINT ( 'NONE',  ( -0.4359958488159583201, 1.724409448818897905, -3.912791665790201101 ) ) ;
#17608=DIRECTION ( 'NONE',  ( 0.000000000000000000, -1.000000000000000000, 0.000000000000000000 ) ) ;
#17612=CARTESIAN_POINT ( 'NONE',  ( 3.911297246792111881, 1.384105334947628885, 0.4492278415794215274 ) ) ;
#17614=ORIENTED_EDGE ( 'NONE', *, *, #26633, .T. ) ;
#17616=CARTESIAN_POINT ( 'NONE',  ( 0.000000000000000000, 0.4201155382560080032, 0.000000000000000000 ) ) ;
#17619=DIRECTION ( 'NONE',  ( 1.408710688920637755E-15, -1.000000000000000000, 4.918487082195260922E-30 ) ) ;
#17642=FACE_OUTER_BOUND ( 'NONE', #25546, .T. ) ;
#17652=AXIS2_PLACEMENT_3D ( 'NONE', #58166, #1782, #53103 ) ;
#17653=EDGE_CURVE ( 'NONE', #81379, #38353, #33199, .T. ) ;
#17662=CARTESIAN_POINT ( 'NONE',  ( -3.924551336943372881, 1.180704189158721329, 0.3131659068132852108 ) ) ;
#17666=CARTESIAN_POINT ( 'NONE',  ( -0.5314960629921123836, 2.755905511811024056, -3.900966923095591454 ) ) ;
#17667=ORIENTED_EDGE ( 'NONE', *, *, #11964, .F. ) ;
#17674=EDGE_CURVE ( 'NONE', #60217, #63415, #12555, .T. ) ;
#17677=DIRECTION ( 'NONE',  ( -0.000000000000000000, -1.000000000000000000, -0.000000000000000000 ) ) ;
#17684=ORIENTED_EDGE ( 'NONE', *, *, #63827, .T. ) ;
#17690=CARTESIAN_POINT ( 'NONE',  ( 0.000000000000000000, 0.000000000000000000, 0.000000000000000000 ) ) ;
#17692=AXIS2_PLACEMENT_3D ( 'NONE', #9428, #1871, #28362 ) ;
#17695=CARTESIAN_POINT ( 'NONE',  ( 0.4734688692633114981, 1.503144958756604366, -2.556625226394979578 ) ) ;
#17701=EDGE_LOOP ( 'NONE', ( #52951, #36072, #42734, #40595 ) ) ;
#17721=B_SPLINE_CURVE_WITH_KNOTS ( 'NONE', 3,
 ( #15885, #14220, #33977, #39880 ),
 .UNSPECIFIED., .F., .F.,
 ( 4, 4 ),
 ( 9.959548797825900302E-07, 0.001423907596959053667 ),
 .UNSPECIFIED. ) ;
#17730=PLANE ( 'NONE',  #49890 ) ;
#17733=FACE_OUTER_BOUND ( 'NONE', #71756, .T. ) ;
#17754=CARTESIAN_POINT ( 'NONE',  ( 0.1341320108093697061, 1.082050302230247896, -1.868011637380655232 ) ) ;
#17759=DIRECTION ( 'NONE',  ( -0.000000000000000000, -1.000000000000000000, -0.000000000000000000 ) ) ;
#17772=CARTESIAN_POINT ( 'NONE',  ( 0.4177787735907000366, 1.299212598425196985, -1.382006255033530806 ) ) ;
#17784=DIRECTION ( 'NONE',  ( 1.000000000000000000, 0.000000000000000000, 3.455050906509825972E-15 ) ) ;
#17793=DIRECTION ( 'NONE',  ( -0.000000000000000000, -1.000000000000000000, 8.673617379884024625E-16 ) ) ;
#17794=CARTESIAN_POINT ( 'NONE',  ( -0.5314960629921224866, 2.755905511811024056, -0.9881811337016660479 ) ) ;
#17795=ORIENTED_EDGE ( 'NONE', *, *, #79452, .F. ) ;
#17812=CONICAL_SURFACE ( 'NONE', #58086, 1.968503937007874072, 0.7853981633974500554 ) ;
#17817=VERTEX_POINT ( 'NONE', #60078 ) ;
#17820=CARTESIAN_POINT ( 'NONE',  ( -1.018726825260306112, 1.601686773136587805, 0.4703072575216136197 ) ) ;
#17821=CARTESIAN_POINT ( 'NONE',  ( 0.6299212598424784870, 1.724409448818897905, 3.937007874015796105 ) ) ;
#17854=CARTESIAN_POINT ( 'NONE',  ( 1.044155967855882050, 1.298756420147472390, 0.4111758506720307738 ) ) ;
#17865=AXIS2_PLACEMENT_3D ( 'NONE', #10381, #10787, #55380 ) ;
#17867=DIRECTION ( 'NONE',  ( 0.000000000000000000, 1.000000000000000000, 0.000000000000000000 ) ) ;
#17871=ORIENTED_EDGE ( 'NONE', *, *, #76605, .T. ) ;
#17875=CARTESIAN_POINT ( 'NONE',  ( -2.138259192565297173, 1.653403552777525487, -0.4602852883866582201 ) ) ;
#17883=CARTESIAN_POINT ( 'NONE',  ( -0.4104818416650150570, 1.299051044647045128, 1.044297694901411555 ) ) ;
#17884=LINE ( 'NONE', #62903, #76222 ) ;
#17905=CIRCLE ( 'NONE', #67656, 2.165354330708661568 ) ;
#17920=CARTESIAN_POINT ( 'NONE',  ( 1.141392835773559211, 0.3937007874015747699, 1.339227481442854195 ) ) ;
#17932=FACE_OUTER_BOUND ( 'NONE', #78665, .T. ) ;
#17938=ORIENTED_EDGE ( 'NONE', *, *, #69071, .T. ) ;
#17940=CARTESIAN_POINT ( 'NONE',  ( -0.4653577321740608452, 1.629972608277046708, 2.575297182719555877 ) ) ;
#17960=CARTESIAN_POINT ( 'NONE',  ( -3.900966923095587457, 2.682389230697235671, 0.5314960629921258173 ) ) ;
#17975=CIRCLE ( 'NONE', #16606, 3.937007874015748143 ) ;
#17977=CARTESIAN_POINT ( 'NONE',  ( 0.3227188174119076658, 1.189353863002647449, 2.759699577397270343 ) ) ;
#17981=CARTESIAN_POINT ( 'NONE',  ( 1.495848283907322829E-16, 0.4201155382560080032, 1.198416298106748767 ) ) ;
#17991=ORIENTED_EDGE ( 'NONE', *, *, #52780, .F. ) ;
#18005=ORIENTED_EDGE ( 'NONE', *, *, #32101, .T. ) ;
#18015=LINE ( 'NONE', #43238, #20075 ) ;
#18017=DIRECTION ( 'NONE',  ( 0.000000000000000000, 0.000000000000000000, -1.000000000000000000 ) ) ;
#18020=AXIS2_PLACEMENT_3D ( 'NONE', #81374, #67494, #74648 ) ;
#18042=CIRCLE ( 'NONE', #16724, 3.937007874015748143 ) ;
#18049=CARTESIAN_POINT ( 'NONE',  ( -1.559171609364246924, 0.000000000000000000, 0.4177787735906735578 ) ) ;
#18060=LINE ( 'NONE', #50428, #56922 ) ;
#18070=DIRECTION ( 'NONE',  ( 0.000000000000000000, 0.000000000000000000, 1.000000000000000000 ) ) ;
#18076=CIRCLE ( 'NONE', #50316, 2.559055118110236560 ) ;
#18082=CARTESIAN_POINT ( 'NONE',  ( -1.559171609364246924, 0.3937007874015748254, 0.4177787735906735578 ) ) ;
#18092=ORIENTED_EDGE ( 'NONE', *, *, #39798, .F. ) ;
#18108=EDGE_LOOP ( 'NONE', ( #21522, #63769, #53206, #35290 ) ) ;
#18142=CARTESIAN_POINT ( 'NONE',  ( -2.857004350179353391, 1.081388112195873497, 0.1351566381870255573 ) ) ;
#18148=ADVANCED_FACE ( 'NONE', ( #78628 ), #50715, .T. ) ;
#18157=CARTESIAN_POINT ( 'NONE',  ( 1.374111566022513293E-16, 1.062992125984252745, -1.122047244094488194 ) ) ;
#18159=EDGE_CURVE ( 'NONE', #27377, #33346, #63157, .T. ) ;
#18166=CARTESIAN_POINT ( 'NONE',  ( -0.4323334181381108254, 1.341458022389044658, -3.913202610827236860 ) ) ;
#18171=LINE ( 'NONE', #9473, #32670 ) ;
#18181=CARTESIAN_POINT ( 'NONE',  ( -2.362204724409448620, 1.929133858267716661, -2.474278114140802984E-14 ) ) ;
#18192=CARTESIAN_POINT ( 'NONE',  ( -0.03443470937339727228, 0.2755905511811023723, -1.417921404050779710 ) ) ;
#18194=CARTESIAN_POINT ( 'NONE',  ( 1.403614904275686858E-14, 1.537401574803149984, -3.937007874015761910 ) ) ;
#18203=CARTESIAN_POINT ( 'NONE',  ( -0.3335738234991588169, 1.199759523613727952, -1.973797438880085187 ) ) ;
#18204=ORIENTED_EDGE ( 'NONE', *, *, #9628, .T. ) ;
#18208=VECTOR ( 'NONE', #29297, 39.37007874015748143 ) ;
#18220=CARTESIAN_POINT ( 'NONE',  ( 0.000000000000000000, 2.716535433070866645, 0.000000000000000000 ) ) ;
#18223=ORIENTED_EDGE ( 'NONE', *, *, #57314, .T. ) ;
#18227=CARTESIAN_POINT ( 'NONE',  ( 0.000000000000000000, 2.165354330708661568, 0.000000000000000000 ) ) ;
#18246=CARTESIAN_POINT ( 'NONE',  ( -0.4671901501889756392, 1.453473631083801676, 2.153053328784569231 ) ) ;
#18260=CARTESIAN_POINT ( 'NONE',  ( 1.016821367227983552, 1.505646504554443821, 0.4744094488188977388 ) ) ;
#18292=CARTESIAN_POINT ( 'NONE',  ( 3.908320185825791881, 1.537401574803149984, 0.4744094488188975722 ) ) ;
#18297=EDGE_CURVE ( 'NONE', #80751, #30111, #74208, .T. ) ;
#18305=AXIS2_PLACEMENT_3D ( 'NONE', #5200, #57349, #76730 ) ;
#18320=EDGE_CURVE ( 'NONE', #65211, #32057, #7731, .T. ) ;
#18332=DIRECTION ( 'NONE',  ( 0.000000000000000000, 1.000000000000000000, -0.000000000000000000 ) ) ;
#18364=CIRCLE ( 'NONE', #39875, 1.122047244094488194 ) ;
#18366=AXIS2_PLACEMENT_3D ( 'NONE', #46475, #26713, #52790 ) ;
#18368=EDGE_CURVE ( 'NONE', #46245, #76474, #29228, .T. ) ;
#18374=DIRECTION ( 'NONE',  ( 0.000000000000000000, -0.000000000000000000, 1.000000000000000000 ) ) ;
#18375=CARTESIAN_POINT ( 'NONE',  ( 0.5314960629921395840, 2.559055118110236560, -3.900966923095588346 ) ) ;
#18385=DIRECTION ( 'NONE',  ( 0.000000000000000000, -1.000000000000000000, 0.000000000000000000 ) ) ;
#18390=CARTESIAN_POINT ( 'NONE',  ( 0.4122368018044499927, 1.300920202588029317, 2.666527984212822666 ) ) ;
#18403=ORIENTED_EDGE ( 'NONE', *, *, #25337, .T. ) ;
#18404=ORIENTED_EDGE ( 'NONE', *, *, #20837, .T. ) ;
#18417=VECTOR ( 'NONE', #51331, 39.37007874015748143 ) ;
#18418=ORIENTED_EDGE ( 'NONE', *, *, #10568, .F. ) ;
#18420=VECTOR ( 'NONE', #75796, 39.37007874015748143 ) ;
#18437=CARTESIAN_POINT ( 'NONE',  ( -1.559171609364246924, 0.3937007874015748254, 0.7327394035119333404 ) ) ;
#18438=ORIENTED_EDGE ( 'NONE', *, *, #75948, .F. ) ;
#18444=PLANE ( 'NONE',  #51938 ) ;
#18447=CYLINDRICAL_SURFACE ( 'NONE', #950, 0.4744094488188972947 ) ;
#18481=CARTESIAN_POINT ( 'NONE',  ( -3.923618555848779721, 1.191084733186814848, -0.3246066631975622618 ) ) ;
#18485=FACE_OUTER_BOUND ( 'NONE', #4399, .T. ) ;
#18487=DIRECTION ( 'NONE',  ( -5.329070518200751394E-15, 0.000000000000000000, -1.000000000000000000 ) ) ;
#18495=LINE ( 'NONE', #50050, #71805 ) ;
#18501=ORIENTED_EDGE ( 'NONE', *, *, #29024, .F. ) ;
#18514=ORIENTED_EDGE ( 'NONE', *, *, #63922, .T. ) ;
#18516=ORIENTED_EDGE ( 'NONE', *, *, #45608, .F. ) ;
#18549=CARTESIAN_POINT ( 'NONE',  ( -2.723802780027896553, 1.230840736494979604, -0.3632157284009264187 ) ) ;
#18563=DIRECTION ( 'NONE',  ( 0.000000000000000000, 0.000000000000000000, -1.000000000000000000 ) ) ;
#18576=CARTESIAN_POINT ( 'NONE',  ( 0.000000000000000000, 1.724409448818900570, 2.362204724409448620 ) ) ;
#18586=CARTESIAN_POINT ( 'NONE',  ( -0.3149606299212633354, 2.165354330708661568, 1.076935383196057305 ) ) ;
#18598=CARTESIAN_POINT ( 'NONE',  ( 0.3149606299212737159, 2.165354330708661568, -3.937007874015761022 ) ) ;
#18600=CARTESIAN_POINT ( 'NONE',  ( 0.5314960629921371416, 2.742783277647743212, -3.197598474799420831 ) ) ;
#18609=CARTESIAN_POINT ( 'NONE',  ( -0.1180926326102824109, 1.077616795999335242, -1.863921337943197365 ) ) ;
#18613=ORIENTED_EDGE ( 'NONE', *, *, #11964, .T. ) ;
#18625=FACE_OUTER_BOUND ( 'NONE', #10055, .T. ) ;
#18633=CARTESIAN_POINT ( 'NONE',  ( -1.559171609364246924, 1.299212598425196985, 0.4177787735906735578 ) ) ;
#18651=CARTESIAN_POINT ( 'NONE',  ( -0.3636368138136299444, 1.231320578257673715, 2.001016126126115235 ) ) ;
#18671=CARTESIAN_POINT ( 'NONE',  ( 1.033875059083676717, 1.724409448818897905, -0.4359958488159719758 ) ) ;
#18680=EDGE_CURVE ( 'NONE', #23049, #65196, #43015, .T. ) ;
#18682=ORIENTED_EDGE ( 'NONE', *, *, #57389, .T. ) ;
#18684=ADVANCED_FACE ( 'NONE', ( #70416 ), #49124, .F. ) ;
#18704=EDGE_CURVE ( 'NONE', #5673, #64597, #45996, .T. ) ;
#18709=ADVANCED_FACE ( 'NONE', ( #7712 ), #716, .F. ) ;
#18723=EDGE_LOOP ( 'NONE', ( #60646, #49876 ) ) ;
#18725=EDGE_LOOP ( 'NONE', ( #11599, #17265, #47178, #34365 ) ) ;
#18732=CARTESIAN_POINT ( 'NONE',  ( -0.5314960629921147151, 2.716535433070866645, -3.224202737261816942 ) ) ;
#18739=ORIENTED_EDGE ( 'NONE', *, *, #72215, .F. ) ;
#18747=CARTESIAN_POINT ( 'NONE',  ( 0.000000000000000000, 1.724409448818897461, 0.000000000000000000 ) ) ;
#18748=CARTESIAN_POINT ( 'NONE',  ( -1.559171609364246924, 0.4110443821404751730, 0.2406134192599649890 ) ) ;
#18773=ORIENTED_EDGE ( 'NONE', *, *, #53723, .T. ) ;
#18787=CARTESIAN_POINT ( 'NONE',  ( 6.267877385347666114E-17, 1.062992125984252745, 2.874015748031495843 ) ) ;
#18794=ADVANCED_FACE ( 'NONE', ( #40104 ), #65792, .F. ) ;
#18825=CARTESIAN_POINT ( 'NONE',  ( 3.886287458032462006, 2.755905511811024056, 0.6299212598425202314 ) ) ;
#18827=FACE_OUTER_BOUND ( 'NONE', #41191, .T. ) ;
#18834=EDGE_LOOP ( 'NONE', ( #11293, #73001, #38925, #72836, #42189, #54326, #46349, #71225, #72155, #47674 ) ) ;
#18879=CARTESIAN_POINT ( 'NONE',  ( 0.4744094488189112835, 1.537401574803149984, -3.908320185825791881 ) ) ;
#18891=DIRECTION ( 'NONE',  ( -3.491481338843132961E-15, 0.000000000000000000, 1.000000000000000000 ) ) ;
#18900=ORIENTED_EDGE ( 'NONE', *, *, #5310, .T. ) ;
#18916=EDGE_LOOP ( 'NONE', ( #18739, #75439, #62410, #30201 ) ) ;
#18929=CONICAL_SURFACE ( 'NONE', #29692, 1.889763779527559251, 0.7853981633974500554 ) ;
#18951=FACE_OUTER_BOUND ( 'NONE', #66542, .T. ) ;
#18966=CARTESIAN_POINT ( 'NONE',  ( 0.4567115769096108391, 1.408171547189567274, -2.130996229389289010 ) ) ;
#18972=CARTESIAN_POINT ( 'NONE',  ( -0.03101198675153587700, 1.063748311984392902, -3.936916529678083254 ) ) ;
#18981=VECTOR ( 'NONE', #82461, 39.37007874015748143 ) ;
#18986=CARTESIAN_POINT ( 'NONE',  ( -2.130073781772672259, 0.01305114060239450161, 0.4563452811745689064 ) ) ;
#18990=CARTESIAN_POINT ( 'NONE',  ( 3.937007874015748143, 2.755905511811024056, 0.5314960629921260393 ) ) ;
#19011=DIRECTION ( 'NONE',  ( 0.000000000000000000, -0.000000000000000000, 1.000000000000000000 ) ) ;
#19012=EDGE_LOOP ( 'NONE', ( #25528, #44144, #10144, #81437, #381, #2665 ) ) ;
#19015=VERTEX_POINT ( 'NONE', #9775 ) ;
#19026=CARTESIAN_POINT ( 'NONE',  ( 3.937007874015748143, 2.755905511811024056, -0.5314960629921260393 ) ) ;
#19031=ORIENTED_EDGE ( 'NONE', *, *, #37866, .T. ) ;
#19039=CARTESIAN_POINT ( 'NONE',  ( 2.130073781772669150, 0.01305114060239445997, -0.4563452811745837834 ) ) ;
#19057=CARTESIAN_POINT ( 'NONE',  ( -0.4725409811167128882, 1.494519345219277762, 2.165580946493155690 ) ) ;
#19062=CARTESIAN_POINT ( 'NONE',  ( 0.6299212598425100174, 2.165354330708661568, 0.9285414500055780840 ) ) ;
#19070=CARTESIAN_POINT ( 'NONE',  ( 1.018309906596789771, 1.474507693700183308, 0.4712541672117732672 ) ) ;
#19103=VECTOR ( 'NONE', #61128, 39.37007874015748143 ) ;
#19128=ORIENTED_EDGE ( 'NONE', *, *, #83089, .F. ) ;
#19134=CARTESIAN_POINT ( 'NONE',  ( -0.2512006810191820261, 1.134651008203183986, 2.808392084767333596 ) ) ;
#19135=DIRECTION ( 'NONE',  ( 1.000000000000000000, 0.000000000000000000, -0.000000000000000000 ) ) ;
#19143=EDGE_CURVE ( 'NONE', #31453, #28229, #54477, .T. ) ;
#19144=DIRECTION ( 'NONE',  ( 0.000000000000000000, 1.000000000000000000, 0.000000000000000000 ) ) ;
#19146=DIRECTION ( 'NONE',  ( 1.000000000000000000, -0.000000000000000000, -0.000000000000000000 ) ) ;
#19150=VERTEX_POINT ( 'NONE', #28297 ) ;
#19151=CARTESIAN_POINT ( 'NONE',  ( 0.000000000000000000, 2.755905511811024056, 0.000000000000000000 ) ) ;
#19152=DIRECTION ( 'NONE',  ( -1.000000000000000000, -8.326672684688674053E-16, 0.000000000000000000 ) ) ;
#19156=AXIS2_PLACEMENT_3D ( 'NONE', #63761, #12846, #50301 ) ;
#19179=ORIENTED_EDGE ( 'NONE', *, *, #30323, .F. ) ;
#19188=CARTESIAN_POINT ( 'NONE',  ( 0.5314960629921322566, 2.755905511811024056, -1.813482582612291782 ) ) ;
#19193=AXIS2_PLACEMENT_3D ( 'NONE', #76752, #17867, #49827 ) ;
#19194=CARTESIAN_POINT ( 'NONE',  ( 0.2893091866268030499, 1.161375622156852083, -1.681321774322261042 ) ) ;
#19206=EDGE_LOOP ( 'NONE', ( #5865, #55128, #68736, #16033, #35194, #80854, #13667, #68604, #32669, #66043, #82460, #39402, #10112, #73201 ) ) ;
#19207=ORIENTED_EDGE ( 'NONE', *, *, #38580, .F. ) ;
#19230=CARTESIAN_POINT ( 'NONE',  ( 0.000000000000000000, 0.03937007874015747977, 0.000000000000000000 ) ) ;
#19231=LINE ( 'NONE', #38593, #2614 ) ;
#19247=CARTESIAN_POINT ( 'NONE',  ( 2.167269426034547308, 1.502969453419623846, 0.4732359647714768358 ) ) ;
#19260=AXIS2_PLACEMENT_3D ( 'NONE', #45359, #32746, #58413 ) ;
#19273=AXIS2_PLACEMENT_3D ( 'NONE', #16976, #81360, #35486 ) ;
#19288=CARTESIAN_POINT ( 'NONE',  ( -3.931479177127797264, 1.111134681805650004, -0.2105673636452098652 ) ) ;
#19296=EDGE_LOOP ( 'NONE', ( #33020, #19179, #73610, #63352 ) ) ;
#19310=ORIENTED_EDGE ( 'NONE', *, *, #25809, .F. ) ;
#19337=EDGE_CURVE ( 'NONE', #40450, #39419, #80908, .T. ) ;
#19351=EDGE_CURVE ( 'NONE', #16864, #62412, #54118, .T. ) ;
#19393=EDGE_CURVE ( 'NONE', #9282, #36478, #36270, .T. ) ;
#19396=DIRECTION ( 'NONE',  ( -0.8660254037844433705, 0.000000000000000000, 0.4999999999999920064 ) ) ;
#19412=ORIENTED_EDGE ( 'NONE', *, *, #153, .F. ) ;
#19419=CARTESIAN_POINT ( 'NONE',  ( 3.924389226575468737, 2.559055118110236560, 0.3149606299212599492 ) ) ;
#19428=CARTESIAN_POINT ( 'NONE',  ( 0.000000000000000000, 0.4374015748031496176, 0.000000000000000000 ) ) ;
#19433=ORIENTED_EDGE ( 'NONE', *, *, #28964, .F. ) ;
#19446=CARTESIAN_POINT ( 'NONE',  ( 3.910259856776663767, 1.664469867010863746, -0.4581933108574676172 ) ) ;
#19542=VERTEX_POINT ( 'NONE', #40935 ) ;
#19550=CARTESIAN_POINT ( 'NONE',  ( -0.1656158939409619058, 1.092528437896311155, 2.846760252546623793 ) ) ;
#19551=DIRECTION ( 'NONE',  ( 0.000000000000000000, -0.6427876096865364763, -0.7660444431189804559 ) ) ;
#19558=ORIENTED_EDGE ( 'NONE', *, *, #67626, .T. ) ;
#19559=CARTESIAN_POINT ( 'NONE',  ( -1.028297472258253853, 1.383492524721027017, -0.4490203305827997204 ) ) ;
#19569=CARTESIAN_POINT ( 'NONE',  ( 0.000000000000000000, 0.000000000000000000, 2.362204724409448620 ) ) ;
#19592=DIRECTION ( 'NONE',  ( 0.000000000000000000, 0.000000000000000000, -1.000000000000000000 ) ) ;
#19596=EDGE_LOOP ( 'NONE', ( #72255, #62103 ) ) ;
#19603=AXIS2_PLACEMENT_3D ( 'NONE', #78352, #77931, #13124 ) ;
#19611=CARTESIAN_POINT ( 'NONE',  ( 0.2656293764155540083, 1.144263613740634566, -1.650922135227781418 ) ) ;
#19625=EDGE_LOOP ( 'NONE', ( #35685, #17522 ) ) ;
#19626=ORIENTED_EDGE ( 'NONE', *, *, #6477, .F. ) ;
#19637=B_SPLINE_CURVE_WITH_KNOTS ( 'NONE', 3,
 ( #56542, #5211, #30875, #53130, #27891, #78841, #40525, #79259, #989, #52715, #21167, #40108, #19919, #78004, #58622, #39263, #53962, #52298, #21574, #32955, #65380, #2226, #65795, #66204, #46823 ),
 .UNSPECIFIED., .F., .F.,
 ( 4, 2, 2, 2, 2, 2, 2, 2, 2, 1, 2, 2, 4 ),
 ( 0.000000000000000000, 0.002357302890897380095, 0.003535954336346069926, 0.004714605781794759323, 0.007071908672692136383, 0.008250560118140825780, 0.009429211563589516912, 0.01178651445448690438, 0.01296516589993559551, 0.01414381734538429011, 0.01532246879083298124, 0.01650112023628167238, 0.01885842312717905811 ),
 .UNSPECIFIED. ) ;
#19641=VERTEX_POINT ( 'NONE', #11847 ) ;
#19652=CARTESIAN_POINT ( 'NONE',  ( -0.02282215444009891639, 1.063505409135067525, -1.439960907823146119 ) ) ;
#19658=VERTEX_POINT ( 'NONE', #37910 ) ;
#19659=ORIENTED_EDGE ( 'NONE', *, *, #4484, .T. ) ;
#19672=AXIS2_PLACEMENT_3D ( 'NONE', #1196, #14243, #60498 ) ;
#19683=CARTESIAN_POINT ( 'NONE',  ( -0.03998971805478993002, 1.064647760289955114, -1.632685650884892370 ) ) ;
#19710=CARTESIAN_POINT ( 'NONE',  ( -3.913926014577544521, 1.327547550174811741, -0.4257567319240657122 ) ) ;
#19717=LINE ( 'NONE', #63505, #75424 ) ;
#19724=ADVANCED_FACE ( 'NONE', ( #11433 ), #11015, .F. ) ;
#19730=DIRECTION ( 'NONE',  ( 0.000000000000000000, 0.000000000000000000, -1.000000000000000000 ) ) ;
#19748=ADVANCED_FACE ( 'NONE', ( #76232 ), #57160, .T. ) ;
#19753=ORIENTED_EDGE ( 'NONE', *, *, #48374, .T. ) ;
#19755=CARTESIAN_POINT ( 'NONE',  ( 2.704370107879210838, 1.253873987468413498, -0.3814095263789911150 ) ) ;
#19758=EDGE_CURVE ( 'NONE', #15966, #33945, #43792, .T. ) ;
#19785=ADVANCED_FACE ( 'NONE', ( #62348 ), #76635, .F. ) ;
#19786=LINE ( 'NONE', #858, #74909 ) ;
#19821=LINE ( 'NONE', #45047, #44729 ) ;
#19828=EDGE_CURVE ( 'NONE', #64046, #79730, #21048, .T. ) ;
#19829=CARTESIAN_POINT ( 'NONE',  ( 1.141392835773559211, 0.3937007874015747699, 1.141392835773562764 ) ) ;
#19834=CARTESIAN_POINT ( 'NONE',  ( -0.4359958488159583201, 1.724409448818897905, -3.912791665790201101 ) ) ;
#19861=AXIS2_PLACEMENT_3D ( 'NONE', #37915, #69090, #56441 ) ;
#19876=CARTESIAN_POINT ( 'NONE',  ( 1.348312163386739426, 0.2755905511811023723, 0.7386866130305692613 ) ) ;
#19907=CARTESIAN_POINT ( 'NONE',  ( -0.4562095852119795736, 1.668416680336018976, 2.129998074986525047 ) ) ;
#19919=CARTESIAN_POINT ( 'NONE',  ( 0.3462686196234177061, 1.212745639448218116, 3.921766127980873762 ) ) ;
#19971=VERTEX_POINT ( 'NONE', #2075 ) ;
#19977=CARTESIAN_POINT ( 'NONE',  ( -0.2642730939577113136, 1.143123705106231736, 2.800754169703324692 ) ) ;
#19978=CARTESIAN_POINT ( 'NONE',  ( -0.4359958488159755841, 1.724409448818897905, 1.033875059083675163 ) ) ;
#19983=FACE_OUTER_BOUND ( 'NONE', #37685, .T. ) ;
#19986=ORIENTED_EDGE ( 'NONE', *, *, #63016, .F. ) ;
#19987=CARTESIAN_POINT ( 'NONE',  ( 0.000000000000000000, 0.4374015748031496176, 0.000000000000000000 ) ) ;
#19988=CARTESIAN_POINT ( 'NONE',  ( 0.3149606299212484029, 2.559055118110236560, 1.076935383196061080 ) ) ;
#19993=VERTEX_POINT ( 'NONE', #7562 ) ;
#20018=CARTESIAN_POINT ( 'NONE',  ( -0.5314960629921194890, 2.716535433070866645, -1.854472803289054283 ) ) ;
#20037=CARTESIAN_POINT ( 'NONE',  ( 0.2538623822092395677, 1.136619844641765242, -1.626743363757151117 ) ) ;
#20050=ORIENTED_EDGE ( 'NONE', *, *, #77818, .T. ) ;
#20068=VERTEX_POINT ( 'NONE', #71951 ) ;
#20075=VECTOR ( 'NONE', #49151, 39.37007874015748143 ) ;
#20087=ORIENTED_EDGE ( 'NONE', *, *, #80969, .F. ) ;
#20094=CARTESIAN_POINT ( 'NONE',  ( 1.901964908973707402, 1.119136672863562776, 0.2244172274865111338 ) ) ;
#20102=CARTESIAN_POINT ( 'NONE',  ( 0.000000000000000000, 2.716535433070866645, 0.000000000000000000 ) ) ;
#20106=B_SPLINE_CURVE_WITH_KNOTS ( 'NONE', 3,
 ( #48749, #74448, #34900, #42431 ),
 .UNSPECIFIED., .F., .F.,
 ( 4, 4 ),
 ( 0.07469576999304926301, 0.07612553241189917719 ),
 .UNSPECIFIED. ) ;
#20142=EDGE_LOOP ( 'NONE', ( #30006, #31811, #64028, #70677 ) ) ;
#20151=CARTESIAN_POINT ( 'NONE',  ( 0.2895944160946348211, 1.160344800674453003, -3.926428547179232620 ) ) ;
#20157=EDGE_LOOP ( 'NONE', ( #20087, #58886, #37034, #50984 ) ) ;
#20171=ORIENTED_EDGE ( 'NONE', *, *, #65042, .F. ) ;
#20174=CARTESIAN_POINT ( 'NONE',  ( 2.723203318070475998, 1.231544801320231919, -0.3638227417423834931 ) ) ;
#20207=DIRECTION ( 'NONE',  ( 0.000000000000000000, -0.6427876096865389188, -0.7660444431189783465 ) ) ;
#20213=EDGE_CURVE ( 'NONE', #9504, #76474, #4934, .T. ) ;
#20246=CARTESIAN_POINT ( 'NONE',  ( -3.937007874015748143, 2.755905511811024056, -0.5314960629921260393 ) ) ;
#20255=ORIENTED_EDGE ( 'NONE', *, *, #29420, .F. ) ;
#20275=ORIENTED_EDGE ( 'NONE', *, *, #55345, .T. ) ;
#20286=CARTESIAN_POINT ( 'NONE',  ( 1.141392835773559211, 1.299212598425196985, 0.9642274814428540841 ) ) ;
#20287=AXIS2_PLACEMENT_3D ( 'NONE', #76563, #37834, #18891 ) ;
#20290=CARTESIAN_POINT ( 'NONE',  ( 0.4359958488159816348, 1.724409448818897905, -2.630268417803909298 ) ) ;
#20293=CARTESIAN_POINT ( 'NONE',  ( 3.912467585512841239, 1.355617292003078012, -0.4390143889087900209 ) ) ;
#20338=PLANE ( 'NONE',  #54696 ) ;
#20343=VECTOR ( 'NONE', #40496, 39.37007874015748143 ) ;
#20368=CARTESIAN_POINT ( 'NONE',  ( 0.4620977091643874712, 1.428887118379093435, 1.022480879491282968 ) ) ;
#20383=AXIS2_PLACEMENT_3D ( 'NONE', #23804, #12012, #70066 ) ;
#20387=ORIENTED_EDGE ( 'NONE', *, *, #53209, .T. ) ;
#20392=LINE ( 'NONE', #33849, #7510 ) ;
#20393=CARTESIAN_POINT ( 'NONE',  ( -0.1179898944395515598, 1.077592634160693841, 2.860510421453457575 ) ) ;
#20394=DIRECTION ( 'NONE',  ( 0.000000000000000000, 0.000000000000000000, 1.000000000000000000 ) ) ;
#20406=DIRECTION ( 'NONE',  ( -0.000000000000000000, -1.000000000000000000, -0.000000000000000000 ) ) ;
#20414=DIRECTION ( 'NONE',  ( 8.659560562354947649E-17, -0.7071067811865462405, 0.7071067811865486830 ) ) ;
#20438=DIRECTION ( 'NONE',  ( 0.000000000000000000, 0.000000000000000000, -1.000000000000000000 ) ) ;
#20457=EDGE_CURVE ( 'NONE', #15514, #13252, #27628, .T. ) ;
#20460=CARTESIAN_POINT ( 'NONE',  ( 0.3798529523383403772, 1.251889725672750142, -1.733216647067249427 ) ) ;
#20472=ORIENTED_EDGE ( 'NONE', *, *, #28057, .T. ) ;
#20489=VERTEX_POINT ( 'NONE', #68125 ) ;
#20500=CARTESIAN_POINT ( 'NONE',  ( 3.937007874015748143, 1.537401574803149984, 2.901595197523589142E-16 ) ) ;
#20506=ORIENTED_EDGE ( 'NONE', *, *, #16133, .T. ) ;
#20507=ORIENTED_EDGE ( 'NONE', *, *, #43446, .T. ) ;
#20509=AXIS2_PLACEMENT_3D ( 'NONE', #22422, #3477, #29145 ) ;
#20514=DIRECTION ( 'NONE',  ( -1.408710688920637755E-15, 1.000000000000000000, -4.918487082195260922E-30 ) ) ;
#20527=CARTESIAN_POINT ( 'NONE',  ( -3.912791665790199769, 1.724409448818897905, -0.4359958488159722534 ) ) ;
#20557=CARTESIAN_POINT ( 'NONE',  ( -3.908320185825792326, 1.537401574803149984, -0.4744094488188975722 ) ) ;
#20559=CARTESIAN_POINT ( 'NONE',  ( 0.4177787735907000921, 0.3937007874015748254, -1.244210979442979648 ) ) ;
#20562=AXIS2_PLACEMENT_3D ( 'NONE', #75180, #76812, #17524 ) ;
#20565=CARTESIAN_POINT ( 'NONE',  ( 0.4418045515502986298, 1.710866862483978679, -2.620820774047688317 ) ) ;
#20573=CARTESIAN_POINT ( 'NONE',  ( 0.3858746366555774188, 1.260986746289878502, -3.918061586339389724 ) ) ;
#20574=CARTESIAN_POINT ( 'NONE',  ( 3.869764100875850765, 2.739927440807262471, 0.5314960629921260393 ) ) ;
#20577=EDGE_LOOP ( 'NONE', ( #53572, #56273, #19310, #7884 ) ) ;
#20591=EDGE_LOOP ( 'NONE', ( #39753, #28787, #77116, #28456 ) ) ;
#20593=ORIENTED_EDGE ( 'NONE', *, *, #42203, .F. ) ;
#20596=CARTESIAN_POINT ( 'NONE',  ( 2.554859668665111272, 1.520054044952884098, 0.4741688556381182251 ) ) ;
#20603=DIRECTION ( 'NONE',  ( 0.000000000000000000, 0.000000000000000000, -1.000000000000000000 ) ) ;
#20605=CONICAL_SURFACE ( 'NONE', #11172, 0.1190944881889763746, 0.8726646259971653219 ) ;
#20627=LINE ( 'NONE', #45438, #6328 ) ;
#20636=DIRECTION ( 'NONE',  ( 0.000000000000000000, 0.000000000000000000, 1.000000000000000000 ) ) ;
#20648=ADVANCED_FACE ( 'NONE', ( #73620 ), #42018, .F. ) ;
#20668=CARTESIAN_POINT ( 'NONE',  ( -0.4498537592782897998, 0.000000000000000000, -2.118110236220472675 ) ) ;
#20678=CONICAL_SURFACE ( 'NONE', #31405, 2.559055118110236560, 0.7853981633974500554 ) ;
#20692=DIRECTION ( 'NONE',  ( 0.000000000000000000, 1.000000000000000000, -0.000000000000000000 ) ) ;
#20698=B_SPLINE_CURVE_WITH_KNOTS ( 'NONE', 3,
 ( #27657, #79861, #21351, #47004, #22178, #72698, #17940, #29318, #49903, #23000, #10392, #9965 ),
 .UNSPECIFIED., .F., .F.,
 ( 4, 2, 2, 2, 2, 4 ),
 ( 0.05454303362711770270, 0.05585633982237129397, 0.05651299291999809654, 0.05716964601762489911, 0.05848295221287848344, 0.05979625840813206777 ),
 .UNSPECIFIED. ) ;
#20714=CARTESIAN_POINT ( 'NONE',  ( 3.923605715242195480, 1.191231191135928791, -0.3247605523133955674 ) ) ;
#20726=VECTOR ( 'NONE', #64680, 39.37007874015748143 ) ;
#20740=CARTESIAN_POINT ( 'NONE',  ( 1.374111565972423831E-16, 0.4374015748031496176, -1.122047244094488194 ) ) ;
#20743=CIRCLE ( 'NONE', #4567, 0.5118110236220472231 ) ;
#20760=CARTESIAN_POINT ( 'NONE',  ( -3.197598481144914739, 2.742783271388837374, 0.5314960629921260393 ) ) ;
#20785=CARTESIAN_POINT ( 'NONE',  ( 0.3136779242486383290, 1.181160616066996294, 1.077380321234679084 ) ) ;
#20810=CARTESIAN_POINT ( 'NONE',  ( -0.1807843743677566839, 1.098495470880701985, 2.841284648355170361 ) ) ;
#20817=EDGE_LOOP ( 'NONE', ( #5154, #83226, #4631, #63824 ) ) ;
#20819=CARTESIAN_POINT ( 'NONE',  ( -1.077529977636055181, 1.180708531484368162, -0.3131643582486707267 ) ) ;
#20822=DIRECTION ( 'NONE',  ( 0.000000000000000000, 0.000000000000000000, 1.000000000000000000 ) ) ;
#20826=ORIENTED_EDGE ( 'NONE', *, *, #82082, .F. ) ;
#20827=DIRECTION ( 'NONE',  ( 0.000000000000000000, 0.000000000000000000, 1.000000000000000000 ) ) ;
#20837=EDGE_CURVE ( 'NONE', #2386, #71433, #59828, .T. ) ;
#20844=CARTESIAN_POINT ( 'NONE',  ( 2.503252890251015828, 2.755905511811024056, 0.5314960629921260393 ) ) ;
#20850=AXIS2_PLACEMENT_3D ( 'NONE', #82305, #50701, #12420 ) ;
#20860=EDGE_LOOP ( 'NONE', ( #57915, #71415, #65518, #1553 ) ) ;
#20861=B_SPLINE_CURVE_WITH_KNOTS ( 'NONE', 3,
 ( #51834, #64903, #32914, #40068, #65755, #71637, #26603, #1769, #13153, #8502, #59413, #8088, #27851, #70800, #945, #33752 ),
 .UNSPECIFIED., .F., .F.,
 ( 4, 2, 2, 2, 2, 2, 2, 4 ),
 ( 0.000000000000000000, 0.0003923911760484576224, 0.0007847823520969152448, 0.001177173528145373030, 0.001569564704193830490, 0.001961955880242287949, 0.002354347056290746060, 0.003139129408387677025 ),
 .UNSPECIFIED. ) ;
#20875=EDGE_CURVE ( 'NONE', #55882, #11181, #2601, .T. ) ;
#20877=CARTESIAN_POINT ( 'NONE',  ( 0.3025936627584911998, 1.171974003123068542, -1.693908891378735015 ) ) ;
#20906=VERTEX_POINT ( 'NONE', #5299 ) ;
#20916=CARTESIAN_POINT ( 'NONE',  ( 0.5314960629920847390, 2.755905511811024056, 3.937007874015794773 ) ) ;
#20928=DIRECTION ( 'NONE',  ( 1.000000000000000000, 1.460819769243627131E-15, 0.000000000000000000 ) ) ;
#20936=EDGE_CURVE ( 'NONE', #27207, #9799, #74364, .T. ) ;
#20941=CARTESIAN_POINT ( 'NONE',  ( 3.912791665790199769, 1.724409448818897905, -0.4359958488159719758 ) ) ;
#20974=DIRECTION ( 'NONE',  ( 0.000000000000000000, 1.000000000000000000, 0.000000000000000000 ) ) ;
#20988=ORIENTED_EDGE ( 'NONE', *, *, #72187, .F. ) ;
#21004=AXIS2_PLACEMENT_3D ( 'NONE', #14938, #2718, #28378 ) ;
#21009=CARTESIAN_POINT ( 'NONE',  ( -1.413425744192504663, 1.183688739992415417, 0.3163780376571070363 ) ) ;
#21025=B_SPLINE_CURVE_WITH_KNOTS ( 'NONE', 3,
 ( #77221, #1457, #32596, #77645, #26279, #52356, #51940, #20393, #64178, #19550, #20810, #78063, #27114, #19134, #19977, #45628, #52777, #46465, #57837, #25858, #59102, #46046, #72159, #7775, #44783, #70480, #14514, #65851, #40167, #8184, #14094, #45209 ),
 .UNSPECIFIED., .F., .F.,
 ( 4, 2, 2, 2, 2, 2, 2, 2, 2, 2, 2, 2, 2, 2, 2, 4 ),
 ( 0.03390883336407149451, 0.03455365212229168786, 0.03519847088051188816, 0.03648810839695228181, 0.03777774591339266852, 0.03906738342983306217, 0.04035702094627344888, 0.04164665846271384253, 0.04422593349559461595, 0.04680520852847537550, 0.04938448356135614198, 0.05067412107779653563, 0.05196375859423692234, 0.05325339611067732293, 0.05389821486889750934, 0.05454303362711770270 ),
 .UNSPECIFIED. ) ;
#21048=B_SPLINE_CURVE_WITH_KNOTS ( 'NONE', 3,
 ( #81734, #82139, #82953, #69498, #50526, #75819, #38325, #55608, #18966, #44615, #63998, #43384, #17351, #37500, #4686, #5922, #81319, #25271, #49303, #24043, #69899, #68674, #31594, #17754, #57250, #75004, #42979, #14348, #45459, #53023 ),
 .UNSPECIFIED., .F., .F.,
 ( 4, 2, 2, 2, 2, 2, 2, 2, 2, 2, 2, 2, 2, 2, 4 ),
 ( 0.005313729678161706153, 0.005969797177609010609, 0.006625864677056315065, 0.007937999675950898823, 0.009250134674845481714, 0.01056226967374006634, 0.01318653967152924947, 0.01581080966931843260, 0.01712294466821301375, 0.01843507966710759144, 0.02105934966489676416, 0.02237148466379134532, 0.02368361966268592647, 0.02499575466158050763, 0.02630788966047508878 ),
 .UNSPECIFIED. ) ;
#21061=AXIS2_PLACEMENT_3D ( 'NONE', #40510, #8114, #65367 ) ;
#21066=AXIS2_PLACEMENT_3D ( 'NONE', #51903, #71286, #73266 ) ;
#21075=DIRECTION ( 'NONE',  ( -3.736327486719276758E-15, 0.000000000000000000, -1.000000000000000000 ) ) ;
#21082=CARTESIAN_POINT ( 'NONE',  ( 1.403614904275686858E-14, 1.537401574803149984, -3.937007874015761910 ) ) ;
#21089=VERTEX_POINT ( 'NONE', #73516 ) ;
#21092=ORIENTED_EDGE ( 'NONE', *, *, #49427, .F. ) ;
#21098=CARTESIAN_POINT ( 'NONE',  ( 0.03198557873782978400, 1.064015804215618699, -1.607980685227602402 ) ) ;
#21102=B_SPLINE_CURVE_WITH_KNOTS ( 'NONE', 3,
 ( #78605, #57953, #77762, #33554, #58808, #741, #46166, #45328, #32713, #44898, #71023, #1578 ),
 .UNSPECIFIED., .F., .F.,
 ( 4, 2, 2, 2, 2, 4 ),
 ( 0.05454303362711723779, 0.05585633982237087070, 0.05651299291999767327, 0.05716964601762447584, 0.05848295221287810874, 0.05979625840813173471 ),
 .UNSPECIFIED. ) ;
#21105=CARTESIAN_POINT ( 'NONE',  ( 0.5314960629921349211, 2.742779986175213569, -2.570293859026649308 ) ) ;
#21107=CARTESIAN_POINT ( 'NONE',  ( -0.4044922606986716129, 1.289103360985772495, -2.048376007908625507 ) ) ;
#21108=VERTEX_POINT ( 'NONE', #46979 ) ;
#21111=ORIENTED_EDGE ( 'NONE', *, *, #60327, .F. ) ;
#21122=DIRECTION ( 'NONE',  ( 0.000000000000000000, -0.5150380749100549327, -0.8571673007021117785 ) ) ;
#21150=LINE ( 'NONE', #47636, #48429 ) ;
#21158=CARTESIAN_POINT ( 'NONE',  ( -0.5314960629921148261, 2.755905511811024056, -3.184294706754632109 ) ) ;
#21167=CARTESIAN_POINT ( 'NONE',  ( 0.3765318260368863412, 1.248382286832529831, 3.918973582884354823 ) ) ;
#21200=CARTESIAN_POINT ( 'NONE',  ( 0.4582162924217514921, 1.413519198382197306, 1.024232834668445724 ) ) ;
#21222=CARTESIAN_POINT ( 'NONE',  ( 2.503252890251015828, 2.755905511811024056, 0.5314960629921260393 ) ) ;
#21230=ORIENTED_EDGE ( 'NONE', *, *, #6995, .F. ) ;
#21232=CARTESIAN_POINT ( 'NONE',  ( -1.096643835343520168, 1.126359415431272382, -0.2388483330940451010 ) ) ;
#21239=AXIS2_PLACEMENT_3D ( 'NONE', #50125, #82144, #32431 ) ;
#21253=EDGE_CURVE ( 'NONE', #6920, #24806, #12039, .T. ) ;
#21274=ORIENTED_EDGE ( 'NONE', *, *, #83070, .T. ) ;
#21276=EDGE_CURVE ( 'NONE', #64597, #43450, #61225, .T. ) ;
#21285=EDGE_CURVE ( 'NONE', #7122, #32917, #22155, .T. ) ;
#21301=VERTEX_POINT ( 'NONE', #75988 ) ;
#21302=ORIENTED_EDGE ( 'NONE', *, *, #12502, .F. ) ;
#21318=EDGE_LOOP ( 'NONE', ( #35521, #69428, #68534, #45200 ) ) ;
#21321=CARTESIAN_POINT ( 'NONE',  ( -1.438119991934921238, 1.333025515147837403, 0.4284971980842492423 ) ) ;
#21327=EDGE_CURVE ( 'NONE', #76797, #60402, #42325, .T. ) ;
#21338=VERTEX_POINT ( 'NONE', #30534 ) ;
#21344=CARTESIAN_POINT ( 'NONE',  ( 1.850582881112983635, 1.063196196511240199, -0.01636564761925528647 ) ) ;
#21351=CARTESIAN_POINT ( 'NONE',  ( -0.4734416007054501607, 1.572145545125846144, 2.556694656352222594 ) ) ;
#21367=CARTESIAN_POINT ( 'NONE',  ( 0.4255982601316013469, 1.327156923586373161, -1.428513422047406944 ) ) ;
#21369=DIRECTION ( 'NONE',  ( -1.000000000000000000, 0.000000000000000000, 0.000000000000000000 ) ) ;
#21377=ORIENTED_EDGE ( 'NONE', *, *, #1933, .F. ) ;
#21383=CARTESIAN_POINT ( 'NONE',  ( -3.913197263145800520, 1.341570523813770954, -0.4323813531989676995 ) ) ;
#21389=CARTESIAN_POINT ( 'NONE',  ( -3.856579543051780856, 2.748002881374839390, -0.5314960629921259283 ) ) ;
#21398=CARTESIAN_POINT ( 'NONE',  ( -2.516666458577628163, 2.742784436987529606, -0.5314960629921260393 ) ) ;
#21399=CARTESIAN_POINT ( 'NONE',  ( 3.900966923095589678, 2.677165354330708791, 0.5314960629921260393 ) ) ;
#21402=ORIENTED_EDGE ( 'NONE', *, *, #81194, .F. ) ;
#21419=VERTEX_POINT ( 'NONE', #35613 ) ;
#21421=EDGE_LOOP ( 'NONE', ( #17465, #803, #22546, #76661 ) ) ;
#21424=CARTESIAN_POINT ( 'NONE',  ( 2.800975763475996860, 1.142877263639039853, 0.2639061591570066589 ) ) ;
#21462=CARTESIAN_POINT ( 'NONE',  ( -0.5314960629921124946, 2.746034003362847198, -3.861376881555341978 ) ) ;
#21480=DIRECTION ( 'NONE',  ( 0.000000000000000000, -0.9925461516413219831, -0.1218693434051477398 ) ) ;
#21499=EDGE_CURVE ( 'NONE', #32355, #20489, #61276, .T. ) ;
#21501=ORIENTED_EDGE ( 'NONE', *, *, #6391, .F. ) ;
#21510=CARTESIAN_POINT ( 'NONE',  ( -0.4603218807116740141, 1.653261878685372777, -2.586075122629556411 ) ) ;
#21522=ORIENTED_EDGE ( 'NONE', *, *, #54718, .F. ) ;
#21539=DIRECTION ( 'NONE',  ( 0.000000000000000000, 0.000000000000000000, -1.000000000000000000 ) ) ;
#21555=DIRECTION ( 'NONE',  ( -0.000000000000000000, 1.000000000000000000, -0.000000000000000000 ) ) ;
#21562=DIRECTION ( 'NONE',  ( 0.000000000000000000, 0.000000000000000000, -1.000000000000000000 ) ) ;
#21571=DIRECTION ( 'NONE',  ( 0.000000000000000000, -1.000000000000000000, 0.000000000000000000 ) ) ;
#21574=CARTESIAN_POINT ( 'NONE',  ( 0.1818524038564936218, 1.098415106551606346, 3.932883554691550376 ) ) ;
#21588=DIRECTION ( 'NONE',  ( -0.000000000000000000, -1.000000000000000000, -0.000000000000000000 ) ) ;
#21602=VECTOR ( 'NONE', #22735, 39.37007874015748143 ) ;
#21610=CARTESIAN_POINT ( 'NONE',  ( 2.362204724409448620, 1.929133858267716661, 8.247593713802677664E-15 ) ) ;
#21629=VERTEX_POINT ( 'NONE', #5273 ) ;
#21631=VERTEX_POINT ( 'NONE', #24210 ) ;
#21634=CARTESIAN_POINT ( 'NONE',  ( 3.224202737261815166, 2.716535433070866645, -0.5314960629921260393 ) ) ;
#21651=ORIENTED_EDGE ( 'NONE', *, *, #15607, .T. ) ;
#21664=AXIS2_PLACEMENT_3D ( 'NONE', #5031, #5439, #57175 ) ;
#21682=CARTESIAN_POINT ( 'NONE',  ( -1.827151678354258069, 2.742788175498064529, 0.5314960629921260393 ) ) ;
#21684=ORIENTED_EDGE ( 'NONE', *, *, #73728, .T. ) ;
#21709=VERTEX_POINT ( 'NONE', #17920 ) ;
#21721=EDGE_CURVE ( 'NONE', #23879, #34573, #76198, .T. ) ;
#21736=CARTESIAN_POINT ( 'NONE',  ( -0.03443470937339728616, 0.2755905511811023723, -1.537015892239756099 ) ) ;
#21750=CARTESIAN_POINT ( 'NONE',  ( 1.867828664896292956, 1.081851677178494286, -0.1334749385307716363 ) ) ;
#21767=CIRCLE ( 'NONE', #39239, 3.937007874015748143 ) ;
#21795=CARTESIAN_POINT ( 'NONE',  ( -3.900966923095589678, 2.677165354330708791, -0.5314960629921260393 ) ) ;
#21808=ORIENTED_EDGE ( 'NONE', *, *, #73302, .F. ) ;
#21826=ORIENTED_EDGE ( 'NONE', *, *, #65042, .T. ) ;
#21845=EDGE_LOOP ( 'NONE', ( #57298, #22467, #76075, #8485 ) ) ;
#21871=CARTESIAN_POINT ( 'NONE',  ( 2.362204724409448620, 0.000000000000000000, 8.247593713802677664E-15 ) ) ;
#21878=AXIS2_PLACEMENT_3D ( 'NONE', #51328, #34919, #9658 ) ;
#21883=ADVANCED_FACE ( 'NONE', ( #63752 ), #12836, .F. ) ;
#21892=FACE_OUTER_BOUND ( 'NONE', #58336, .T. ) ;
#21898=LINE ( 'NONE', #2133, #42058 ) ;
#21902=B_SPLINE_CURVE_WITH_KNOTS ( 'NONE', 3,
 ( #30391, #18600, #3908, #69932 ),
 .UNSPECIFIED., .F., .F.,
 ( 4, 4 ),
 ( 0.1795298335526529787, 0.1809577925700027734 ),
 .UNSPECIFIED. ) ;
#21909=DIRECTION ( 'NONE',  ( -1.000000000000000000, 0.000000000000000000, -1.047444401652940480E-14 ) ) ;
#21910=DIRECTION ( 'NONE',  ( 1.734723475976807489E-15, 0.000000000000000000, -1.000000000000000000 ) ) ;
#21914=ORIENTED_EDGE ( 'NONE', *, *, #10296, .T. ) ;
#21918=ORIENTED_EDGE ( 'NONE', *, *, #15090, .T. ) ;
#21923=VECTOR ( 'NONE', #34936, 39.37007874015748143 ) ;
#21925=CARTESIAN_POINT ( 'NONE',  ( 0.01745729623385432541, 1.063258500840309706, -1.453357034165985828 ) ) ;
#21956=CARTESIAN_POINT ( 'NONE',  ( 3.908320185825791881, 1.537401574803149984, 0.4744094488188975722 ) ) ;
#21965=CARTESIAN_POINT ( 'NONE',  ( -0.6299212598425164567, 1.724409448818897905, -0.9285414500055737541 ) ) ;
#21981=ADVANCED_FACE ( 'NONE', ( #45627 ), #51516, .F. ) ;
#21986=VECTOR ( 'NONE', #60087, 39.37007874015748143 ) ;
#21993=DIRECTION ( 'NONE',  ( 0.000000000000000000, 1.000000000000000000, -0.000000000000000000 ) ) ;
#22007=FACE_OUTER_BOUND ( 'NONE', #19625, .T. ) ;
#22009=DIRECTION ( 'NONE',  ( -0.000000000000000000, 1.000000000000000000, -0.000000000000000000 ) ) ;
#22014=VERTEX_POINT ( 'NONE', #26278 ) ;
#22027=DIRECTION ( 'NONE',  ( 0.000000000000000000, 0.000000000000000000, 1.000000000000000000 ) ) ;
#22028=DIRECTION ( 'NONE',  ( 0.000000000000000000, 0.000000000000000000, 1.000000000000000000 ) ) ;
#22044=CARTESIAN_POINT ( 'NONE',  ( -0.4359958488159582091, 1.724409448818897905, -3.937007874015763687 ) ) ;
#22047=ORIENTED_EDGE ( 'NONE', *, *, #55030, .F. ) ;
#22050=DIRECTION ( 'NONE',  ( -0.000000000000000000, -1.000000000000000000, -0.000000000000000000 ) ) ;
#22051=FACE_OUTER_BOUND ( 'NONE', #66881, .T. ) ;
#22053=VECTOR ( 'NONE', #13912, 39.37007874015749564 ) ;
#22058=ORIENTED_EDGE ( 'NONE', *, *, #26365, .T. ) ;
#22060=CARTESIAN_POINT ( 'NONE',  ( -1.120715528315120002, 1.066117147761049821, 0.06272875519749153417 ) ) ;
#22066=DIRECTION ( 'NONE',  ( 0.000000000000000000, 0.000000000000000000, -1.000000000000000000 ) ) ;
#22069=DIRECTION ( 'NONE',  ( -0.000000000000000000, 1.000000000000000000, -0.000000000000000000 ) ) ;
#22073=EDGE_CURVE ( 'NONE', #33549, #17115, #8898, .T. ) ;
#22085=CARTESIAN_POINT ( 'NONE',  ( -0.6299212598425059095, 1.724409448818897905, -3.937007874015764131 ) ) ;
#22098=AXIS2_PLACEMENT_3D ( 'NONE', #9136, #2406, #28064 ) ;
#22100=DIRECTION ( 'NONE',  ( 1.000000000000000000, 0.000000000000000000, 3.455050906509825972E-15 ) ) ;
#22102=EDGE_LOOP ( 'NONE', ( #9225, #47181, #19433, #49575 ) ) ;
#22131=ORIENTED_EDGE ( 'NONE', *, *, #72797, .T. ) ;
#22137=CARTESIAN_POINT ( 'NONE',  ( 1.348312163386739426, 0.2755905511811023723, 0.8577811012195456497 ) ) ;
#22148=ORIENTED_EDGE ( 'NONE', *, *, #33639, .T. ) ;
#22151=DIRECTION ( 'NONE',  ( -1.000000000000000000, -0.000000000000000000, -0.000000000000000000 ) ) ;
#22155=LINE ( 'NONE', #56604, #77376 ) ;
#22166=ORIENTED_EDGE ( 'NONE', *, *, #4970, .T. ) ;
#22168=PLANE ( 'NONE',  #17865 ) ;
#22170=CARTESIAN_POINT ( 'NONE',  ( 1.901586028222546521, 1.118719813955014741, -0.2236424093447257344 ) ) ;
#22177=CARTESIAN_POINT ( 'NONE',  ( -1.313877454013331780, 0.000000000000000000, 0.7983292792091805090 ) ) ;
#22178=CARTESIAN_POINT ( 'NONE',  ( -0.4695140184743471501, 1.605872332714552542, 2.565964038698629768 ) ) ;
#22181=AXIS2_PLACEMENT_3D ( 'NONE', #10265, #78902, #73411 ) ;
#22191=B_SPLINE_CURVE_WITH_KNOTS ( 'NONE', 3,
 ( #57981, #32319, #346, #52500, #32739, #72308, #78209, #26841 ),
 .UNSPECIFIED., .F., .F.,
 ( 4, 2, 2, 4 ),
 ( 0.000000000000000000, 0.002441020876198872046, 0.003661531314298308287, 0.004882041752397744960 ),
 .UNSPECIFIED. ) ;
#22199=B_SPLINE_CURVE_WITH_KNOTS ( 'NONE', 3,
 ( #27325, #59312, #27746, #26071, #77432, #45420, #52985, #13459, #46682, #39116, #8396, #72375 ),
 .UNSPECIFIED., .F., .F.,
 ( 4, 2, 2, 2, 2, 4 ),
 ( 0.007992874908875674880, 0.009303755029337829399, 0.01061463514979998392, 0.01192551527026214017, 0.01258095533049322090, 0.01323639539072430336 ),
 .UNSPECIFIED. ) ;
#22201=DIRECTION ( 'NONE',  ( -3.491481338843132961E-15, -0.000000000000000000, 1.000000000000000000 ) ) ;
#22227=VECTOR ( 'NONE', #80088, 39.37007874015748143 ) ;
#22245=ORIENTED_EDGE ( 'NONE', *, *, #43710, .F. ) ;
#22250=CARTESIAN_POINT ( 'NONE',  ( -0.4744094488189106174, 1.537401574803149984, 3.908320185825790105 ) ) ;
#22263=DIRECTION ( 'NONE',  ( 0.000000000000000000, 0.000000000000000000, 1.000000000000000000 ) ) ;
#22264=ORIENTED_EDGE ( 'NONE', *, *, #73388, .F. ) ;
#22290=CARTESIAN_POINT ( 'NONE',  ( 0.5314960629920851831, 2.725289161120230563, 3.884611959489594035 ) ) ;
#22298=CARTESIAN_POINT ( 'NONE',  ( -3.937007874015748143, 2.165354330708661568, 0.6299212598425196763 ) ) ;
#22317=CARTESIAN_POINT ( 'NONE',  ( 0.000000000000000000, 1.724409448818897461, 0.000000000000000000 ) ) ;
#22318=ORIENTED_EDGE ( 'NONE', *, *, #6995, .T. ) ;
#22333=ORIENTED_EDGE ( 'NONE', *, *, #49427, .T. ) ;
#22348=CARTESIAN_POINT ( 'NONE',  ( 0.03411923929626541063, 1.063910482648552369, -2.873164143118426495 ) ) ;
#22351=VERTEX_POINT ( 'NONE', #39745 ) ;
#22354=EDGE_LOOP ( 'NONE', ( #27015, #43188, #61, #78956 ) ) ;
#22356=AXIS2_PLACEMENT_3D ( 'NONE', #50713, #76412, #58694 ) ;
#22379=B_SPLINE_CURVE_WITH_KNOTS ( 'NONE', 3,
 ( #61346, #21398, #27707, #47880 ),
 .UNSPECIFIED., .F., .F.,
 ( 4, 4 ),
 ( 0.1658669167714240389, 0.1672512987629738990 ),
 .UNSPECIFIED. ) ;
#22383=FACE_OUTER_BOUND ( 'NONE', #59815, .T. ) ;
#22390=CARTESIAN_POINT ( 'NONE',  ( -0.2774512451045073602, 1.152276239669946856, -1.087282494290732870 ) ) ;
#22392=CARTESIAN_POINT ( 'NONE',  ( 0.000000000000000000, 2.559055118110236560, 0.000000000000000000 ) ) ;
#22393=EDGE_CURVE ( 'NONE', #43641, #70804, #15642, .T. ) ;
#22396=VECTOR ( 'NONE', #61716, 39.37007874015748143 ) ;
#22398=AXIS2_PLACEMENT_3D ( 'NONE', #23363, #54515, #54097 ) ;
#22408=EDGE_CURVE ( 'NONE', #47922, #21629, #12156, .T. ) ;
#22409=CARTESIAN_POINT ( 'NONE',  ( -0.02865809819635581693, 1.063823086577868615, -1.634058138423551076 ) ) ;
#22422=CARTESIAN_POINT ( 'NONE',  ( 0.000000000000000000, 2.755905511811024056, 0.000000000000000000 ) ) ;
#22426=CARTESIAN_POINT ( 'NONE',  ( 2.161121219943137106, 1.597527518877484676, -0.4706608522957222984 ) ) ;
#22431=VERTEX_POINT ( 'NONE', #21222 ) ;
#22440=CIRCLE ( 'NONE', #54691, 0.09842519685039365085 ) ;
#22450=AXIS2_PLACEMENT_3D ( 'NONE', #18220, #44268, #5574 ) ;
#22453=EDGE_CURVE ( 'NONE', #36503, #68098, #42459, .T. ) ;
#22463=CARTESIAN_POINT ( 'NONE',  ( -0.06838555148300114184, 1.067631514832608319, -2.869717892578235841 ) ) ;
#22467=ORIENTED_EDGE ( 'NONE', *, *, #31058, .T. ) ;
#22478=ORIENTED_EDGE ( 'NONE', *, *, #29420, .T. ) ;
#22503=AXIS2_PLACEMENT_3D ( 'NONE', #51887, #71268, #26650 ) ;
#22504=CARTESIAN_POINT ( 'NONE',  ( 1.141392835773559211, 0.3937007874015747699, 0.9435581901042713326 ) ) ;
#22516=CARTESIAN_POINT ( 'NONE',  ( 0.008542603271838917003, 1.062992125984252745, 1.850393700787401619 ) ) ;
#22546=ORIENTED_EDGE ( 'NONE', *, *, #76757, .F. ) ;
#22547=EDGE_CURVE ( 'NONE', #34953, #50774, #3113, .T. ) ;
#22554=LINE ( 'NONE', #22137, #8774 ) ;
#22565=ORIENTED_EDGE ( 'NONE', *, *, #30606, .F. ) ;
#22569=AXIS2_PLACEMENT_3D ( 'NONE', #48798, #54704, #47974 ) ;
#22586=CARTESIAN_POINT ( 'NONE',  ( 2.167277156196865118, 1.503024749832830853, -0.4732391302016644152 ) ) ;
#22592=FACE_OUTER_BOUND ( 'NONE', #13342, .T. ) ;
#22613=CARTESIAN_POINT ( 'NONE',  ( 3.224202737261815166, 2.716535433070866645, -0.5314960629921260393 ) ) ;
#22635=ADVANCED_FACE ( 'NONE', ( #47294 ), #61272, .F. ) ;
#22645=EDGE_CURVE ( 'NONE', #1571, #30834, #41411, .T. ) ;
#22662=LINE ( 'NONE', #55047, #28725 ) ;
#22702=EDGE_CURVE ( 'NONE', #66965, #54650, #20392, .T. ) ;
#22703=CARTESIAN_POINT ( 'NONE',  ( -1.867405098639518091, 1.081388112195859508, -0.1351566381869792888 ) ) ;
#22709=EDGE_CURVE ( 'NONE', #62412, #50709, #41150, .T. ) ;
#22729=ORIENTED_EDGE ( 'NONE', *, *, #70277, .F. ) ;
#22732=CARTESIAN_POINT ( 'NONE',  ( 0.2567756966273455066, 1.138473552315965032, -1.484942126512834859 ) ) ;
#22735=DIRECTION ( 'NONE',  ( -0.000000000000000000, -1.000000000000000000, -0.000000000000000000 ) ) ;
#22741=EDGE_LOOP ( 'NONE', ( #63011, #47825 ) ) ;
#22744=ORIENTED_EDGE ( 'NONE', *, *, #17348, .T. ) ;
#22750=CARTESIAN_POINT ( 'NONE',  ( 0.05679685702235415246, 1.066397369817506435, -1.517643113990623238 ) ) ;
#22755=CARTESIAN_POINT ( 'NONE',  ( 0.3230088838496886772, 1.189621120221110440, -2.759465352243644531 ) ) ;
#22773=DIRECTION ( 'NONE',  ( -1.000000000000000000, -0.000000000000000000, -0.000000000000000000 ) ) ;
#22790=DIRECTION ( 'NONE',  ( 0.000000000000000000, 0.000000000000000000, -1.000000000000000000 ) ) ;
#22797=CARTESIAN_POINT ( 'NONE',  ( -0.4588941285983808571, 1.412993309469693370, -1.023939894463827160 ) ) ;
#22798=EDGE_CURVE ( 'NONE', #77721, #39649, #62008, .T. ) ;
#22805=EDGE_CURVE ( 'NONE', #81379, #9709, #30430, .T. ) ;
#22816=CARTESIAN_POINT ( 'NONE',  ( -0.01122658826027363339, 1.063090000085920250, -1.632673439369667800 ) ) ;
#22831=LINE ( 'NONE', #29962, #62137 ) ;
#22832=DIRECTION ( 'NONE',  ( 0.000000000000000000, -1.000000000000000000, 0.000000000000000000 ) ) ;
#22833=CARTESIAN_POINT ( 'NONE',  ( 2.362204724409448620, 0.03937007874015751446, 8.247593713802677664E-15 ) ) ;
#22843=CARTESIAN_POINT ( 'NONE',  ( 3.900966923095587457, 2.682389230697235671, -0.5314960629921258173 ) ) ;
#22849=EDGE_CURVE ( 'NONE', #79084, #5432, #24111, .T. ) ;
#22873=EDGE_LOOP ( 'NONE', ( #69676, #929, #81343, #73256 ) ) ;
#22876=PLANE ( 'NONE',  #16257 ) ;
#22877=FACE_OUTER_BOUND ( 'NONE', #79391, .T. ) ;
#22879=CARTESIAN_POINT ( 'NONE',  ( 0.6299212598425341092, 1.724409448818898127, -3.937007874015759690 ) ) ;
#22880=CARTESIAN_POINT ( 'NONE',  ( 0.000000000000000000, 2.755905511811024056, 0.000000000000000000 ) ) ;
#22913=ADVANCED_FACE ( 'NONE', ( #22877 ), #80566, .F. ) ;
#22922=CARTESIAN_POINT ( 'NONE',  ( -0.4359958488159582091, 1.724409448818897905, -3.937007874015763687 ) ) ;
#22925=EDGE_CURVE ( 'NONE', #82069, #9892, #13211, .T. ) ;
#22926=CARTESIAN_POINT ( 'NONE',  ( -0.6299212598425230070, 2.165354330708661568, 0.9285414500055690912 ) ) ;
#22941=CARTESIAN_POINT ( 'NONE',  ( -2.543486866223389153, 2.716535433070866645, 0.5314960629921260393 ) ) ;
#22954=ORIENTED_EDGE ( 'NONE', *, *, #15339, .F. ) ;
#22956=EDGE_CURVE ( 'NONE', #61385, #10785, #51879, .T. ) ;
#22961=DIRECTION ( 'NONE',  ( -3.491481338843132961E-15, -0.000000000000000000, 1.000000000000000000 ) ) ;
#22990=ORIENTED_EDGE ( 'NONE', *, *, #41310, .T. ) ;
#22994=DIRECTION ( 'NONE',  ( -0.000000000000000000, -1.000000000000000000, 0.000000000000000000 ) ) ;
#23000=CARTESIAN_POINT ( 'NONE',  ( -0.4469779880792152382, 1.697109554835841916, 2.611722799339278200 ) ) ;
#23021=DIRECTION ( 'NONE',  ( 0.000000000000000000, -0.000000000000000000, 1.000000000000000000 ) ) ;
#23049=VERTEX_POINT ( 'NONE', #10263 ) ;
#23051=ORIENTED_EDGE ( 'NONE', *, *, #33188, .F. ) ;
#23074=CARTESIAN_POINT ( 'NONE',  ( 0.4678446894728544025, 1.617652276888540852, 1.019864652736552690 ) ) ;
#23089=DIRECTION ( 'NONE',  ( -0.000000000000000000, 1.000000000000000000, -0.000000000000000000 ) ) ;
#23111=CARTESIAN_POINT ( 'NONE',  ( -1.850582881112984746, 1.063196196511240865, 0.01636564761927281758 ) ) ;
#23130=DIRECTION ( 'NONE',  ( 0.000000000000000000, -0.000000000000000000, 1.000000000000000000 ) ) ;
#23136=ORIENTED_EDGE ( 'NONE', *, *, #16862, .T. ) ;
#23148=ORIENTED_EDGE ( 'NONE', *, *, #75249, .T. ) ;
#23166=VERTEX_POINT ( 'NONE', #29194 ) ;
#23207=CARTESIAN_POINT ( 'NONE',  ( 3.937007874015748143, 1.537401574803149984, 2.901595197523589142E-16 ) ) ;
#23238=CARTESIAN_POINT ( 'NONE',  ( 0.4177787735907000366, 1.299212598425196985, -1.736336963694947944 ) ) ;
#23240=CARTESIAN_POINT ( 'NONE',  ( -2.362204724409448620, 1.724409448818897905, 0.5118110236220224651 ) ) ;
#23241=CARTESIAN_POINT ( 'NONE',  ( 2.158445410120265695, 1.605872332714552986, -0.4695140184743379352 ) ) ;
#23248=VECTOR ( 'NONE', #15383, 39.37007874015748143 ) ;
#23277=CARTESIAN_POINT ( 'NONE',  ( -0.4122598602536396428, 1.300945800302086619, -2.666505492093648844 ) ) ;
#23283=ORIENTED_EDGE ( 'NONE', *, *, #35630, .F. ) ;
#23290=CARTESIAN_POINT ( 'NONE',  ( 2.362204724409448620, 0.03937007874015751446, 0.5118110236220555498 ) ) ;
#23306=CARTESIAN_POINT ( 'NONE',  ( 0.5314960629920851831, 2.559055118110236560, 3.900966923095595451 ) ) ;
#23311=AXIS2_PLACEMENT_3D ( 'NONE', #14490, #60330, #51913 ) ;
#23321=CARTESIAN_POINT ( 'NONE',  ( 0.4177787735906999811, 1.312623414240995157, -1.714017618091133288 ) ) ;
#23337=ADVANCED_FACE ( 'NONE', ( #62416 ), #73828, .F. ) ;
#23343=DIRECTION ( 'NONE',  ( 0.000000000000000000, 0.000000000000000000, 1.000000000000000000 ) ) ;
#23352=FACE_OUTER_BOUND ( 'NONE', #619, .T. ) ;
#23363=CARTESIAN_POINT ( 'NONE',  ( 0.000000000000000000, 0.000000000000000000, 0.000000000000000000 ) ) ;
#23372=DIRECTION ( 'NONE',  ( -3.491481338843132961E-15, -0.000000000000000000, 1.000000000000000000 ) ) ;
#23384=ORIENTED_EDGE ( 'NONE', *, *, #63827, .F. ) ;
#23392=EDGE_CURVE ( 'NONE', #76416, #2295, #73442, .T. ) ;
#23397=EDGE_CURVE ( 'NONE', #63914, #74015, #36740, .T. ) ;
#23416=CIRCLE ( 'NONE', #47563, 1.244489337948954555 ) ;
#23423=EDGE_CURVE ( 'NONE', #67465, #56386, #45144, .T. ) ;
#23435=VERTEX_POINT ( 'NONE', #56504 ) ;
#23437=EDGE_CURVE ( 'NONE', #78176, #73035, #39762, .T. ) ;
#23477=ORIENTED_EDGE ( 'NONE', *, *, #1370, .T. ) ;
#23485=CARTESIAN_POINT ( 'NONE',  ( -0.4478269029167694093, 1.694792223680989363, -3.911458217027259376 ) ) ;
#23486=AXIS2_PLACEMENT_3D ( 'NONE', #67925, #8599, #9018 ) ;
#23488=CARTESIAN_POINT ( 'NONE',  ( 0.4359958488159610956, 1.724409448818897461, 1.033875059083681158 ) ) ;
#23502=DIRECTION ( 'NONE',  ( -3.491481338843132961E-15, 0.000000000000000000, 1.000000000000000000 ) ) ;
#23521=CARTESIAN_POINT ( 'NONE',  ( -1.923433685342933241, 1.142877263639054286, 0.2639061591570278087 ) ) ;
#23552=CARTESIAN_POINT ( 'NONE',  ( -0.5314960629921122726, 2.559055118110236560, -3.937007874015763687 ) ) ;
#23555=CARTESIAN_POINT ( 'NONE',  ( 1.141392835773559211, 0.3937007874015748254, 1.141392835773562764 ) ) ;
#23568=DIRECTION ( 'NONE',  ( 0.000000000000000000, 0.000000000000000000, 1.000000000000000000 ) ) ;
#23573=DIRECTION ( 'NONE',  ( 0.000000000000000000, 1.000000000000000000, 0.000000000000000000 ) ) ;
#23579=EDGE_LOOP ( 'NONE', ( #45066, #18204, #73608, #5767 ) ) ;
#23609=DIRECTION ( 'NONE',  ( 0.000000000000000000, -1.000000000000000000, -0.000000000000000000 ) ) ;
#23613=DIRECTION ( 'NONE',  ( 0.000000000000000000, 0.000000000000000000, 1.000000000000000000 ) ) ;
#23616=CARTESIAN_POINT ( 'NONE',  ( -2.829418903715950062, 1.111478976311902400, -0.2095522481616286514 ) ) ;
#23650=CARTESIAN_POINT ( 'NONE',  ( 0.000000000000000000, 2.755905511811024056, 0.000000000000000000 ) ) ;
#23658=VERTEX_POINT ( 'NONE', #82206 ) ;
#23663=DIRECTION ( 'NONE',  ( -8.673617379884021667E-16, 1.000000000000000000, -3.028377322213054317E-30 ) ) ;
#23687=DIRECTION ( 'NONE',  ( 0.000000000000000000, -1.000000000000000000, 0.000000000000000000 ) ) ;
#23694=AXIS2_PLACEMENT_3D ( 'NONE', #41016, #39765, #27550 ) ;
#23697=AXIS2_PLACEMENT_3D ( 'NONE', #72263, #73088, #36027 ) ;
#23699=CARTESIAN_POINT ( 'NONE',  ( 0.5314960629921064994, 2.716535433070866645, 1.854472803289057836 ) ) ;
#23703=FILL_AREA_STYLE ('',( #11506 ) ) ;
#23727=DIRECTION ( 'NONE',  ( 0.000000000000000000, 0.000000000000000000, 1.000000000000000000 ) ) ;
#23748=CARTESIAN_POINT ( 'NONE',  ( 0.04294987210466596345, 1.064862614867414070, 1.852127137687914704 ) ) ;
#23757=CARTESIAN_POINT ( 'NONE',  ( -2.170146923806554273, 1.546132656481028489, -0.4744094488188974612 ) ) ;
#23761=CIRCLE ( 'NONE', #78881, 1.889763779527559251 ) ;
#23762=AXIS2_PLACEMENT_3D ( 'NONE', #49024, #73892, #67573 ) ;
#23768=DIRECTION ( 'NONE',  ( -0.000000000000000000, -1.000000000000000000, -0.000000000000000000 ) ) ;
#23803=DIRECTION ( 'NONE',  ( -0.000000000000000000, -1.000000000000000000, -0.000000000000000000 ) ) ;
#23804=CARTESIAN_POINT ( 'NONE',  ( 0.000000000000000000, 2.165354330708661568, 0.000000000000000000 ) ) ;
#23821=VECTOR ( 'NONE', #64817, 39.37007874015748143 ) ;
#23825=CIRCLE ( 'NONE', #25118, 1.122047244094488194 ) ;
#23826=LINE ( 'NONE', #62543, #55662 ) ;
#23873=AXIS2_PLACEMENT_3D ( 'NONE', #64036, #64875, #58554 ) ;
#23877=ORIENTED_EDGE ( 'NONE', *, *, #9959, .F. ) ;
#23879=VERTEX_POINT ( 'NONE', #40903 ) ;
#23889=ADVANCED_FACE ( 'NONE', ( #79642 ), #24961, .F. ) ;
#23894=VERTEX_POINT ( 'NONE', #77968 ) ;
#23901=DIRECTION ( 'NONE',  ( 0.000000000000000000, 0.000000000000000000, -1.000000000000000000 ) ) ;
#23902=DIRECTION ( 'NONE',  ( 0.000000000000000000, 1.000000000000000000, 0.000000000000000000 ) ) ;
#23910=EDGE_LOOP ( 'NONE', ( #73509, #26482, #12083 ) ) ;
#23912=CARTESIAN_POINT ( 'NONE',  ( -0.6299212598425060206, 1.724409448818897905, -3.886287458032464226 ) ) ;
#23913=ORIENTED_EDGE ( 'NONE', *, *, #8974, .F. ) ;
#23919=CARTESIAN_POINT ( 'NONE',  ( -0.1959442453386707195, 1.105068466360755064, 3.932155085606260148 ) ) ;
#23936=CARTESIAN_POINT ( 'NONE',  ( -1.947231901457312064, 1.169463170161832100, 0.3010181502270706244 ) ) ;
#23953=CARTESIAN_POINT ( 'NONE',  ( -3.913864544620323294, 1.327201601969144829, 0.4264239150993004990 ) ) ;
#23955=EDGE_CURVE ( 'NONE', #6933, #38768, #48756, .T. ) ;
#23959=B_SPLINE_CURVE_WITH_KNOTS ( 'NONE', 3,
 ( #30011, #54860, #10262, #17820, #35930, #36739, #4344, #17414, #4753, #43453 ),
 .UNSPECIFIED., .F., .F.,
 ( 4, 2, 2, 2, 4 ),
 ( 0.04304707915996866530, 0.04426528421037419919, 0.04548348926077973309, 0.04670169431118526698, 0.04791989936159080088 ),
 .UNSPECIFIED. ) ;
#23961=EDGE_CURVE ( 'NONE', #33187, #27190, #76410, .T. ) ;
#23995=ORIENTED_EDGE ( 'NONE', *, *, #43710, .T. ) ;
#24021=CARTESIAN_POINT ( 'NONE',  ( 0.4359958488159859646, 1.724409448818897905, -3.937007874015760578 ) ) ;
#24027=CARTESIAN_POINT ( 'NONE',  ( -2.593372381816044570, 1.408244132531270454, 0.4567322424080941246 ) ) ;
#24043=CARTESIAN_POINT ( 'NONE',  ( 0.2516608251556240461, 1.134091190147781925, -1.915569722591573987 ) ) ;
#24048=CARTESIAN_POINT ( 'NONE',  ( -0.3771896033470157894, 1.248011834530954323, -3.918935672522287916 ) ) ;
#24062=CARTESIAN_POINT ( 'NONE',  ( 3.900966923095589678, 2.755905511811024056, 0.5314960629921260393 ) ) ;
#24086=CARTESIAN_POINT ( 'NONE',  ( 0.000000000000000000, 0.4374015748031496176, 1.122047244094488194 ) ) ;
#24103=CARTESIAN_POINT ( 'NONE',  ( 3.912791665790199769, 1.724409448818897905, -0.4359958488159719758 ) ) ;
#24106=ORIENTED_EDGE ( 'NONE', *, *, #71135, .F. ) ;
#24107=ORIENTED_EDGE ( 'NONE', *, *, #34103, .F. ) ;
#24111=LINE ( 'NONE', #17821, #47810 ) ;
#24129=CARTESIAN_POINT ( 'NONE',  ( -3.908320185825791881, 1.553306296213791793, -0.4744094488188976277 ) ) ;
#24136=CARTESIAN_POINT ( 'NONE',  ( 0.000000000000000000, 2.755905511811024056, 0.000000000000000000 ) ) ;
#24144=EDGE_CURVE ( 'NONE', #28368, #43450, #74455, .T. ) ;
#24145=CARTESIAN_POINT ( 'NONE',  ( 1.120717929797273582, 1.066111340139089814, 0.06270518838489094748 ) ) ;
#24159=CARTESIAN_POINT ( 'NONE',  ( 0.4744094488188900782, 1.537401574803149984, 2.170146923806596906 ) ) ;
#24176=CYLINDRICAL_SURFACE ( 'NONE', #49293, 0.3149606299212598381 ) ;
#24187=DIRECTION ( 'NONE',  ( 0.000000000000000000, 0.000000000000000000, -1.000000000000000000 ) ) ;
#24203=VERTEX_POINT ( 'NONE', #52680 ) ;
#24206=DIRECTION ( 'NONE',  ( 0.000000000000000000, 0.000000000000000000, -1.000000000000000000 ) ) ;
#24210=CARTESIAN_POINT ( 'NONE',  ( 3.908320185825791881, 1.537401574803149984, 0.4744094488188975722 ) ) ;
#24225=CARTESIAN_POINT ( 'NONE',  ( 2.165487897237717174, 1.580736828574223374, 0.4725026149319441759 ) ) ;
#24254=ORIENTED_EDGE ( 'NONE', *, *, #4102, .F. ) ;
#24267=CARTESIAN_POINT ( 'NONE',  ( 0.3257991949422233136, 1.192497134494935995, -1.407652438512451587 ) ) ;
#24269=EDGE_CURVE ( 'NONE', #4140, #19015, #30447, .T. ) ;
#24271=CIRCLE ( 'NONE', #28313, 1.889763779527559251 ) ;
#24291=VECTOR ( 'NONE', #66118, 39.37007874015748143 ) ;
#24303=CARTESIAN_POINT ( 'NONE',  ( -1.382762875929156809, 1.274900446720740321, 0.3961663554760424533 ) ) ;
#24307=CARTESIAN_POINT ( 'NONE',  ( -0.4744094488188834169, 1.569371252656013516, -3.908320185825794990 ) ) ;
#24313=CARTESIAN_POINT ( 'NONE',  ( 3.915517305244492707, 1.299713873440154099, 0.4108643250733345909 ) ) ;
#24318=VERTEX_POINT ( 'NONE', #13996 ) ;
#24344=CARTESIAN_POINT ( 'NONE',  ( -1.857147851633406788, 1.070284760220074460, 0.08454815954501419817 ) ) ;
#24352=DIRECTION ( 'NONE',  ( 0.000000000000000000, -1.000000000000000000, 0.000000000000000000 ) ) ;
#24363=CARTESIAN_POINT ( 'NONE',  ( -3.920816016192138154, 1.224393450447388343, 0.3568336507794432899 ) ) ;
#24382=ORIENTED_EDGE ( 'NONE', *, *, #57238, .T. ) ;
#24393=AXIS2_PLACEMENT_3D ( 'NONE', #27533, #53190, #16170 ) ;
#24399=ORIENTED_EDGE ( 'NONE', *, *, #13121, .T. ) ;
#24429=CARTESIAN_POINT ( 'NONE',  ( 0.4177787735907000366, 0.3937007874015747699, -1.361336963694947944 ) ) ;
#24436=DIRECTION ( 'NONE',  ( 0.000000000000000000, 0.000000000000000000, -1.000000000000000000 ) ) ;
#24449=CARTESIAN_POINT ( 'NONE',  ( 0.2384209555248066326, 1.126084429615796578, -1.096744324950771121 ) ) ;
#24451=AXIS2_PLACEMENT_3D ( 'NONE', #23650, #3479, #42998 ) ;
#24452=EDGE_CURVE ( 'NONE', #50774, #60402, #57278, .T. ) ;
#24459=CARTESIAN_POINT ( 'NONE',  ( -0.5314960629921172686, 2.755905511811024056, -2.503252890251017604 ) ) ;
#24465=CARTESIAN_POINT ( 'NONE',  ( -0.6299212598425164567, 0.000000000000000000, -0.9285414500055735321 ) ) ;
#24473=DIRECTION ( 'NONE',  ( 0.000000000000000000, -1.000000000000000000, -0.000000000000000000 ) ) ;
#24474=DIRECTION ( 'NONE',  ( 0.000000000000000000, 0.000000000000000000, 1.000000000000000000 ) ) ;
#24482=VERTEX_POINT ( 'NONE', #75692 ) ;
#24499=CARTESIAN_POINT ( 'NONE',  ( -0.2886821576726690264, 1.160628398849495868, -1.939323366023511852 ) ) ;
#24500=VERTEX_POINT ( 'NONE', #63458 ) ;
#24515=VECTOR ( 'NONE', #35049, 39.37007874015748143 ) ;
#24523=DIRECTION ( 'NONE',  ( 0.000000000000000000, 0.000000000000000000, 1.000000000000000000 ) ) ;
#24527=SURFACE_SIDE_STYLE ('',( #37162 ) ) ;
#24541=B_SPLINE_CURVE_WITH_KNOTS ( 'NONE', 3,
 ( #43474, #34616, #14017, #45552 ),
 .UNSPECIFIED., .F., .F.,
 ( 4, 4 ),
 ( 0.09865403381126973403, 0.1000779257405593758 ),
 .UNSPECIFIED. ) ;
#24551=LINE ( 'NONE', #50217, #34409 ) ;
#24559=CARTESIAN_POINT ( 'NONE',  ( 1.111560454228161632, 1.088337758531439992, -0.1537820215174434957 ) ) ;
#24569=CIRCLE ( 'NONE', #59481, 0.1771653543307085410 ) ;
#24587=CARTESIAN_POINT ( 'NONE',  ( -0.3573726498115010752, 1.223876645116869000, 1.063858708914491524 ) ) ;
#24607=VECTOR ( 'NONE', #41860, 39.37007874015748143 ) ;
#24618=EDGE_LOOP ( 'NONE', ( #56304, #27225, #54969, #65436, #21826, #6615, #82996, #11137, #13136, #40688, #74849, #70590, #49901, #37618, #77313, #75271, #61478, #68226, #61135, #74198, #68505, #28558, #1888, #56649, #79951, #17555, #25298, #70152, #66764, #45943, #1465, #38688, #59278, #62179, #60501, #73710 ) ) ;
#24619=DIRECTION ( 'NONE',  ( 0.000000000000000000, -1.000000000000000000, -0.000000000000000000 ) ) ;
#24625=DIRECTION ( 'NONE',  ( -1.000000000000000000, 0.000000000000000000, -3.491481338843132961E-15 ) ) ;
#24627=EDGE_CURVE ( 'NONE', #50308, #61368, #69369, .T. ) ;
#24641=ORIENTED_EDGE ( 'NONE', *, *, #1862, .T. ) ;
#24663=DIRECTION ( 'NONE',  ( -0.000000000000000000, 1.000000000000000000, -0.000000000000000000 ) ) ;
#24679=AXIS2_PLACEMENT_3D ( 'NONE', #43838, #64044, #11889 ) ;
#24695=ORIENTED_EDGE ( 'NONE', *, *, #11333, .T. ) ;
#24719=CARTESIAN_POINT ( 'NONE',  ( 0.000000000000000000, 2.755905511811024056, 0.000000000000000000 ) ) ;
#24722=AXIS2_PLACEMENT_3D ( 'NONE', #1323, #28221, #59790 ) ;
#24726=ORIENTED_EDGE ( 'NONE', *, *, #7531, .T. ) ;
#24729=ORIENTED_EDGE ( 'NONE', *, *, #19143, .T. ) ;
#24752=CARTESIAN_POINT ( 'NONE',  ( 0.4177787735907000366, 0.3937007874015747699, -1.757006255033530806 ) ) ;
#24760=CARTESIAN_POINT ( 'NONE',  ( -3.224202737261815166, 2.716535433070866645, 0.5314960629921260393 ) ) ;
#24770=CARTESIAN_POINT ( 'NONE',  ( -3.927306557984919344, 1.151598356332751871, 0.2765182861327670771 ) ) ;
#24774=DIRECTION ( 'NONE',  ( 0.000000000000000000, 1.000000000000000000, 0.000000000000000000 ) ) ;
#24782=FACE_OUTER_BOUND ( 'NONE', #38069, .T. ) ;
#24790=CIRCLE ( 'NONE', #70458, 0.3149606299212598381 ) ;
#24806=VERTEX_POINT ( 'NONE', #50812 ) ;
#24810=CARTESIAN_POINT ( 'NONE',  ( 2.776658174029195347, 1.170105060311650069, -0.3006284332565901662 ) ) ;
#24840=ADVANCED_FACE ( 'NONE', ( #81185 ), #18444, .F. ) ;
#24842=CARTESIAN_POINT ( 'NONE',  ( -2.558820304884324326, 1.494558157769224183, 0.4725443725032419939 ) ) ;
#24855=CARTESIAN_POINT ( 'NONE',  ( 0.1539095575340513611, 1.088378732996000631, -1.111543816720518274 ) ) ;
#24865=DIRECTION ( 'NONE',  ( 1.000000000000000000, -0.000000000000000000, -0.000000000000000000 ) ) ;
#24882=FACE_OUTER_BOUND ( 'NONE', #74316, .T. ) ;
#24891=LINE ( 'NONE', #76263, #30546 ) ;
#24906=ORIENTED_EDGE ( 'NONE', *, *, #82137, .T. ) ;
#24907=AXIS2_PLACEMENT_3D ( 'NONE', #46820, #33379, #72511 ) ;
#24920=EDGE_CURVE ( 'NONE', #48388, #49969, #74487, .T. ) ;
#24923=ORIENTED_EDGE ( 'NONE', *, *, #80068, .F. ) ;
#24924=ORIENTED_EDGE ( 'NONE', *, *, #37615, .T. ) ;
#24943=CARTESIAN_POINT ( 'NONE',  ( -6.686372609646914991E-25, 1.062992125984252745, 1.850393700787401619 ) ) ;
#24949=FACE_OUTER_BOUND ( 'NONE', #31355, .T. ) ;
#24957=EDGE_CURVE ( 'NONE', #43450, #49642, #70762, .T. ) ;
#24958=CARTESIAN_POINT ( 'NONE',  ( 1.024231438423351292, 1.413526771164698159, 0.4582195470708000373 ) ) ;
#24961=CONICAL_SURFACE ( 'NONE', #69328, 1.968503937007874072, 0.7853981633974500554 ) ;
#24992=EDGE_CURVE ( 'NONE', #3121, #76416, #31762, .T. ) ;
#25000=AXIS2_PLACEMENT_3D ( 'NONE', #6112, #31784, #57447 ) ;
#25003=CONICAL_SURFACE ( 'NONE', #59992, 2.165354330708661568, 0.7853981633974500554 ) ;
#25028=DIRECTION ( 'NONE',  ( 0.000000000000000000, 0.000000000000000000, -1.000000000000000000 ) ) ;
#25029=CARTESIAN_POINT ( 'NONE',  ( 0.1406185367545949583, 0.000000000000000000, -1.409564117849439802 ) ) ;
#25037=DIRECTION ( 'NONE',  ( -1.000000000000000000, -0.000000000000000000, -0.000000000000000000 ) ) ;
#25072=ORIENTED_EDGE ( 'NONE', *, *, #36983, .T. ) ;
#25081=CARTESIAN_POINT ( 'NONE',  ( 1.348312163386739426, 0.2755905511811023723, 0.7386866130305692613 ) ) ;
#25087=CARTESIAN_POINT ( 'NONE',  ( 0.3165050273377052470, 1.183948952745706995, -1.413700202057344590 ) ) ;
#25111=VECTOR ( 'NONE', #69728, 39.37007874015748143 ) ;
#25118=AXIS2_PLACEMENT_3D ( 'NONE', #82198, #77113, #36732 ) ;
#25119=AXIS2_PLACEMENT_3D ( 'NONE', #43660, #50396, #76093 ) ;
#25136=VERTEX_POINT ( 'NONE', #70597 ) ;
#25144=DIRECTION ( 'NONE',  ( -1.000000000000000000, 0.000000000000000000, -3.491481338843132961E-15 ) ) ;
#25177=EDGE_CURVE ( 'NONE', #42693, #5361, #21102, .T. ) ;
#25184=CARTESIAN_POINT ( 'NONE',  ( -3.918068336532610108, 1.260885577041682248, 0.3858078592113795557 ) ) ;
#25189=EDGE_CURVE ( 'NONE', #67810, #68995, #43816, .T. ) ;
#25191=EDGE_LOOP ( 'NONE', ( #1736, #80838, #9421, #81480 ) ) ;
#25204=ORIENTED_EDGE ( 'NONE', *, *, #67559, .T. ) ;
#25216=CARTESIAN_POINT ( 'NONE',  ( 0.4567483893478956336, 1.408297760469685356, -2.593341242975145899 ) ) ;
#25219=VERTEX_POINT ( 'NONE', #33137 ) ;
#25221=ORIENTED_EDGE ( 'NONE', *, *, #56394, .F. ) ;
#25224=B_SPLINE_CURVE_WITH_KNOTS ( 'NONE', 3,
 ( #4299, #41367, #75022, #16119 ),
 .UNSPECIFIED., .F., .F.,
 ( 4, 4 ),
 ( 9.989667305668851654E-07, 0.001428340232518097606 ),
 .UNSPECIFIED. ) ;
#25250=EDGE_CURVE ( 'NONE', #13252, #28229, #1166, .T. ) ;
#25253=CARTESIAN_POINT ( 'NONE',  ( -2.556694656352302530, 1.572145545125843924, -0.4734416007054419451 ) ) ;
#25256=DIRECTION ( 'NONE',  ( -0.000000000000000000, -1.000000000000000000, -0.000000000000000000 ) ) ;
#25268=CARTESIAN_POINT ( 'NONE',  ( 0.2112933010598323225, 1.111520798820692990, -1.102352278213539316 ) ) ;
#25271=CARTESIAN_POINT ( 'NONE',  ( 0.3006999498584591590, 1.170162153792016158, -1.947802021145076168 ) ) ;
#25276=CARTESIAN_POINT ( 'NONE',  ( 1.854472803289052507, 2.716535433070866645, -0.5314960629921260393 ) ) ;
#25281=DIRECTION ( 'NONE',  ( 0.000000000000000000, -1.000000000000000000, -0.000000000000000000 ) ) ;
#25290=DIRECTION ( 'NONE',  ( 0.000000000000000000, -0.000000000000000000, -1.000000000000000000 ) ) ;
#25294=CARTESIAN_POINT ( 'NONE',  ( 0.4177787735907000366, 1.299212598425196985, -1.559171609364239375 ) ) ;
#25298=ORIENTED_EDGE ( 'NONE', *, *, #47465, .T. ) ;
#25304=CARTESIAN_POINT ( 'NONE',  ( -3.924389226575468737, 2.165354330708661568, 0.3149606299212595606 ) ) ;
#25308=EDGE_CURVE ( 'NONE', #10444, #58992, #65231, .T. ) ;
#25315=DIRECTION ( 'NONE',  ( 0.000000000000000000, 9.738798461624180871E-16, 1.000000000000000000 ) ) ;
#25330=CARTESIAN_POINT ( 'NONE',  ( 1.912049360642951330E-20, 1.062992125984252745, -2.874015748031495843 ) ) ;
#25332=DIRECTION ( 'NONE',  ( 0.000000000000000000, -1.000000000000000000, 1.408710688920637755E-15 ) ) ;
#25337=EDGE_CURVE ( 'NONE', #38567, #13837, #2819, .T. ) ;
#25338=ORIENTED_EDGE ( 'NONE', *, *, #66088, .T. ) ;
#25363=CARTESIAN_POINT ( 'NONE',  ( -0.4425803288943545577, 1.365943002350755053, 2.104928023556738914 ) ) ;
#25368=DIRECTION ( 'NONE',  ( 1.000000000000000000, -0.000000000000000000, -0.000000000000000000 ) ) ;
#25439=DIRECTION ( 'NONE',  ( 0.000000000000000000, 0.000000000000000000, -1.000000000000000000 ) ) ;
#25459=EDGE_CURVE ( 'NONE', #26586, #48126, #61326, .T. ) ;
#25484=ORIENTED_EDGE ( 'NONE', *, *, #46415, .F. ) ;
#25500=CARTESIAN_POINT ( 'NONE',  ( -0.03443470937339728616, 0.2755905511811023723, -1.753551325310622078 ) ) ;
#25507=EDGE_CURVE ( 'NONE', #51592, #10444, #984, .T. ) ;
#25513=ORIENTED_EDGE ( 'NONE', *, *, #32216, .T. ) ;
#25520=DIRECTION ( 'NONE',  ( 0.000000000000000000, 1.000000000000000000, -0.000000000000000000 ) ) ;
#25528=ORIENTED_EDGE ( 'NONE', *, *, #36242, .F. ) ;
#25546=EDGE_LOOP ( 'NONE', ( #13866, #7639, #69444, #70525 ) ) ;
#25547=VERTEX_POINT ( 'NONE', #82317 ) ;
#25554=CARTESIAN_POINT ( 'NONE',  ( 1.947751274789685016, 1.170105060311642742, 0.3006284332565817285 ) ) ;
#25595=CARTESIAN_POINT ( 'NONE',  ( -3.915444394612497714, 1.299891025107167364, 0.4118628028680341169 ) ) ;
#25615=ORIENTED_EDGE ( 'NONE', *, *, #78000, .T. ) ;
#25636=DIRECTION ( 'NONE',  ( 1.000000000000000000, -0.000000000000000000, 3.491481338843132961E-15 ) ) ;
#25647=CIRCLE ( 'NONE', #80846, 3.937007874015748143 ) ;
#25667=AXIS2_PLACEMENT_3D ( 'NONE', #44135, #37427, #43304 ) ;
#25671=CARTESIAN_POINT ( 'NONE',  ( 1.076935383196057749, -5.463695987328518425E-17, -0.3149606299212591720 ) ) ;
#25693=CARTESIAN_POINT ( 'NONE',  ( -0.1959128669332750872, 1.105054483805734566, -3.932156628022151157 ) ) ;
#25698=CARTESIAN_POINT ( 'NONE',  ( 1.868118594278514344, 2.729653106663536555, 0.5314960629921260393 ) ) ;
#25731=CARTESIAN_POINT ( 'NONE',  ( 0.000000000000000000, 2.755905511811024056, 0.000000000000000000 ) ) ;
#25736=ORIENTED_EDGE ( 'NONE', *, *, #15160, .T. ) ;
#25748=FACE_OUTER_BOUND ( 'NONE', #76795, .T. ) ;
#25751=ORIENTED_EDGE ( 'NONE', *, *, #18704, .F. ) ;
#25763=PRODUCT ( 'Cast Iron Heavy Chuck Body', 'Cast Iron Heavy Chuck Body', '', ( #68350 ) ) ;
#25779=CARTESIAN_POINT ( 'NONE',  ( -0.08477834984147802899, 1.070319560067209963, 1.857180095838086631 ) ) ;
#25793=CARTESIAN_POINT ( 'NONE',  ( 1.077480042006655703, 1.180860146545615885, 0.3133340167985102509 ) ) ;
#25805=CARTESIAN_POINT ( 'NONE',  ( 0.6299212598424784870, 2.165354330708661568, 3.937007874015796105 ) ) ;
#25809=EDGE_CURVE ( 'NONE', #64186, #2910, #11601, .T. ) ;
#25821=CARTESIAN_POINT ( 'NONE',  ( 0.4177787735907000366, 0.3937007874015748254, -1.559171609364239375 ) ) ;
#25857=CLOSED_SHELL ( 'NONE', ( #74348, #75100, #71156, #69191, #33473, #11941, #82590, #12134, #60173, #18684, #61504, #22635, #70074, #62024, #63467, #8043, #55189, #36506, #35461, #41549, #27491, #80719, #47069, #11624, #28941, #30648, #77956, #13717, #12143, #51550, #5872, #46293, #8117, #71640, #19724, #40121, #36166, #65122, #45547, #30331, #68450, #34686, #38163, #75824, #14043, #71282, #995, #31168, #47984, #48514, #38323, #10452, #62411, #30668, #31175, #21981, #29986, #67090, #18794, #61336, #28474, #44546, #44736, #53424, #8523, #26537, #77668, #28093, #74389, #72528, #64894, #75484, #4827, #65316, #63425, #52596, #4176, #33389, #40464, #36257, #60304, #73876, #39944, #36194, #72439, #29137, #4673, #5428, #12182, #64484, #67221, #74186, #76043, #72658, #53265, #19748, #59438, #26870, #49957, #44444, #26046, #49179, #23889, #55290, #16951, #5061, #56282, #27094, #70686, #55749, #11406, #23337, #76267, #13813, #37367, #74057, #42342, #29106, #80571, #20648, #54159, #9057, #10898, #9532, #11732, #8303, #21883, #13194, #29568, #7468, #51124, #22913, #33047, #79109, #9822, #73241, #78873, #28938, #50679, #47621, #68661, #12761, #73395, #9472, #56234, #1837, #58771, #49657, #16811, #74795, #60552, #32317, #59116, #28336, #7861, #24840, #56841, #13237, #55020, #18148, #34742, #4371, #15112, #7893, #69392, #58291, #53257, #64340, #1705, #72691, #35600, #59970, #71759, #64110, #79061, #2735, #1770, #52837, #54723, #790, #57483, #74831, #64625, #34263, #56077, #64633, #18709, #10373, #40934, #8356, #39351, #59497, #47329, #28632, #15084, #8910, #19785, #75418, #43999, #65582, #9254, #4804 ) ) ;
#25858=CARTESIAN_POINT ( 'NONE',  ( -0.4124503923812501971, 1.301275207309029014, 2.666248201964647180 ) ) ;
#25868=CARTESIAN_POINT ( 'NONE',  ( 0.4153789062890288486, 1.308162955913704462, -1.721441067367122990 ) ) ;
#25874=CARTESIAN_POINT ( 'NONE',  ( 1.033875059083676717, 1.724409448818897905, 0.4359958488159722534 ) ) ;
#25879=CIRCLE ( 'NONE', #48784, 1.178877988035069047 ) ;
#25905=EDGE_CURVE ( 'NONE', #66126, #45287, #62720, .T. ) ;
#25919=PRODUCT_DEFINITION ( 'UNKNOWN', '', #49063, #7487 ) ;
#25920=AXIS2_PLACEMENT_3D ( 'NONE', #38536, #6132, #64217 ) ;
#25921=CARTESIAN_POINT ( 'NONE',  ( 0.3256317079376986889, 1.192144240734427818, -1.710856511100560029 ) ) ;
#25941=EDGE_CURVE ( 'NONE', #35211, #33346, #43570, .T. ) ;
#25960=CARTESIAN_POINT ( 'NONE',  ( 2.094141031014985721, 1.724409448818900570, -0.4359958488159719758 ) ) ;
#25967=ORIENTED_EDGE ( 'NONE', *, *, #80626, .T. ) ;
#25974=EDGE_CURVE ( 'NONE', #27710, #74865, #26353, .T. ) ;
#25975=CARTESIAN_POINT ( 'NONE',  ( 2.114058874202384253, 1.379859446982308446, 0.4477348144951676656 ) ) ;
#25977=DIRECTION ( 'NONE',  ( 1.000000000000000000, 0.000000000000000000, 3.455050906509825972E-15 ) ) ;
#25988=CARTESIAN_POINT ( 'NONE',  ( -0.03443470937343537375, 1.064243487142137568, -1.440673310089392478 ) ) ;
#25989=AXIS2_PLACEMENT_3D ( 'NONE', #52506, #45774, #772 ) ;
#26003=AXIS2_PLACEMENT_3D ( 'NONE', #21610, #59078, #46855 ) ;
#26023=ORIENTED_EDGE ( 'NONE', *, *, #28811, .T. ) ;
#26029=DIRECTION ( 'NONE',  ( -0.000000000000000000, 1.000000000000000000, -0.000000000000000000 ) ) ;
#26039=ORIENTED_EDGE ( 'NONE', *, *, #61973, .T. ) ;
#26046=ADVANCED_FACE ( 'NONE', ( #44384 ), #82720, .T. ) ;
#26059=FACE_OUTER_BOUND ( 'NONE', #77693, .T. ) ;
#26071=CARTESIAN_POINT ( 'NONE',  ( -2.594411373832338441, 1.668416680336019198, 0.4562095852119718575 ) ) ;
#26091=LINE ( 'NONE', #39562, #38585 ) ;
#26119=TOROIDAL_SURFACE ( 'NONE', #7326, 3.858267716535433323, 0.07874015748031495954 ) ;
#26135=EDGE_CURVE ( 'NONE', #72153, #49485, #32193, .T. ) ;
#26202=CARTESIAN_POINT ( 'NONE',  ( -0.1345703391920888281, 1.081211091791626222, 1.867241868865190391 ) ) ;
#26230=EDGE_CURVE ( 'NONE', #56386, #17817, #51951, .T. ) ;
#26273=VERTEX_POINT ( 'NONE', #19988 ) ;
#26278=CARTESIAN_POINT ( 'NONE',  ( 1.076935383196057749, 2.559055118110236560, -0.3149606299212596716 ) ) ;
#26279=CARTESIAN_POINT ( 'NONE',  ( -0.04294987210466714306, 1.064862614867412516, 2.872282311130982979 ) ) ;
#26280=CARTESIAN_POINT ( 'NONE',  ( 0.4177787735907000366, 0.2755905511811023723, -1.559171609364239375 ) ) ;
#26287=ORIENTED_EDGE ( 'NONE', *, *, #61531, .F. ) ;
#26288=LINE ( 'NONE', #65019, #29917 ) ;
#26290=CARTESIAN_POINT ( 'NONE',  ( 0.5314960629921396951, 2.755905511811024056, -3.937007874015760578 ) ) ;
#26291=CARTESIAN_POINT ( 'NONE',  ( -0.5314960629921193780, 2.755905511811024056, -1.895394334970793793 ) ) ;
#26296=AXIS2_PLACEMENT_3D ( 'NONE', #18633, #82610, #71229 ) ;
#26298=CARTESIAN_POINT ( 'NONE',  ( -1.895394334970792016, 2.755905511811024056, -0.5314960629921260393 ) ) ;
#26299=CARTESIAN_POINT ( 'NONE',  ( 2.583694225513480713, 2.755905511811024056, -0.5314960629921260393 ) ) ;
#26322=DIRECTION ( 'NONE',  ( 0.000000000000000000, 1.000000000000000000, 0.000000000000000000 ) ) ;
#26326=ORIENTED_EDGE ( 'NONE', *, *, #21327, .T. ) ;
#26333=VECTOR ( 'NONE', #35612, 39.37007874015748143 ) ;
#26341=CARTESIAN_POINT ( 'NONE',  ( 1.019880138406203063, 1.617842475621884768, 0.4678109194727893549 ) ) ;
#26352=CARTESIAN_POINT ( 'NONE',  ( 0.000000000000000000, 1.724409448818897905, 0.000000000000000000 ) ) ;
#26353=CIRCLE ( 'NONE', #35814, 1.244489337948954555 ) ;
#26361=LINE ( 'NONE', #39410, #78666 ) ;
#26365=EDGE_CURVE ( 'NONE', #10035, #36478, #14105, .T. ) ;
#26367=EDGE_CURVE ( 'NONE', #55060, #80751, #6026, .T. ) ;
#26371=ORIENTED_EDGE ( 'NONE', *, *, #23961, .F. ) ;
#26381=B_SPLINE_CURVE_WITH_KNOTS ( 'NONE', 3,
 ( #68716, #43429, #69126, #82583, #11476, #18609, #37132, #30814, #56479, #82182, #44252, #24499, #50165, #75861, #18203, #6800, #7223, #21107, #13135, #32471, #58133, #32056, #502, #70784, #51393, #66144, #64463, #8072, #45080, #77521 ),
 .UNSPECIFIED., .F., .F.,
 ( 4, 2, 2, 2, 2, 2, 2, 2, 2, 2, 2, 2, 2, 2, 4 ),
 ( 0.02630788966047508878, 0.02761938857346193238, 0.02893088748644877597, 0.03024238639943561957, 0.03155388531242245970, 0.03417688313839615383, 0.03548838205138300089, 0.03679988096436985490, 0.03942287879034354903, 0.04073437770333040303, 0.04204587661631725704, 0.04335737552930411798, 0.04466887444229096504, 0.04598037335527782599, 0.04729187226826467999 ),
 .UNSPECIFIED. ) ;
#26385=CARTESIAN_POINT ( 'NONE',  ( 0.4695140184743307188, 1.605872332714558537, 2.158445410120229724 ) ) ;
#26398=DIRECTION ( 'NONE',  ( 0.000000000000000000, -1.000000000000000000, 0.000000000000000000 ) ) ;
#26405=CONICAL_SURFACE ( 'NONE', #4897, 3.307086614173228689, 0.7853981633974500554 ) ;
#26423=VECTOR ( 'NONE', #76100, 39.37007874015748143 ) ;
#26447=CARTESIAN_POINT ( 'NONE',  ( 1.141392835773559211, 0.3937007874015747699, 1.339227481442854195 ) ) ;
#26453=VECTOR ( 'NONE', #34849, 39.37007874015748143 ) ;
#26460=CARTESIAN_POINT ( 'NONE',  ( 0.2098426342062970074, 1.111641651325031566, -3.931435521548293455 ) ) ;
#26461=AXIS2_PLACEMENT_3D ( 'NONE', #40171, #65855, #743 ) ;
#26466=EDGE_LOOP ( 'NONE', ( #68302, #69147, #32254, #76845 ) ) ;
#26468=ORIENTED_EDGE ( 'NONE', *, *, #48374, .F. ) ;
#26482=ORIENTED_EDGE ( 'NONE', *, *, #41448, .T. ) ;
#26515=CARTESIAN_POINT ( 'NONE',  ( -2.571961977011561817, 1.622068519643037554, -0.4668652553835666574 ) ) ;
#26524=CIRCLE ( 'NONE', #76220, 0.1190944881889763746 ) ;
#26535=CYLINDRICAL_SURFACE ( 'NONE', #1803, 3.937007874015748143 ) ;
#26537=ADVANCED_FACE ( 'NONE', ( #58270 ), #34492, .T. ) ;
#26545=DIRECTION ( 'NONE',  ( 0.000000000000000000, 0.000000000000000000, -1.000000000000000000 ) ) ;
#26552=VERTEX_POINT ( 'NONE', #73840 ) ;
#26558=LINE ( 'NONE', #40438, #49830 ) ;
#26567=ORIENTED_EDGE ( 'NONE', *, *, #47141, .T. ) ;
#26571=ORIENTED_EDGE ( 'NONE', *, *, #5433, .F. ) ;
#26586=VERTEX_POINT ( 'NONE', #2299 ) ;
#26590=CONICAL_SURFACE ( 'NONE', #21239, 2.559055118110236560, 0.7853981633974500554 ) ;
#26603=CARTESIAN_POINT ( 'NONE',  ( -0.5314960629921394730, 2.745602313593968891, 3.861135848600277143 ) ) ;
#26630=FACE_OUTER_BOUND ( 'NONE', #19296, .T. ) ;
#26633=EDGE_CURVE ( 'NONE', #79730, #68390, #66694, .T. ) ;
#26644=FACE_OUTER_BOUND ( 'NONE', #53183, .T. ) ;
#26650=DIRECTION ( 'NONE',  ( 1.000000000000000000, 1.408710688920637755E-15, 0.000000000000000000 ) ) ;
#26658=DIRECTION ( 'NONE',  ( 0.000000000000000000, 0.000000000000000000, -1.000000000000000000 ) ) ;
#26677=CARTESIAN_POINT ( 'NONE',  ( 0.1687987930166117423, 1.093765707632013306, 1.109372847106409932 ) ) ;
#26695=ORIENTED_EDGE ( 'NONE', *, *, #33639, .F. ) ;
#26697=ORIENTED_EDGE ( 'NONE', *, *, #29666, .F. ) ;
#26702=PLANE ( 'NONE',  #41705 ) ;
#26706=CARTESIAN_POINT ( 'NONE',  ( 0.4359958488159859091, 1.724409448818897905, -3.912791665790197992 ) ) ;
#26713=DIRECTION ( 'NONE',  ( 0.000000000000000000, 1.000000000000000000, -0.000000000000000000 ) ) ;
#26715=EDGE_CURVE ( 'NONE', #51415, #32057, #79746, .T. ) ;
#26718=VERTEX_POINT ( 'NONE', #46474 ) ;
#26719=DIRECTION ( 'NONE',  ( -0.000000000000000000, -1.000000000000000000, -0.000000000000000000 ) ) ;
#26720=DIRECTION ( 'NONE',  ( 0.000000000000000000, 0.000000000000000000, -1.000000000000000000 ) ) ;
#26746=DIRECTION ( 'NONE',  ( -0.000000000000000000, -1.000000000000000000, -0.000000000000000000 ) ) ;
#26774=ORIENTED_EDGE ( 'NONE', *, *, #38804, .T. ) ;
#26809=EDGE_LOOP ( 'NONE', ( #22245, #33131, #76679, #65319, #63125, #61784 ) ) ;
#26810=ORIENTED_EDGE ( 'NONE', *, *, #56687, .T. ) ;
#26817=CARTESIAN_POINT ( 'NONE',  ( -0.4744094488189106174, 1.537401574803149984, 3.908320185825790105 ) ) ;
#26841=CARTESIAN_POINT ( 'NONE',  ( -1.016821367227983552, 1.537401574803149984, -0.4744094488188975722 ) ) ;
#26845=CARTESIAN_POINT ( 'NONE',  ( 0.3149606299212737159, 2.165354330708661568, -3.937007874015761022 ) ) ;
#26863=ORIENTED_EDGE ( 'NONE', *, *, #53218, .T. ) ;
#26864=CARTESIAN_POINT ( 'NONE',  ( 0.000000000000000000, 0.000000000000000000, 0.000000000000000000 ) ) ;
#26869=DIRECTION ( 'NONE',  ( 0.000000000000000000, 1.000000000000000000, 0.000000000000000000 ) ) ;
#26870=ADVANCED_FACE ( 'NONE', ( #34702 ), #80165, .T. ) ;
#26873=CARTESIAN_POINT ( 'NONE',  ( 0.4713254705329260053, 1.475163719089159997, -3.908698025846080171 ) ) ;
#26892=ORIENTED_EDGE ( 'NONE', *, *, #56817, .T. ) ;
#26897=CARTESIAN_POINT ( 'NONE',  ( 2.723802780027873016, 1.230840736494986709, 0.3632157284009329135 ) ) ;
#26904=CARTESIAN_POINT ( 'NONE',  ( 1.348312163386739426, 0.2755905511811023723, 0.7386866130305692613 ) ) ;
#26909=CARTESIAN_POINT ( 'NONE',  ( -0.3149606299212558413, 2.165354330708661568, -1.076935383196058860 ) ) ;
#26941=B_SPLINE_CURVE_WITH_KNOTS ( 'NONE', 3,
 ( #83022, #7683, #19039, #78390 ),
 .UNSPECIFIED., .F., .F.,
 ( 4, 4 ),
 ( 2.857347768990396770E-07, 0.001436604392377179105 ),
 .UNSPECIFIED. ) ;
#26967=CARTESIAN_POINT ( 'NONE',  ( 0.4603218807116906675, 1.653261878685373665, -2.138334326189375023 ) ) ;
#26972=CARTESIAN_POINT ( 'NONE',  ( 3.937007874015748143, 2.165354330708661568, 0.3149606299212600047 ) ) ;
#26979=VERTEX_POINT ( 'NONE', #15126 ) ;
#26983=CARTESIAN_POINT ( 'NONE',  ( 1.348312163386739426, 0.2755905511811023723, 0.7386866130305692613 ) ) ;
#26992=CARTESIAN_POINT ( 'NONE',  ( 0.000000000000000000, 2.755905511811024056, 0.000000000000000000 ) ) ;
#26998=ORIENTED_EDGE ( 'NONE', *, *, #62552, .T. ) ;
#27014=CARTESIAN_POINT ( 'NONE',  ( 3.916325068365210438, 1.286797242935906471, -0.4031187015191872725 ) ) ;
#27015=ORIENTED_EDGE ( 'NONE', *, *, #13664, .F. ) ;
#27041=DIRECTION ( 'NONE',  ( -0.000000000000000000, -1.000000000000000000, -0.000000000000000000 ) ) ;
#27052=EDGE_CURVE ( 'NONE', #37547, #23879, #46255, .T. ) ;
#27053=CARTESIAN_POINT ( 'NONE',  ( 1.074005671585215538, 1.191469999471042041, -0.3250085130549520973 ) ) ;
#27062=DIRECTION ( 'NONE',  ( -1.000000000000000000, -0.000000000000000000, -0.000000000000000000 ) ) ;
#27067=CIRCLE ( 'NONE', #17652, 1.122047244094488194 ) ;
#27089=CARTESIAN_POINT ( 'NONE',  ( 0.2118050467152636229, 1.111762164670342390, 1.102258206560161158 ) ) ;
#27094=ADVANCED_FACE ( 'NONE', ( #72369 ), #14303, .F. ) ;
#27108=ORIENTED_EDGE ( 'NONE', *, *, #39374, .T. ) ;
#27113=DIRECTION ( 'NONE',  ( 0.000000000000000000, 0.000000000000000000, 1.000000000000000000 ) ) ;
#27114=CARTESIAN_POINT ( 'NONE',  ( -0.2240801135442098413, 1.118954560528812037, 2.822610029984497171 ) ) ;
#27121=ORIENTED_EDGE ( 'NONE', *, *, #48672, .T. ) ;
#27130=ORIENTED_EDGE ( 'NONE', *, *, #71612, .F. ) ;
#27132=CARTESIAN_POINT ( 'NONE',  ( -3.937007874015748143, 1.537401574803149984, -2.901595197523589142E-16 ) ) ;
#27156=CARTESIAN_POINT ( 'NONE',  ( 0.5314960629920859603, 2.755905511811024056, 3.821484228344198986 ) ) ;
#27163=ORIENTED_EDGE ( 'NONE', *, *, #14047, .F. ) ;
#27187=CARTESIAN_POINT ( 'NONE',  ( -2.503252890251015828, 2.755905511811024056, 0.5314960629921260393 ) ) ;
#27189=EDGE_CURVE ( 'NONE', #66338, #79813, #34477, .T. ) ;
#27190=VERTEX_POINT ( 'NONE', #28569 ) ;
#27207=VERTEX_POINT ( 'NONE', #41202 ) ;
#27219=CARTESIAN_POINT ( 'NONE',  ( 0.4359958488159500489, 1.724409448818897905, 2.094141031014936871 ) ) ;
#27225=ORIENTED_EDGE ( 'NONE', *, *, #24920, .T. ) ;
#27228=AXIS2_PLACEMENT_3D ( 'NONE', #64858, #58107, #72015 ) ;
#27231=( LENGTH_UNIT ( ) NAMED_UNIT ( * ) SI_UNIT ( $, .METRE. ) );
#27233=CARTESIAN_POINT ( 'NONE',  ( 2.139011644334231743, 1.422882880004778139, 0.4606469518571244537 ) ) ;
#27263=CARTESIAN_POINT ( 'NONE',  ( 0.4744094488188886904, 1.537401574803149984, 2.554262525012303886 ) ) ;
#27272=CARTESIAN_POINT ( 'NONE',  ( -3.916339746322849980, 1.286570825603250201, -0.4029754474414414256 ) ) ;
#27277=AXIS2_PLACEMENT_3D ( 'NONE', #59361, #2964, #65708 ) ;
#27285=EDGE_CURVE ( 'NONE', #56091, #8593, #75370, .T. ) ;
#27289=CARTESIAN_POINT ( 'NONE',  ( 0.3462931014723631407, 1.212771528347503347, -3.921763973690792326 ) ) ;
#27308=ORIENTED_EDGE ( 'NONE', *, *, #4102, .T. ) ;
#27310=VERTEX_POINT ( 'NONE', #35710 ) ;
#27313=CARTESIAN_POINT ( 'NONE',  ( -1.504247987312398616, 1.133706091002348426, 0.2492029244898440743 ) ) ;
#27325=CARTESIAN_POINT ( 'NONE',  ( -2.630268417803885317, 1.724409448818897905, 0.4359958488159718093 ) ) ;
#27340=CIRCLE ( 'NONE', #19273, 0.1978346456692914035 ) ;
#27347=DIRECTION ( 'NONE',  ( 0.000000000000000000, -0.6427876096865352551, -0.7660444431189814551 ) ) ;
#27360=DIRECTION ( 'NONE',  ( 8.881784197001252323E-16, 0.000000000000000000, 1.000000000000000000 ) ) ;
#27377=VERTEX_POINT ( 'NONE', #28978 ) ;
#27384=CARTESIAN_POINT ( 'NONE',  ( 0.4470293165555208059, 1.696956328257586577, -2.112781292380983444 ) ) ;
#27396=ORIENTED_EDGE ( 'NONE', *, *, #64058, .F. ) ;
#27411=ORIENTED_EDGE ( 'NONE', *, *, #8016, .T. ) ;
#27424=CARTESIAN_POINT ( 'NONE',  ( 2.543486866223389153, 2.716535433070866645, -0.5314960629921260393 ) ) ;
#27430=CARTESIAN_POINT ( 'NONE',  ( 3.908688349857626587, 1.475633291777086020, -0.4714062836140362478 ) ) ;
#27431=EDGE_CURVE ( 'NONE', #60812, #21419, #24271, .T. ) ;
#27454=EDGE_CURVE ( 'NONE', #53272, #8593, #3729, .T. ) ;
#27456=EDGE_CURVE ( 'NONE', #42276, #49776, #10047, .T. ) ;
#27461=AXIS2_PLACEMENT_3D ( 'NONE', #23555, #29868, #5845 ) ;
#27463=CARTESIAN_POINT ( 'NONE',  ( -0.4602852883866647149, 1.653403552777526819, 2.138259192565361566 ) ) ;
#27469=DIRECTION ( 'NONE',  ( 0.000000000000000000, 0.000000000000000000, -1.000000000000000000 ) ) ;
#27491=ADVANCED_FACE ( 'NONE', ( #10869 ), #47112, .F. ) ;
#27497=CARTESIAN_POINT ( 'NONE',  ( 0.4177787735906991484, 1.312623414240987163, -1.404325600637324367 ) ) ;
#27507=CARTESIAN_POINT ( 'NONE',  ( 0.2899149735282853246, 1.161568142327694897, 1.084016376660781100 ) ) ;
#27512=VECTOR ( 'NONE', #76566, 39.37007874015748143 ) ;
#27533=CARTESIAN_POINT ( 'NONE',  ( 0.000000000000000000, 2.755905511811024056, 0.000000000000000000 ) ) ;
#27536=DIRECTION ( 'NONE',  ( -0.000000000000000000, -1.000000000000000000, -0.000000000000000000 ) ) ;
#27539=ORIENTED_EDGE ( 'NONE', *, *, #22805, .F. ) ;
#27541=CARTESIAN_POINT ( 'NONE',  ( -1.018274559621366038, 1.474925757642550295, -0.4713314535542892925 ) ) ;
#27550=DIRECTION ( 'NONE',  ( 0.000000000000000000, -0.000000000000000000, -1.000000000000000000 ) ) ;
#27566=CARTESIAN_POINT ( 'NONE',  ( -0.6299212598425332210, 1.724409448818897905, 3.886287458032460229 ) ) ;
#27573=CIRCLE ( 'NONE', #2046, 1.122047244094488194 ) ;
#27578=DIRECTION ( 'NONE',  ( -0.000000000000000000, -1.000000000000000000, -0.000000000000000000 ) ) ;
#27582=DIRECTION ( 'NONE',  ( 0.000000000000000000, 0.000000000000000000, -1.000000000000000000 ) ) ;
#27584=VERTEX_POINT ( 'NONE', #38178 ) ;
#27599=CARTESIAN_POINT ( 'NONE',  ( 0.4177787735907000366, 0.3937007874015748254, -1.874132239285499324 ) ) ;
#27627=DIRECTION ( 'NONE',  ( 0.000000000000000000, 1.000000000000000000, -0.000000000000000000 ) ) ;
#27628=CIRCLE ( 'NONE', #65258, 0.2165354330708660069 ) ;
#27650=CARTESIAN_POINT ( 'NONE',  ( 2.131054703900698843, 1.408268389154267552, -0.4567427728026668410 ) ) ;
#27657=CARTESIAN_POINT ( 'NONE',  ( -0.4744094488189058989, 1.537401574803149984, 2.554262525012261253 ) ) ;
#27672=VECTOR ( 'NONE', #36768, 39.37007874015748143 ) ;
#27674=CARTESIAN_POINT ( 'NONE',  ( 0.4410019072768808779, 1.362365694854143383, -1.490705430580310464 ) ) ;
#27675=EDGE_CURVE ( 'NONE', #46125, #80970, #75677, .T. ) ;
#27683=CARTESIAN_POINT ( 'NONE',  ( -0.5314960629921123836, 2.559055118110236560, -3.900966923095591454 ) ) ;
#27690=AXIS2_PLACEMENT_3D ( 'NONE', #36334, #4754, #48957 ) ;
#27693=CARTESIAN_POINT ( 'NONE',  ( -0.6299212598425332210, 2.755905511811024056, 3.886287458032460229 ) ) ;
#27699=CARTESIAN_POINT ( 'NONE',  ( -3.898836503597932435, 2.697992270790282365, -0.5314960629921259283 ) ) ;
#27707=CARTESIAN_POINT ( 'NONE',  ( -2.530077749183804237, 2.729661042043246777, -0.5314960629921260393 ) ) ;
#27710=VERTEX_POINT ( 'NONE', #12517 ) ;
#27731=AXIS2_PLACEMENT_3D ( 'NONE', #3126, #3955, #41011 ) ;
#27746=CARTESIAN_POINT ( 'NONE',  ( -2.611754389584905578, 1.697151583350148041, 0.4469586986359056491 ) ) ;
#27773=CARTESIAN_POINT ( 'NONE',  ( -2.001206130748376832, 1.231544801320217264, -0.3638227417423721133 ) ) ;
#27792=VECTOR ( 'NONE', #4142, 39.37007874015748143 ) ;
#27795=CARTESIAN_POINT ( 'NONE',  ( -1.559171609364246924, 0.000000000000000000, 0.1028181436694137613 ) ) ;
#27807=DIRECTION ( 'NONE',  ( 1.000000000000000000, 0.000000000000000000, 3.455050906509825972E-15 ) ) ;
#27818=ORIENTED_EDGE ( 'NONE', *, *, #17674, .F. ) ;
#27824=CARTESIAN_POINT ( 'NONE',  ( -0.4418084573054544273, 1.710857756487497161, -2.620814421478965706 ) ) ;
#27830=CARTESIAN_POINT ( 'NONE',  ( 0.5314960629921349211, 2.729656593086051242, -2.556891438210025846 ) ) ;
#27842=EDGE_CURVE ( 'NONE', #60402, #50774, #37729, .T. ) ;
#27851=CARTESIAN_POINT ( 'NONE',  ( -0.5314960629921394730, 2.712230453466948799, 3.892840969167623566 ) ) ;
#27852=AXIS2_PLACEMENT_3D ( 'NONE', #26983, #69930, #52228 ) ;
#27855=CARTESIAN_POINT ( 'NONE',  ( 3.935132539805148433, 1.078793357725790658, 0.1224154028705949776 ) ) ;
#27872=CARTESIAN_POINT ( 'NONE',  ( -0.03156192328343619680, 1.063779846874849389, -1.121713509234345540 ) ) ;
#27874=CARTESIAN_POINT ( 'NONE',  ( -0.03443470937339728616, 0.2755905511811023723, -1.537015892239756099 ) ) ;
#27879=CARTESIAN_POINT ( 'NONE',  ( -0.03443470937339727228, 0.2929341459200028863, -1.438590695389362573 ) ) ;
#27891=CARTESIAN_POINT ( 'NONE',  ( 0.4585058784351956906, 1.414602624921270646, 3.910220467301401825 ) ) ;
#27908=CIRCLE ( 'NONE', #23873, 0.1771653543307085410 ) ;
#27913=ORIENTED_EDGE ( 'NONE', *, *, #49898, .T. ) ;
#27925=CARTESIAN_POINT ( 'NONE',  ( 0.06292302554185959240, 1.066149053166906002, 1.120702161501667238 ) ) ;
#27945=ORIENTED_EDGE ( 'NONE', *, *, #31423, .T. ) ;
#27948=DIRECTION ( 'NONE',  ( -0.000000000000000000, -1.000000000000000000, -0.000000000000000000 ) ) ;
#27949=CARTESIAN_POINT ( 'NONE',  ( -1.559171609364246924, 0.3937007874015748254, 0.4177787735906735578 ) ) ;
#27950=CARTESIAN_POINT ( 'NONE',  ( 0.000000000000000000, 2.559055118110236560, 0.000000000000000000 ) ) ;
#27952=CARTESIAN_POINT ( 'NONE',  ( 0.4423023948155340168, 1.709706175544221329, -3.912088937888734907 ) ) ;
#27955=EDGE_LOOP ( 'NONE', ( #48820, #10817, #8979, #60911 ) ) ;
#27965=VERTEX_POINT ( 'NONE', #56298 ) ;
#27967=CARTESIAN_POINT ( 'NONE',  ( -0.03443470937339728616, 1.062992125984252079, -1.537015892239756099 ) ) ;
#28024=ORIENTED_EDGE ( 'NONE', *, *, #42584, .F. ) ;
#28043=ORIENTED_EDGE ( 'NONE', *, *, #30705, .T. ) ;
#28044=CARTESIAN_POINT ( 'NONE',  ( 0.000000000000000000, 2.716535433070866645, 0.000000000000000000 ) ) ;
#28049=CARTESIAN_POINT ( 'NONE',  ( 1.018715732779042815, 1.601535527459639452, -0.4703312907311759106 ) ) ;
#28057=EDGE_CURVE ( 'NONE', #41276, #31528, #14989, .T. ) ;
#28064=DIRECTION ( 'NONE',  ( 1.000000000000000000, 0.000000000000000000, 0.000000000000000000 ) ) ;
#28093=ADVANCED_FACE ( 'NONE', ( #50798 ), #10832, .T. ) ;
#28101=VERTEX_POINT ( 'NONE', #68937 ) ;
#28114=CARTESIAN_POINT ( 'NONE',  ( -3.892840969167625786, 2.712230453466949687, -0.5314960629921260393 ) ) ;
#28147=CARTESIAN_POINT ( 'NONE',  ( 2.872342878167411406, 1.064797240280315194, 0.04222672046126994816 ) ) ;
#28181=DIRECTION ( 'NONE',  ( 0.000000000000000000, -0.6427876096865392519, -0.7660444431189781245 ) ) ;
#28187=CARTESIAN_POINT ( 'NONE',  ( -2.105021046755463754, 1.366082762360717018, -0.4426340671871326071 ) ) ;
#28211=DIRECTION ( 'NONE',  ( -0.000000000000000000, -1.000000000000000000, -1.408710688920637755E-15 ) ) ;
#28212=ORIENTED_EDGE ( 'NONE', *, *, #4866, .T. ) ;
#28217=LINE ( 'NONE', #47987, #14949 ) ;
#28221=DIRECTION ( 'NONE',  ( -0.000000000000000000, -1.000000000000000000, -0.000000000000000000 ) ) ;
#28226=EDGE_LOOP ( 'NONE', ( #77924, #41682, #38583, #57737 ) ) ;
#28229=VERTEX_POINT ( 'NONE', #63441 ) ;
#28235=CARTESIAN_POINT ( 'NONE',  ( 0.03775315452881272682, 1.064486638582849531, -1.473643470224546892 ) ) ;
#28241=CARTESIAN_POINT ( 'NONE',  ( 0.5314960629921349211, 2.716535433070866645, -2.543486866223387377 ) ) ;
#28264=CARTESIAN_POINT ( 'NONE',  ( 3.934091615812861154, 1.087812615256082083, 0.1522392691923797337 ) ) ;
#28274=PLANE ( 'NONE',  #82173 ) ;
#28297=CARTESIAN_POINT ( 'NONE',  ( 6.267877385347666114E-17, 1.062992125984252745, 2.874015748031495843 ) ) ;
#28306=DIRECTION ( 'NONE',  ( -1.000000000000000000, 0.000000000000000000, 0.000000000000000000 ) ) ;
#28313=AXIS2_PLACEMENT_3D ( 'NONE', #2905, #74440, #47914 ) ;
#28315=DIRECTION ( 'NONE',  ( 0.000000000000000000, 0.000000000000000000, 1.000000000000000000 ) ) ;
#28328=CARTESIAN_POINT ( 'NONE',  ( 6.267877318470707138E-17, 0.000000000000000000, -1.850393700787401619 ) ) ;
#28336=ADVANCED_FACE ( 'NONE', ( #18827 ), #5777, .F. ) ;
#28352=DIRECTION ( 'NONE',  ( 0.8660254037844363761, 0.000000000000000000, 0.5000000000000038858 ) ) ;
#28361=DIRECTION ( 'NONE',  ( 0.000000000000000000, 0.000000000000000000, 1.000000000000000000 ) ) ;
#28362=DIRECTION ( 'NONE',  ( 0.000000000000000000, 0.000000000000000000, -1.000000000000000000 ) ) ;
#28368=VERTEX_POINT ( 'NONE', #25960 ) ;
#28371=CARTESIAN_POINT ( 'NONE',  ( -1.096639669977155007, 1.126360982307443415, 0.2389055636428836504 ) ) ;
#28372=DIRECTION ( 'NONE',  ( 0.000000000000000000, 1.000000000000000000, 0.000000000000000000 ) ) ;
#28375=DIRECTION ( 'NONE',  ( -0.000000000000000000, 1.000000000000000000, -0.000000000000000000 ) ) ;
#28378=DIRECTION ( 'NONE',  ( 0.000000000000000000, 0.000000000000000000, -1.000000000000000000 ) ) ;
#28386=DIRECTION ( 'NONE',  ( 0.000000000000000000, -0.000000000000000000, -1.000000000000000000 ) ) ;
#28390=AXIS2_PLACEMENT_3D ( 'NONE', #16080, #36246, #22790 ) ;
#28396=PLANE ( 'NONE',  #4095 ) ;
#28410=CARTESIAN_POINT ( 'NONE',  ( -0.03443470937339727228, 1.062992125984252079, -1.438590695389362573 ) ) ;
#28427=CARTESIAN_POINT ( 'NONE',  ( -2.503252890251015828, 2.755905511811024056, 0.5314960629921260393 ) ) ;
#28440=ORIENTED_EDGE ( 'NONE', *, *, #23397, .F. ) ;
#28456=ORIENTED_EDGE ( 'NONE', *, *, #56394, .T. ) ;
#28459=CARTESIAN_POINT ( 'NONE',  ( -2.118110236220467790, 0.000000000000000000, -0.4498537592783120598 ) ) ;
#28472=CARTESIAN_POINT ( 'NONE',  ( 0.5314960629921393620, 2.755400581649068315, -3.831845081856512181 ) ) ;
#28473=ORIENTED_EDGE ( 'NONE', *, *, #7888, .F. ) ;
#28474=ADVANCED_FACE ( 'NONE', ( #65117 ), #41410, .F. ) ;
#28501=EDGE_CURVE ( 'NONE', #74653, #25219, #41811, .T. ) ;
#28505=EDGE_CURVE ( 'NONE', #63201, #53272, #68215, .T. ) ;
#28529=CARTESIAN_POINT ( 'NONE',  ( 0.000000000000000000, 2.559055118110236560, 0.000000000000000000 ) ) ;
#28535=DIRECTION ( 'NONE',  ( 0.000000000000000000, 1.000000000000000000, -8.673617379884024625E-16 ) ) ;
#28539=ORIENTED_EDGE ( 'NONE', *, *, #238, .F. ) ;
#28558=ORIENTED_EDGE ( 'NONE', *, *, #4397, .T. ) ;
#28563=CARTESIAN_POINT ( 'NONE',  ( 2.874027875014219635, 1.062979042929935503, 0.007789085821686646954 ) ) ;
#28569=CARTESIAN_POINT ( 'NONE',  ( -0.4677827689124922084, 0.03937007874015747977, 2.154527559055118946 ) ) ;
#28577=ORIENTED_EDGE ( 'NONE', *, *, #22453, .T. ) ;
#28604=CARTESIAN_POINT ( 'NONE',  ( -1.964921794496046648, 1.189595890467119776, -0.3229789317950364502 ) ) ;
#28630=CARTESIAN_POINT ( 'NONE',  ( -0.6299212598425062426, 2.755905511811024056, -3.886287458032464226 ) ) ;
#28632=ADVANCED_FACE ( 'NONE', ( #51618 ), #60583, .F. ) ;
#28637=DIRECTION ( 'NONE',  ( 0.000000000000000000, 0.000000000000000000, -1.000000000000000000 ) ) ;
#28640=CARTESIAN_POINT ( 'NONE',  ( 0.9881811337016640495, 2.559055118110236560, -0.5314960629921260393 ) ) ;
#28654=CARTESIAN_POINT ( 'NONE',  ( 0.05186593092965807728, 1.065829223649503277, -1.574764142214714946 ) ) ;
#28659=DIRECTION ( 'NONE',  ( 0.000000000000000000, -0.000000000000000000, 1.000000000000000000 ) ) ;
#28683=CARTESIAN_POINT ( 'NONE',  ( 3.927338144698056421, 1.151278041681430553, 0.2760671784697421582 ) ) ;
#28699=CARTESIAN_POINT ( 'NONE',  ( -0.3575568722600962479, 1.224102705420558435, -1.063793812528210703 ) ) ;
#28715=CARTESIAN_POINT ( 'NONE',  ( 1.348312163386739426, 0.000000000000000000, 0.7386866130305692613 ) ) ;
#28725=VECTOR ( 'NONE', #81989, 39.37007874015748143 ) ;
#28735=DIRECTION ( 'NONE',  ( 0.000000000000000000, 0.000000000000000000, -1.000000000000000000 ) ) ;
#28740=EDGE_LOOP ( 'NONE', ( #32604, #37021, #56090, #698, #55412, #55823, #71331, #55002 ) ) ;
#28744=CARTESIAN_POINT ( 'NONE',  ( 3.896872718254346779, 2.702643891907236640, -0.5314960629921260393 ) ) ;
#28766=CIRCLE ( 'NONE', #65055, 3.937007874015748143 ) ;
#28769=CARTESIAN_POINT ( 'NONE',  ( -0.1181161979004358292, 1.077624259009879459, -2.860481230828558985 ) ) ;
#28771=B_SPLINE_CURVE_WITH_KNOTS ( 'NONE', 3,
 ( #81450, #11150, #75132, #17477, #36808, #30497, #70030, #17883, #5237, #56568, #24587, #75952, #43936, #69630, #11975, #37630, #5644, #50664, #76364, #61976, #41380, #10645, #55232, #16552, #9806, #68308 ),
 .UNSPECIFIED., .F., .F.,
 ( 4, 2, 2, 2, 2, 2, 2, 2, 2, 2, 2, 2, 4 ),
 ( 0.05717903794320495364, 0.05955951868967798712, 0.06193999943615102061, 0.06313023980938753388, 0.06432048018262405409, 0.06670096092909708063, 0.06789120130233358696, 0.06908144167557010717, 0.07027168204880662739, 0.07146192242204313372, 0.07384240316851617414, 0.07503264354175269435, 0.07622288391498921456 ),
 .UNSPECIFIED. ) ;
#28773=EDGE_LOOP ( 'NONE', ( #52014, #63798, #9434, #80249, #47903 ) ) ;
#28779=DIRECTION ( 'NONE',  ( 0.8660254037844362651, 0.000000000000000000, 0.5000000000000041078 ) ) ;
#28780=DIRECTION ( 'NONE',  ( -0.000000000000000000, 1.000000000000000000, -0.000000000000000000 ) ) ;
#28782=TOROIDAL_SURFACE ( 'NONE', #46253, 3.858267716535433323, 0.07874015748031495954 ) ;
#28787=ORIENTED_EDGE ( 'NONE', *, *, #61511, .F. ) ;
#28790=CARTESIAN_POINT ( 'NONE',  ( 6.267877318470705905E-17, 1.929133858267716661, -1.850393700787401619 ) ) ;
#28811=EDGE_CURVE ( 'NONE', #55851, #52658, #64690, .T. ) ;
#28821=EDGE_CURVE ( 'NONE', #50709, #19542, #40078, .T. ) ;
#28823=DIRECTION ( 'NONE',  ( -0.000000000000000000, -1.000000000000000000, -0.000000000000000000 ) ) ;
#28839=AXIS2_PLACEMENT_3D ( 'NONE', #34373, #4041, #41917 ) ;
#28842=CARTESIAN_POINT ( 'NONE',  ( -0.4359958488159628165, 1.724409448818897905, -2.630268417803939940 ) ) ;
#28853=CARTESIAN_POINT ( 'NONE',  ( 0.5314960629921395840, 2.677165354330708791, -3.900966923095588346 ) ) ;
#28855=ORIENTED_EDGE ( 'NONE', *, *, #59902, .F. ) ;
#28871=VERTEX_POINT ( 'NONE', #45314 ) ;
#28874=CARTESIAN_POINT ( 'NONE',  ( -1.637380676922836731, 1.357125752008925268, 0.4389107506287909244 ) ) ;
#28878=CARTESIAN_POINT ( 'NONE',  ( 1.016821367227983774, 1.553403318890016704, -0.4744094488188971281 ) ) ;
#28904=AXIS2_PLACEMENT_3D ( 'NONE', #30841, #31250, #43869 ) ;
#28925=DIRECTION ( 'NONE',  ( -0.000000000000000000, 1.000000000000000000, 0.000000000000000000 ) ) ;
#28937=CARTESIAN_POINT ( 'NONE',  ( -0.5314960629921346991, 2.755905511811024056, 2.503252890251014939 ) ) ;
#28938=ADVANCED_FACE ( 'NONE', ( #42641 ), #75066, .F. ) ;
#28941=ADVANCED_FACE ( 'NONE', ( #68338 ), #56503, .F. ) ;
#28945=EDGE_CURVE ( 'NONE', #49366, #50786, #23959, .T. ) ;
#28948=DIRECTION ( 'NONE',  ( 0.000000000000000000, 8.673617379884024625E-16, 1.000000000000000000 ) ) ;
#28964=EDGE_CURVE ( 'NONE', #42501, #49642, #82205, .T. ) ;
#28967=ORIENTED_EDGE ( 'NONE', *, *, #33956, .T. ) ;
#28969=ORIENTED_EDGE ( 'NONE', *, *, #60504, .F. ) ;
#28978=CARTESIAN_POINT ( 'NONE',  ( -0.4744094488188934089, 1.537401574803149984, -1.016821367227985551 ) ) ;
#28983=ORIENTED_EDGE ( 'NONE', *, *, #59891, .T. ) ;
#28985=DIRECTION ( 'NONE',  ( 0.000000000000000000, 1.000000000000000000, 0.000000000000000000 ) ) ;
#29014=CARTESIAN_POINT ( 'NONE',  ( -1.895263394252401090, 1.111778211650215509, -0.2101609992702490048 ) ) ;
#29024=EDGE_CURVE ( 'NONE', #27310, #9114, #48486, .T. ) ;
#29039=FACE_OUTER_BOUND ( 'NONE', #34449, .T. ) ;
#29040=ORIENTED_EDGE ( 'NONE', *, *, #25308, .T. ) ;
#29043=CARTESIAN_POINT ( 'NONE',  ( 0.2661270878686344821, 1.144642331940836755, -1.467344394069625579 ) ) ;
#29050=AXIS2_PLACEMENT_3D ( 'NONE', #49495, #11623, #54563 ) ;
#29051=AXIS2_PLACEMENT_3D ( 'NONE', #9162, #73131, #47438 ) ;
#29055=VERTEX_POINT ( 'NONE', #75479 ) ;
#29058=VERTEX_POINT ( 'NONE', #81383 ) ;
#29064=CARTESIAN_POINT ( 'NONE',  ( -0.4744094488188882464, 1.546091976385118194, -2.554262525012306551 ) ) ;
#29069=CARTESIAN_POINT ( 'NONE',  ( 0.2886821576726813499, 1.160628398849492315, -2.785086082795377393 ) ) ;
#29075=ORIENTED_EDGE ( 'NONE', *, *, #4265, .T. ) ;
#29099=EDGE_CURVE ( 'NONE', #13017, #2386, #83295, .T. ) ;
#29103=CARTESIAN_POINT ( 'NONE',  ( 0.5314960629921373636, 2.729657712569141026, -3.237502114873378023 ) ) ;
#29106=ADVANCED_FACE ( 'NONE', ( #3943 ), #22876, .F. ) ;
#29119=VECTOR ( 'NONE', #39758, 39.37007874015748143 ) ;
#29137=ADVANCED_FACE ( 'NONE', ( #36333 ), #18929, .T. ) ;
#29145=DIRECTION ( 'NONE',  ( 0.000000000000000000, 0.000000000000000000, 1.000000000000000000 ) ) ;
#29173=AXIS2_PLACEMENT_3D ( 'NONE', #57732, #5985, #5167 ) ;
#29174=CIRCLE ( 'NONE', #70809, 0.1978346456692914035 ) ;
#29185=CARTESIAN_POINT ( 'NONE',  ( -0.4477123500621962293, 1.379796003448452435, -2.610391114557127690 ) ) ;
#29189=VERTEX_POINT ( 'NONE', #30429 ) ;
#29193=DIRECTION ( 'NONE',  ( -8.673617379884022653E-16, 1.000000000000000000, -3.028377322213053966E-30 ) ) ;
#29194=CARTESIAN_POINT ( 'NONE',  ( 4.773229650219999425E-16, 0.000000000000000000, -3.858267716535433323 ) ) ;
#29196=CARTESIAN_POINT ( 'NONE',  ( -0.4359958488159856316, 1.724409448818897905, 3.912791665790197992 ) ) ;
#29206=CARTESIAN_POINT ( 'NONE',  ( -1.111516660996405559, 1.088445792224367326, 0.1541100987596267513 ) ) ;
#29211=FACE_BOUND ( 'NONE', #72022, .T. ) ;
#29221=FACE_BOUND ( 'NONE', #40771, .T. ) ;
#29228=CIRCLE ( 'NONE', #76276, 2.598425196850393970 ) ;
#29234=DIRECTION ( 'NONE',  ( 1.000000000000000000, -0.000000000000000000, -0.000000000000000000 ) ) ;
#29241=CARTESIAN_POINT ( 'NONE',  ( -6.686372609646914991E-25, 1.062992125984252745, 1.850393700787401619 ) ) ;
#29244=LINE ( 'NONE', #24465, #23248 ) ;
#29246=ORIENTED_EDGE ( 'NONE', *, *, #67169, .T. ) ;
#29271=B_SPLINE_CURVE_WITH_KNOTS ( 'NONE', 3,
 ( #55322, #42697, #67978, #17058, #17875, #43509, #50246, #80620, #68394, #10733, #23757, #75942 ),
 .UNSPECIFIED., .F., .F.,
 ( 4, 2, 2, 2, 2, 4 ),
 ( 0.007992874908874989665, 0.009303755029337034896, 0.01061463514979908013, 0.01192551527026112709, 0.01258095533049215925, 0.01323639539072319141 ),
 .UNSPECIFIED. ) ;
#29278=DIRECTION ( 'NONE',  ( 9.381338752702757898E-17, -0.6427876096865366984, 0.7660444431189802339 ) ) ;
#29289=ORIENTED_EDGE ( 'NONE', *, *, #65634, .T. ) ;
#29293=AXIS2_PLACEMENT_3D ( 'NONE', #35767, #36175, #61848 ) ;
#29297=DIRECTION ( 'NONE',  ( 0.000000000000000000, 1.000000000000000000, 0.000000000000000000 ) ) ;
#29307=EDGE_LOOP ( 'NONE', ( #76060, #8054, #13747, #44381 ) ) ;
#29309=DIRECTION ( 'NONE',  ( -0.000000000000000000, -1.000000000000000000, -0.000000000000000000 ) ) ;
#29317=DIRECTION ( 'NONE',  ( 0.8660254037844363761, 0.000000000000000000, 0.5000000000000038858 ) ) ;
#29318=CARTESIAN_POINT ( 'NONE',  ( -0.4603267246303611726, 1.653225543546885223, 2.586063147568501641 ) ) ;
#29357=DIRECTION ( 'NONE',  ( 0.000000000000000000, 0.000000000000000000, -1.000000000000000000 ) ) ;
#29387=CARTESIAN_POINT ( 'NONE',  ( -1.393803226718939747, 1.220767705744369547, 0.3535424564827598926 ) ) ;
#29400=DIRECTION ( 'NONE',  ( 1.000000000000000000, 0.000000000000000000, 3.455050906509825972E-15 ) ) ;
#29420=EDGE_CURVE ( 'NONE', #46648, #32589, #74052, .T. ) ;
#29427=CARTESIAN_POINT ( 'NONE',  ( -1.851423525050897689, 1.064103292658516331, 0.03357545743410488698 ) ) ;
#29460=DIRECTION ( 'NONE',  ( 0.000000000000000000, 1.000000000000000000, -0.000000000000000000 ) ) ;
#29467=VERTEX_POINT ( 'NONE', #22504 ) ;
#29487=VERTEX_POINT ( 'NONE', #27566 ) ;
#29514=CARTESIAN_POINT ( 'NONE',  ( 0.5314960629921373636, 2.755905511811024056, -3.264097702071371288 ) ) ;
#29518=CARTESIAN_POINT ( 'NONE',  ( 0.000000000000000000, 0.000000000000000000, 0.000000000000000000 ) ) ;
#29542=DIRECTION ( 'NONE',  ( -3.491481338843132961E-15, -0.000000000000000000, 1.000000000000000000 ) ) ;
#29554=CARTESIAN_POINT ( 'NONE',  ( -0.5314960629921171575, 2.716535433070866645, -2.543486866223390930 ) ) ;
#29568=ADVANCED_FACE ( 'NONE', ( #1494 ), #28396, .F. ) ;
#29578=CARTESIAN_POINT ( 'NONE',  ( 0.4744094488188841940, 1.569669905603892524, 3.908320185825794990 ) ) ;
#29592=CARTESIAN_POINT ( 'NONE',  ( -0.3336463653987898903, 1.199832043049264163, -2.750549046294851419 ) ) ;
#29594=DIRECTION ( 'NONE',  ( -0.000000000000000000, -1.000000000000000000, -0.000000000000000000 ) ) ;
#29599=VERTEX_POINT ( 'NONE', #54054 ) ;
#29603=CARTESIAN_POINT ( 'NONE',  ( 1.141392835773559211, 0.000000000000000000, 1.141392835773562764 ) ) ;
#29620=CARTESIAN_POINT ( 'NONE',  ( 1.827151662668104581, 2.742788190551038952, 0.5314960629921260393 ) ) ;
#29638=CARTESIAN_POINT ( 'NONE',  ( -0.4703312907311723579, 1.601535527459639896, -1.018715732779044592 ) ) ;
#29666=EDGE_CURVE ( 'NONE', #22431, #6368, #59145, .T. ) ;
#29681=B_SPLINE_CURVE_WITH_KNOTS ( 'NONE', 3,
 ( #48387, #35773, #43709, #68994 ),
 .UNSPECIFIED., .F., .F.,
 ( 4, 4 ),
 ( 0.2189251788971746659, 0.2203393341987958387 ),
 .UNSPECIFIED. ) ;
#29687=DIRECTION ( 'NONE',  ( 0.000000000000000000, 0.000000000000000000, 1.000000000000000000 ) ) ;
#29692=AXIS2_PLACEMENT_3D ( 'NONE', #48538, #74238, #24523 ) ;
#29698=ORIENTED_EDGE ( 'NONE', *, *, #34592, .F. ) ;
#29706=CARTESIAN_POINT ( 'NONE',  ( 0.5314960629921396951, 2.559055118110236560, -3.937007874015760578 ) ) ;
#29714=AXIS2_PLACEMENT_3D ( 'NONE', #36188, #17271, #28637 ) ;
#29745=CARTESIAN_POINT ( 'NONE',  ( -3.898413161119330450, 2.697625129285034173, 0.5314960629921259283 ) ) ;
#29748=AXIS2_PLACEMENT_3D ( 'NONE', #12580, #6671, #5434 ) ;
#29749=ORIENTED_EDGE ( 'NONE', *, *, #75585, .T. ) ;
#29786=B_SPLINE_CURVE_WITH_KNOTS ( 'NONE', 3,
 ( #43799, #69503, #30780, #57678, #11438, #11852, #64006, #18166, #5113, #76641, #38748, #24048, #77057, #5927, #70743, #70316, #69904, #51354, #25693, #6347, #75825, #50944, #63180, #18972, #37094, #37505 ),
 .UNSPECIFIED., .F., .F.,
 ( 4, 2, 2, 2, 2, 2, 2, 2, 2, 2, 2, 2, 4 ),
 ( 0.01885843700256156080, 0.02003653724487836768, 0.02121463748719517803, 0.02357083797182877444, 0.02474893821414556744, 0.02592703845646236738, 0.02828323894109595685, 0.03063943942572954632, 0.03181753966804633932, 0.03299563991036313232, 0.03535184039499672526, 0.03652994063731351826, 0.03770804087963031126 ),
 .UNSPECIFIED. ) ;
#29789=ORIENTED_EDGE ( 'NONE', *, *, #55183, .T. ) ;
#29800=CARTESIAN_POINT ( 'NONE',  ( 0.4702942589932804229, 1.601810907557264851, 1.018732849840053634 ) ) ;
#29805=EDGE_LOOP ( 'NONE', ( #82297, #7968, #78768, #81918 ) ) ;
#29808=VERTEX_POINT ( 'NONE', #71073 ) ;
#29814=CARTESIAN_POINT ( 'NONE',  ( -0.1232739590129246776, 1.078238888412932583, 3.935195127778579938 ) ) ;
#29829=DIRECTION ( 'NONE',  ( -0.000000000000000000, -1.000000000000000000, 0.000000000000000000 ) ) ;
#29834=CARTESIAN_POINT ( 'NONE',  ( -2.000606668791069076, 1.230840736495002030, 0.3632157284009445153 ) ) ;
#29852=PLANE ( 'NONE',  #53498 ) ;
#29859=ORIENTED_EDGE ( 'NONE', *, *, #8199, .F. ) ;
#29868=DIRECTION ( 'NONE',  ( 0.000000000000000000, -1.000000000000000000, 0.000000000000000000 ) ) ;
#29875=VERTEX_POINT ( 'NONE', #369 ) ;
#29889=ORIENTED_EDGE ( 'NONE', *, *, #50692, .T. ) ;
#29892=ORIENTED_EDGE ( 'NONE', *, *, #57258, .F. ) ;
#29917=VECTOR ( 'NONE', #77654, 39.37007874015748143 ) ;
#29927=CARTESIAN_POINT ( 'NONE',  ( -2.841478809456101207, 1.098283573398291413, -0.1802708669123563034 ) ) ;
#29930=CARTESIAN_POINT ( 'NONE',  ( -0.1023049608108107106, 1.074140789190347389, -1.493476385750995394 ) ) ;
#29939=CARTESIAN_POINT ( 'NONE',  ( 0.4744094488189011249, 1.505635681685443039, -1.016821367227981776 ) ) ;
#29942=B_SPLINE_CURVE_WITH_KNOTS ( 'NONE', 3,
 ( #24103, #4746, #19446, #43445, #44676, #81792, #30831, #50996 ),
 .UNSPECIFIED., .F., .F.,
 ( 4, 2, 2, 4 ),
 ( 0.03284617093396371978, 0.03527709790192264105, 0.03649256138590211557, 0.03770802486988159008 ),
 .UNSPECIFIED. ) ;
#29955=AXIS2_PLACEMENT_3D ( 'NONE', #76632, #31173, #18563 ) ;
#29961=CARTESIAN_POINT ( 'NONE',  ( -1.681781318038497730, 1.161248049485916312, 0.2892642709497436071 ) ) ;
#29962=CARTESIAN_POINT ( 'NONE',  ( 3.937007874015748143, 2.755905511811024056, -0.5314960629921260393 ) ) ;
#29986=ADVANCED_FACE ( 'NONE', ( #69822 ), #39072, .F. ) ;
#30001=CARTESIAN_POINT ( 'NONE',  ( -0.6299212598425332210, 2.165354330708661568, 3.886287458032460229 ) ) ;
#30006=ORIENTED_EDGE ( 'NONE', *, *, #58860, .T. ) ;
#30007=EDGE_CURVE ( 'NONE', #2585, #46748, #19717, .T. ) ;
#30011=CARTESIAN_POINT ( 'NONE',  ( -1.016821367227983997, 1.537401574803149984, 0.4744094488188970171 ) ) ;
#30012=CARTESIAN_POINT ( 'NONE',  ( -3.224202737261815166, 2.716535433070866645, -0.5314960629921260393 ) ) ;
#30015=CARTESIAN_POINT ( 'NONE',  ( 0.4563452811745912219, 0.01305114060239447385, -2.130073781772667374 ) ) ;
#30019=CIRCLE ( 'NONE', #25989, 3.228346456692913424 ) ;
#30048=CARTESIAN_POINT ( 'NONE',  ( 0.000000000000000000, 2.677165354330708791, 0.000000000000000000 ) ) ;
#30094=CIRCLE ( 'NONE', #62356, 0.09842519685039351207 ) ;
#30111=VERTEX_POINT ( 'NONE', #63915 ) ;
#30112=DIRECTION ( 'NONE',  ( -0.000000000000000000, -1.000000000000000000, -0.000000000000000000 ) ) ;
#30134=CARTESIAN_POINT ( 'NONE',  ( 0.5314960629921064994, 2.716535433070866645, 1.854472803289057836 ) ) ;
#30142=AXIS2_PLACEMENT_3D ( 'NONE', #18747, #43575, #82323 ) ;
#30188=ORIENTED_EDGE ( 'NONE', *, *, #79291, .F. ) ;
#30201=ORIENTED_EDGE ( 'NONE', *, *, #7741, .F. ) ;
#30206=CARTESIAN_POINT ( 'NONE',  ( 0.000000000000000000, 1.062992125984252745, 1.122047244094488194 ) ) ;
#30211=AXIS2_PLACEMENT_3D ( 'NONE', #55779, #17514, #63343 ) ;
#30217=CARTESIAN_POINT ( 'NONE',  ( 3.916359054710398357, 1.286266870969481779, 0.4027888758938074076 ) ) ;
#30219=VERTEX_POINT ( 'NONE', #12171 ) ;
#30221=CARTESIAN_POINT ( 'NONE',  ( -2.118110236220467790, 0.000000000000000000, -0.4498537592783120598 ) ) ;
#30238=EDGE_CURVE ( 'NONE', #73035, #80330, #5837, .T. ) ;
#30245=DIRECTION ( 'NONE',  ( 1.000000000000000000, 1.601283208593975810E-15, 0.000000000000000000 ) ) ;
#30256=DIRECTION ( 'NONE',  ( -3.491481338843132961E-15, -0.000000000000000000, 1.000000000000000000 ) ) ;
#30265=DIRECTION ( 'NONE',  ( -0.000000000000000000, 1.000000000000000000, -1.408710688920637755E-15 ) ) ;
#30269=AXIS2_PLACEMENT_3D ( 'NONE', #68418, #17496, #29687 ) ;
#30278=DIRECTION ( 'NONE',  ( 0.000000000000000000, 0.000000000000000000, -1.000000000000000000 ) ) ;
#30281=DIRECTION ( 'NONE',  ( -0.000000000000000000, -1.000000000000000000, -0.000000000000000000 ) ) ;
#30285=EDGE_LOOP ( 'NONE', ( #24106, #48011, #67603, #82055 ) ) ;
#30294=CYLINDRICAL_SURFACE ( 'NONE', #17173, 0.1771653543307085410 ) ;
#30299=DIRECTION ( 'NONE',  ( 8.673617379884022653E-16, -1.000000000000000000, 3.028377322213053966E-30 ) ) ;
#30302=ORIENTED_EDGE ( 'NONE', *, *, #60079, .T. ) ;
#30323=EDGE_CURVE ( 'NONE', #15098, #11783, #25647, .T. ) ;
#30331=ADVANCED_FACE ( 'NONE', ( #38238, #37422, #63095 ), #6251, .F. ) ;
#30334=LINE ( 'NONE', #24429, #2863 ) ;
#30337=CARTESIAN_POINT ( 'NONE',  ( 0.4486317206264793800, 1.694949792723955850, -1.028546380722449527 ) ) ;
#30340=CARTESIAN_POINT ( 'NONE',  ( -2.829146054566457291, 1.111778211650234605, 0.2101609992702869745 ) ) ;
#30343=CARTESIAN_POINT ( 'NONE',  ( -0.1109781590376841404, 1.076155248315993074, -1.526021004911278567 ) ) ;
#30353=CARTESIAN_POINT ( 'NONE',  ( 0.4582086034426817722, 1.413485598871839555, -1.024236350951628571 ) ) ;
#30357=CARTESIAN_POINT ( 'NONE',  ( -0.03443470937339728616, 0.2755905511811023723, -1.537015892239756099 ) ) ;
#30364=CARTESIAN_POINT ( 'NONE',  ( 0.000000000000000000, 2.716535433070866645, 0.000000000000000000 ) ) ;
#30375=CARTESIAN_POINT ( 'NONE',  ( 0.3149606299212479033, -5.463695987328517809E-17, 1.076935383196061080 ) ) ;
#30381=AXIS2_PLACEMENT_3D ( 'NONE', #53607, #72571, #1456 ) ;
#30390=CARTESIAN_POINT ( 'NONE',  ( 2.118110236220470899, 0.000000000000000000, 0.4498537592782972383 ) ) ;
#30391=CARTESIAN_POINT ( 'NONE',  ( 0.5314960629921371416, 2.755905511811024056, -3.184294706754629001 ) ) ;
#30402=DIRECTION ( 'NONE',  ( 1.224646799147349509E-16, 0.000000000000000000, -1.000000000000000000 ) ) ;
#30403=ORIENTED_EDGE ( 'NONE', *, *, #17120, .T. ) ;
#30408=B_SPLINE_CURVE_WITH_KNOTS ( 'NONE', 3,
 ( #45801, #64761, #377, #58437, #33611, #78241, #7100, #26460, #52113, #77821, #20151, #71498, #27289, #1630, #39504, #20573, #65192, #7528, #33198, #14270, #58866, #1224, #26873, #71920, #46224 ),
 .UNSPECIFIED., .F., .F.,
 ( 4, 2, 2, 1, 2, 2, 2, 2, 2, 2, 2, 2, 4 ),
 ( 0.03770804087963031126, 0.04006530914106495866, 0.04124394327178228237, 0.04242257740249960607, 0.04360121153321692977, 0.04477984566393425347, 0.04713711392536890782, 0.04831574805608623846, 0.04949438218680355522, 0.05185165044823820957, 0.05303028457895553327, 0.05420891870967285697, 0.05656618697110752519 ),
 .UNSPECIFIED. ) ;
#30417=CARTESIAN_POINT ( 'NONE',  ( -0.01707598052245469858, 1.062992125984253411, -2.874015748031497175 ) ) ;
#30419=DIRECTION ( 'NONE',  ( 0.000000000000000000, 0.000000000000000000, -1.000000000000000000 ) ) ;
#30423=ORIENTED_EDGE ( 'NONE', *, *, #32224, .F. ) ;
#30424=CONICAL_SURFACE ( 'NONE', #77475, 0.09842519685039351207, 1.029744258676652091 ) ;
#30429=CARTESIAN_POINT ( 'NONE',  ( 1.374111566022513293E-16, 1.062992125984252745, -1.122047244094488194 ) ) ;
#30430=LINE ( 'NONE', #35510, #49190 ) ;
#30447=CIRCLE ( 'NONE', #55973, 0.5118110236220472231 ) ;
#30460=EDGE_CURVE ( 'NONE', #55363, #50475, #31094, .T. ) ;
#30465=CARTESIAN_POINT ( 'NONE',  ( 1.111517297590296494, 1.088444344143271847, 0.1541001657482228560 ) ) ;
#30484=EDGE_CURVE ( 'NONE', #22014, #52853, #41823, .T. ) ;
#30491=AXIS2_PLACEMENT_3D ( 'NONE', #12726, #68733, #30419 ) ;
#30492=CIRCLE ( 'NONE', #4956, 3.937007874015748143 ) ;
#30497=CARTESIAN_POINT ( 'NONE',  ( -0.4318705504292276176, 1.340445554703190378, 1.035625287865071353 ) ) ;
#30498=CARTESIAN_POINT ( 'NONE',  ( -0.5314960629921196000, 2.742788220949579081, -1.827151630990901054 ) ) ;
#30510=CARTESIAN_POINT ( 'NONE',  ( 0.4177787735907000366, 0.3937007874015747699, -1.559171609364239375 ) ) ;
#30527=ORIENTED_EDGE ( 'NONE', *, *, #2876, .T. ) ;
#30534=CARTESIAN_POINT ( 'NONE',  ( -0.5314960629921225976, 2.559055118110236560, -0.9881811337016657149 ) ) ;
#30536=CARTESIAN_POINT ( 'NONE',  ( 0.5314960629921323676, 2.729664702882089511, -1.840814949217402186 ) ) ;
#30545=CARTESIAN_POINT ( 'NONE',  ( 0.000000000000000000, 2.755905511811024056, 0.000000000000000000 ) ) ;
#30546=VECTOR ( 'NONE', #55229, 39.37007874015748143 ) ;
#30548=DIRECTION ( 'NONE',  ( 0.000000000000000000, 0.000000000000000000, 1.000000000000000000 ) ) ;
#30550=AXIS2_PLACEMENT_3D ( 'NONE', #7495, #64310, #57979 ) ;
#30551=DIRECTION ( 'NONE',  ( -3.491481338843132961E-15, -0.000000000000000000, 1.000000000000000000 ) ) ;
#30592=CARTESIAN_POINT ( 'NONE',  ( 0.1345703391920829439, 1.081211091791629109, 2.857167579953707737 ) ) ;
#30603=AXIS2_PLACEMENT_3D ( 'NONE', #78744, #66105, #59772 ) ;
#30606=EDGE_CURVE ( 'NONE', #3377, #30219, #52939, .T. ) ;
#30609=VERTEX_POINT ( 'NONE', #34436 ) ;
#30614=EDGE_CURVE ( 'NONE', #712, #60855, #12935, .T. ) ;
#30631=CARTESIAN_POINT ( 'NONE',  ( -0.4574207045264588878, 1.664236311372951471, -3.910347889586886172 ) ) ;
#30637=CARTESIAN_POINT ( 'NONE',  ( 3.935572654129527503, 1.075044193959341809, 0.1073736613157593028 ) ) ;
#30648=ADVANCED_FACE ( 'NONE', ( #58857 ), #10899, .F. ) ;
#30668=ADVANCED_FACE ( 'NONE', ( #66426, #46633, #1214, #9181, #33601 ), #15083, .F. ) ;
#30669=B_SPLINE_CURVE_WITH_KNOTS ( 'NONE', 3,
 ( #67836, #61089, #29103, #10175 ),
 .UNSPECIFIED., .F., .F.,
 ( 4, 4 ),
 ( 0.1000642744325471178, 0.1014879310549284402 ),
 .UNSPECIFIED. ) ;
#30688=CARTESIAN_POINT ( 'NONE',  ( -3.929901827426621530, 1.125753869628013160, -0.2378376118093886160 ) ) ;
#30693=ORIENTED_EDGE ( 'NONE', *, *, #41957, .F. ) ;
#30702=CARTESIAN_POINT ( 'NONE',  ( 0.4359958488159500489, 1.724409448818897905, 2.094141031014936871 ) ) ;
#30705=EDGE_CURVE ( 'NONE', #21301, #75845, #44069, .T. ) ;
#30724=ORIENTED_EDGE ( 'NONE', *, *, #46607, .F. ) ;
#30726=ORIENTED_EDGE ( 'NONE', *, *, #15919, .T. ) ;
#30728=CARTESIAN_POINT ( 'NONE',  ( -1.076935383196057749, 2.165354330708661568, 0.3149606299212595606 ) ) ;
#30759=CARTESIAN_POINT ( 'NONE',  ( -2.872985923768006877, 1.064103292658512556, -0.03357545743405447591 ) ) ;
#30762=DIRECTION ( 'NONE',  ( 1.000000000000000000, 0.000000000000000000, -1.224646799147353207E-16 ) ) ;
#30775=DIRECTION ( 'NONE',  ( -0.000000000000000000, -1.000000000000000000, -0.000000000000000000 ) ) ;
#30780=CARTESIAN_POINT ( 'NONE',  ( -0.4736533538817698230, 1.506391317405408214, -3.908412196150712781 ) ) ;
#30799=ORIENTED_EDGE ( 'NONE', *, *, #22798, .F. ) ;
#30814=CARTESIAN_POINT ( 'NONE',  ( -0.1654368116759051266, 1.092466590690397199, -1.877592342312344842 ) ) ;
#30815=VERTEX_POINT ( 'NONE', #4925 ) ;
#30818=EDGE_LOOP ( 'NONE', ( #5972, #72766, #80360, #56148 ) ) ;
#30831=CARTESIAN_POINT ( 'NONE',  ( 3.908320185825792326, 1.553377289108603732, -0.4744094488188970171 ) ) ;
#30834=VERTEX_POINT ( 'NONE', #28937 ) ;
#30838=CARTESIAN_POINT ( 'NONE',  ( 3.937007874015748143, 2.165354330708661568, -0.6299212598425196763 ) ) ;
#30841=CARTESIAN_POINT ( 'NONE',  ( 0.000000000000000000, 2.755905511811024056, 0.000000000000000000 ) ) ;
#30858=CARTESIAN_POINT ( 'NONE',  ( 0.5314960629920997270, 2.755905511811024056, 2.503252890251021601 ) ) ;
#30862=CARTESIAN_POINT ( 'NONE',  ( -0.5314960629921124946, 2.716724272663528783, -3.890406373195416379 ) ) ;
#30864=DIRECTION ( 'NONE',  ( 0.000000000000000000, 0.000000000000000000, -1.000000000000000000 ) ) ;
#30872=CARTESIAN_POINT ( 'NONE',  ( 1.109386689909465318, 1.093731576984011689, 0.1687003897380535689 ) ) ;
#30875=CARTESIAN_POINT ( 'NONE',  ( 0.4713260495230639502, 1.475165172288837923, 3.908697958268506856 ) ) ;
#30884=CARTESIAN_POINT ( 'NONE',  ( -0.5314960629921372526, 2.716535433070866645, 3.224202737261813834 ) ) ;
#30902=CARTESIAN_POINT ( 'NONE',  ( 0.000000000000000000, 2.165354330708661568, 0.000000000000000000 ) ) ;
#30913=CARTESIAN_POINT ( 'NONE',  ( -2.583694225513480713, 2.755905511811024056, 0.5314960629921260393 ) ) ;
#30932=EDGE_LOOP ( 'NONE', ( #44679, #8073, #77909, #71399 ) ) ;
#30938=CARTESIAN_POINT ( 'NONE',  ( -0.5314960629921146040, 2.729657713787763118, -3.237502116108450956 ) ) ;
#30948=DIRECTION ( 'NONE',  ( 0.000000000000000000, -0.000000000000000000, 1.000000000000000000 ) ) ;
#30993=CARTESIAN_POINT ( 'NONE',  ( 0.3443067643236821795, 1.210770866460127770, -1.397620821078814579 ) ) ;
#31008=ORIENTED_EDGE ( 'NONE', *, *, #29024, .T. ) ;
#31015=CIRCLE ( 'NONE', #68653, 1.122047244094488194 ) ;
#31022=ORIENTED_EDGE ( 'NONE', *, *, #41175, .F. ) ;
#31031=CARTESIAN_POINT ( 'NONE',  ( -0.9881811337016640495, 0.000000000000000000, 0.5314960629921260393 ) ) ;
#31049=CARTESIAN_POINT ( 'NONE',  ( -0.3133562546434896512, 1.179838254429707023, 3.924580492031178647 ) ) ;
#31058=EDGE_CURVE ( 'NONE', #19641, #28871, #76790, .T. ) ;
#31068=CARTESIAN_POINT ( 'NONE',  ( -1.894990545102987367, 1.111478976311921274, 0.2095522481616672039 ) ) ;
#31088=CARTESIAN_POINT ( 'NONE',  ( -3.918976913854863575, 1.248341192856212034, 0.3764949346671048747 ) ) ;
#31093=ORIENTED_EDGE ( 'NONE', *, *, #75321, .T. ) ;
#31094=LINE ( 'NONE', #56761, #18981 ) ;
#31100=CYLINDRICAL_SURFACE ( 'NONE', #61975, 0.1771653543307085410 ) ;
#31107=ORIENTED_EDGE ( 'NONE', *, *, #15715, .F. ) ;
#31117=CIRCLE ( 'NONE', #20383, 1.122047244094488194 ) ;
#31123=ORIENTED_EDGE ( 'NONE', *, *, #1221, .F. ) ;
#31125=ORIENTED_EDGE ( 'NONE', *, *, #4265, .F. ) ;
#31127=CARTESIAN_POINT ( 'NONE',  ( 2.869680830158524820, 1.067671560069316294, -0.06860298820096749628 ) ) ;
#31160=CARTESIAN_POINT ( 'NONE',  ( -2.610350574616450814, 1.379859446982315330, 0.4477348144951694420 ) ) ;
#31168=ADVANCED_FACE ( 'NONE', ( #44067 ), #44880, .F. ) ;
#31173=DIRECTION ( 'NONE',  ( -0.000000000000000000, -1.000000000000000000, -0.000000000000000000 ) ) ;
#31175=ADVANCED_FACE ( 'NONE', ( #76496 ), #43237, .F. ) ;
#31176=AXIS2_PLACEMENT_3D ( 'NONE', #49731, #57273, #25290 ) ;
#31183=B_SPLINE_CURVE_WITH_KNOTS ( 'NONE', 3,
 ( #901, #32444, #27384, #47151, #26967, #46321, #6772, #71175, #72014, #58106, #72432, #77493 ),
 .UNSPECIFIED., .F., .F.,
 ( 4, 2, 2, 2, 2, 4 ),
 ( 0.000000000000000000, 0.001328432419540427623, 0.002656864839080855245, 0.003985297258621282868, 0.004649513468391494944, 0.005313729678161706153 ),
 .UNSPECIFIED. ) ;
#31184=FACE_OUTER_BOUND ( 'NONE', #45644, .T. ) ;
#31198=CARTESIAN_POINT ( 'NONE',  ( 0.000000000000000000, 2.755905511811024056, 0.000000000000000000 ) ) ;
#31202=DIRECTION ( 'NONE',  ( 0.000000000000000000, 0.000000000000000000, -1.000000000000000000 ) ) ;
#31222=FACE_OUTER_BOUND ( 'NONE', #15936, .T. ) ;
#31243=ORIENTED_EDGE ( 'NONE', *, *, #17348, .F. ) ;
#31250=DIRECTION ( 'NONE',  ( 0.000000000000000000, 1.000000000000000000, -0.000000000000000000 ) ) ;
#31251=DIRECTION ( 'NONE',  ( -0.8660254037844432595, 0.000000000000000000, 0.4999999999999918954 ) ) ;
#31265=VECTOR ( 'NONE', #82673, 39.37007874015748143 ) ;
#31267=CARTESIAN_POINT ( 'NONE',  ( -0.2096960158929757345, 1.111548270248047476, 1.895053761512689894 ) ) ;
#31282=CARTESIAN_POINT ( 'NONE',  ( 0.000000000000000000, 2.716535433070866645, 0.000000000000000000 ) ) ;
#31293=CIRCLE ( 'NONE', #71628, 0.3149606299212597826 ) ;
#31312=CARTESIAN_POINT ( 'NONE',  ( 0.000000000000000000, 2.559055118110236560, 0.000000000000000000 ) ) ;
#31340=ORIENTED_EDGE ( 'NONE', *, *, #35777, .F. ) ;
#31346=DIRECTION ( 'NONE',  ( 0.000000000000000000, 1.000000000000000000, 1.734723475976808327E-16 ) ) ;
#31347=CARTESIAN_POINT ( 'NONE',  ( 0.5314960629921324786, 2.716535433070866645, -1.854472803289050509 ) ) ;
#31349=VECTOR ( 'NONE', #73680, 39.37007874015748143 ) ;
#31355=EDGE_LOOP ( 'NONE', ( #30423, #78330, #7642, #28983 ) ) ;
#31357=CYLINDRICAL_SURFACE ( 'NONE', #20562, 0.4744094488188972947 ) ;
#31360=CARTESIAN_POINT ( 'NONE',  ( -1.559171609364246924, 0.000000000000000000, 0.4177787735906735578 ) ) ;
#31362=EDGE_CURVE ( 'NONE', #46245, #65458, #60203, .T. ) ;
#31365=ORIENTED_EDGE ( 'NONE', *, *, #69234, .T. ) ;
#31393=ORIENTED_EDGE ( 'NONE', *, *, #58860, .F. ) ;
#31405=AXIS2_PLACEMENT_3D ( 'NONE', #15536, #2899, #79935 ) ;
#31407=CARTESIAN_POINT ( 'NONE',  ( 0.03412294937773927700, 1.063915752041795670, 2.873159270261472553 ) ) ;
#31423=EDGE_CURVE ( 'NONE', #16468, #69029, #37359, .T. ) ;
#31446=CARTESIAN_POINT ( 'NONE',  ( -0.3149606299212459048, 2.559055118110236560, -3.937007874015763242 ) ) ;
#31449=CONICAL_SURFACE ( 'NONE', #24722, 0.09842519685039351207, 1.029744258676651647 ) ;
#31453=VERTEX_POINT ( 'NONE', #58791 ) ;
#31483=CARTESIAN_POINT ( 'NONE',  ( -1.863753233923699737, 1.077434660671937161, 0.1173752429317948681 ) ) ;
#31507=CARTESIAN_POINT ( 'NONE',  ( 0.000000000000000000, 0.07874015748031502893, 0.000000000000000000 ) ) ;
#31511=DIRECTION ( 'NONE',  ( -0.000000000000000000, -1.000000000000000000, -0.000000000000000000 ) ) ;
#31517=DIRECTION ( 'NONE',  ( -0.000000000000000000, -1.000000000000000000, -0.000000000000000000 ) ) ;
#31521=PLANE ( 'NONE',  #1935 ) ;
#31528=VERTEX_POINT ( 'NONE', #723 ) ;
#31541=ORIENTED_EDGE ( 'NONE', *, *, #81099, .T. ) ;
#31543=ORIENTED_EDGE ( 'NONE', *, *, #67559, .F. ) ;
#31577=CARTESIAN_POINT ( 'NONE',  ( -2.822444539845162303, 1.119136672863575876, 0.2244172274865353089 ) ) ;
#31594=CARTESIAN_POINT ( 'NONE',  ( 0.1654213697349169176, 1.092461187568466219, -1.877587376364790339 ) ) ;
#31620=VERTEX_POINT ( 'NONE', #7875 ) ;
#31624=EDGE_CURVE ( 'NONE', #2780, #55113, #51168, .T. ) ;
#31659=ORIENTED_EDGE ( 'NONE', *, *, #38333, .T. ) ;
#31685=CARTESIAN_POINT ( 'NONE',  ( 0.5314960629921064994, 2.716535433070866645, 1.854472803289057836 ) ) ;
#31699=CARTESIAN_POINT ( 'NONE',  ( 1.030613340552999135, 1.368770328279408144, 0.4436984845053965065 ) ) ;
#31729=LINE ( 'NONE', #38456, #51975 ) ;
#31740=DIRECTION ( 'NONE',  ( 0.000000000000000000, 0.000000000000000000, -1.000000000000000000 ) ) ;
#31758=ORIENTED_EDGE ( 'NONE', *, *, #72915, .F. ) ;
#31762=CIRCLE ( 'NONE', #15695, 1.968503937007874072 ) ;
#31767=CARTESIAN_POINT ( 'NONE',  ( 0.000000000000000000, 0.07874015748031502893, 0.000000000000000000 ) ) ;
#31784=DIRECTION ( 'NONE',  ( -0.000000000000000000, -1.000000000000000000, -0.000000000000000000 ) ) ;
#31800=VECTOR ( 'NONE', #58221, 39.37007874015748143 ) ;
#31811=ORIENTED_EDGE ( 'NONE', *, *, #22393, .F. ) ;
#31825=CARTESIAN_POINT ( 'NONE',  ( 0.4567021909596065687, 1.408136488465070002, 2.593432289528808887 ) ) ;
#31829=CARTESIAN_POINT ( 'NONE',  ( -3.937007874015748143, 2.755905511811024056, -0.5314960629921260393 ) ) ;
#31850=VECTOR ( 'NONE', #1836, 39.37007874015748143 ) ;
#31853=ORIENTED_EDGE ( 'NONE', *, *, #47538, .F. ) ;
#31855=AXIS2_PLACEMENT_3D ( 'NONE', #31903, #76535, #32316 ) ;
#31857=LINE ( 'NONE', #77314, #56977 ) ;
#31859=AXIS2_PLACEMENT_3D ( 'NONE', #29518, #62327, #23613 ) ;
#31875=ORIENTED_EDGE ( 'NONE', *, *, #8916, .T. ) ;
#31882=CARTESIAN_POINT ( 'NONE',  ( 2.131037067002786944, 1.408244132531265791, 0.4567322424080934584 ) ) ;
#31903=CARTESIAN_POINT ( 'NONE',  ( 0.000000000000000000, 2.755905511811024056, 0.000000000000000000 ) ) ;
#31925=DIRECTION ( 'NONE',  ( 9.381338752702771457E-17, -0.6427876096865352551, 0.7660444431189814551 ) ) ;
#31927=ORIENTED_EDGE ( 'NONE', *, *, #45702, .F. ) ;
#31943=ORIENTED_EDGE ( 'NONE', *, *, #70814, .F. ) ;
#31958=ORIENTED_EDGE ( 'NONE', *, *, #59409, .F. ) ;
#31962=CARTESIAN_POINT ( 'NONE',  ( 2.867114984585486859, 1.070443199938755807, -0.08545185031212575166 ) ) ;
#31981=CONICAL_SURFACE ( 'NONE', #79064, 3.307086614173228689, 0.7853981633974500554 ) ;
#31995=CARTESIAN_POINT ( 'NONE',  ( -0.5314960629921122726, 2.755905511811024056, -3.937007874015763687 ) ) ;
#32018=LINE ( 'NONE', #64425, #66983 ) ;
#32031=LINE ( 'NONE', #30375, #9540 ) ;
#32040=EDGE_LOOP ( 'NONE', ( #30693, #77229, #39525, #51699 ) ) ;
#32047=DIRECTION ( 'NONE',  ( -0.000000000000000000, -1.000000000000000000, -0.000000000000000000 ) ) ;
#32056=CARTESIAN_POINT ( 'NONE',  ( -0.4426658557721557807, 1.366171107244632310, -2.105078266945731080 ) ) ;
#32057=VERTEX_POINT ( 'NONE', #9125 ) ;
#32072=PLANE ( 'NONE',  #39930 ) ;
#32074=CARTESIAN_POINT ( 'NONE',  ( 3.935112320374951178, 1.078966695441597512, -0.1230623252665035139 ) ) ;
#32076=VERTEX_POINT ( 'NONE', #53710 ) ;
#32101=EDGE_CURVE ( 'NONE', #65284, #9834, #66365, .T. ) ;
#32116=CARTESIAN_POINT ( 'NONE',  ( 1.057189182743691225, 1.247828027546490803, 0.3760955751420046456 ) ) ;
#32141=VECTOR ( 'NONE', #14018, 39.37007874015748143 ) ;
#32145=CARTESIAN_POINT ( 'NONE',  ( 3.910334576242769256, 1.663832811914786936, 0.4575345774109204622 ) ) ;
#32173=EDGE_CURVE ( 'NONE', #6265, #7002, #68844, .T. ) ;
#32190=ORIENTED_EDGE ( 'NONE', *, *, #55183, .F. ) ;
#32193=LINE ( 'NONE', #26290, #8954 ) ;
#32200=CARTESIAN_POINT ( 'NONE',  ( 0.000000000000000000, 0.000000000000000000, 1.850393700787401619 ) ) ;
#32216=EDGE_CURVE ( 'NONE', #12593, #9282, #31117, .T. ) ;
#32222=CARTESIAN_POINT ( 'NONE',  ( -3.937007874015748143, 2.559055118110236560, 0.5314960629921260393 ) ) ;
#32224=EDGE_CURVE ( 'NONE', #72153, #2295, #71069, .T. ) ;
#32227=ORIENTED_EDGE ( 'NONE', *, *, #53218, .F. ) ;
#32241=CARTESIAN_POINT ( 'NONE',  ( 0.000000000000000000, 0.000000000000000000, -3.444881889763779625 ) ) ;
#32254=ORIENTED_EDGE ( 'NONE', *, *, #73728, .F. ) ;
#32279=CARTESIAN_POINT ( 'NONE',  ( 0.4744094488188901337, 1.554943921348594493, 2.170146923806597350 ) ) ;
#32286=ORIENTED_EDGE ( 'NONE', *, *, #79536, .T. ) ;
#32306=CARTESIAN_POINT ( 'NONE',  ( -0.07064761070677771926, 1.068257286200871681, -1.454808247151501588 ) ) ;
#32316=DIRECTION ( 'NONE',  ( 0.000000000000000000, 0.000000000000000000, 1.000000000000000000 ) ) ;
#32317=ADVANCED_FACE ( 'NONE', ( #69260 ), #4453, .F. ) ;
#32319=CARTESIAN_POINT ( 'NONE',  ( -1.028550503362776425, 1.694972584785692904, -0.4486219446274117839 ) ) ;
#32325=DIRECTION ( 'NONE',  ( -0.000000000000000000, -1.000000000000000000, -0.000000000000000000 ) ) ;
#32341=ORIENTED_EDGE ( 'NONE', *, *, #68594, .F. ) ;
#32343=DIRECTION ( 'NONE',  ( -0.000000000000000000, 1.000000000000000000, 0.000000000000000000 ) ) ;
#32355=VERTEX_POINT ( 'NONE', #25029 ) ;
#32357=VERTEX_POINT ( 'NONE', #62942 ) ;
#32374=CARTESIAN_POINT ( 'NONE',  ( 2.557140022784311295, 1.502969453419624735, -0.4732359647714761697 ) ) ;
#32380=CARTESIAN_POINT ( 'NONE',  ( 0.5314960629921346991, 2.755905511811024056, -2.503252890251014495 ) ) ;
#32407=LINE ( 'NONE', #52173, #62816 ) ;
#32413=EDGE_CURVE ( 'NONE', #9951, #36503, #50038, .T. ) ;
#32431=DIRECTION ( 'NONE',  ( 0.000000000000000000, 0.000000000000000000, 1.000000000000000000 ) ) ;
#32440=VECTOR ( 'NONE', #14920, 39.37007874015748143 ) ;
#32444=CARTESIAN_POINT ( 'NONE',  ( 0.4418084573054713027, 1.710857756487497383, -2.103595027339961732 ) ) ;
#32445=CARTESIAN_POINT ( 'NONE',  ( -2.094141031015012366, 1.724409448818897905, 0.4359958488159718093 ) ) ;
#32471=CARTESIAN_POINT ( 'NONE',  ( -0.4252607725274083483, 1.326635381343780562, -2.077176919885365791 ) ) ;
#32472=VERTEX_POINT ( 'NONE', #82306 ) ;
#32488=FACE_OUTER_BOUND ( 'NONE', #57317, .T. ) ;
#32491=ORIENTED_EDGE ( 'NONE', *, *, #16141, .F. ) ;
#32492=ORIENTED_EDGE ( 'NONE', *, *, #65884, .T. ) ;
#32522=CARTESIAN_POINT ( 'NONE',  ( -0.4359958488159792478, 1.724409448818897683, 2.094141031014984389 ) ) ;
#32546=EDGE_CURVE ( 'NONE', #47373, #38086, #82215, .T. ) ;
#32558=LINE ( 'NONE', #70875, #31800 ) ;
#32589=VERTEX_POINT ( 'NONE', #19978 ) ;
#32596=CARTESIAN_POINT ( 'NONE',  ( -0.01711285633636233997, 1.063222675620814073, 2.873802023517004312 ) ) ;
#32597=DIRECTION ( 'NONE',  ( 0.000000000000000000, 0.000000000000000000, -1.000000000000000000 ) ) ;
#32604=ORIENTED_EDGE ( 'NONE', *, *, #19758, .F. ) ;
#32607=B_SPLINE_CURVE_WITH_KNOTS ( 'NONE', 3,
 ( #27497, #59483, #35063, #34656 ),
 .UNSPECIFIED., .F., .F.,
 ( 4, 4 ),
 ( 0.01019635767495674639, 0.01088423237384165791 ),
 .UNSPECIFIED. ) ;
#32642=ORIENTED_EDGE ( 'NONE', *, *, #4112, .T. ) ;
#32656=CARTESIAN_POINT ( 'NONE',  ( 1.028546380722451081, 1.694949792723957183, 0.4486317206264757718 ) ) ;
#32669=ORIENTED_EDGE ( 'NONE', *, *, #72215, .T. ) ;
#32670=VECTOR ( 'NONE', #82149, 39.37007874015748143 ) ;
#32687=CARTESIAN_POINT ( 'NONE',  ( -0.3149606299212553973, -5.463695987328517809E-17, -1.076935383196058860 ) ) ;
#32702=EDGE_CURVE ( 'NONE', #56386, #20489, #67439, .T. ) ;
#32713=CARTESIAN_POINT ( 'NONE',  ( -2.130163876374039589, 1.668131542012053048, 0.4562955581495582447 ) ) ;
#32739=CARTESIAN_POINT ( 'NONE',  ( -1.018733685929528399, 1.601836984657050378, -0.4702924666327328307 ) ) ;
#32746=DIRECTION ( 'NONE',  ( 0.000000000000000000, -1.000000000000000000, 0.000000000000000000 ) ) ;
#32755=LINE ( 'NONE', #27693, #81755 ) ;
#32761=ORIENTED_EDGE ( 'NONE', *, *, #44453, .T. ) ;
#32780=VECTOR ( 'NONE', #83209, 39.37007874015748143 ) ;
#32796=DIRECTION ( 'NONE',  ( 3.491481338843132961E-15, 0.000000000000000000, -1.000000000000000000 ) ) ;
#32801=CIRCLE ( 'NONE', #7273, 1.929133858267716661 ) ;
#32829=CARTESIAN_POINT ( 'NONE',  ( -2.554262525012343854, 1.528780496884629025, -0.4744094488188976277 ) ) ;
#32836=LINE ( 'NONE', #71562, #22053 ) ;
#32857=AXIS2_PLACEMENT_3D ( 'NONE', #53071, #77097, #7656 ) ;
#32861=VERTEX_POINT ( 'NONE', #57838 ) ;
#32867=CARTESIAN_POINT ( 'NONE',  ( -1.895394334970792016, 2.755905511811024056, 0.5314960629921260393 ) ) ;
#32872=LINE ( 'NONE', #51794, #14003 ) ;
#32876=ORIENTED_EDGE ( 'NONE', *, *, #42409, .F. ) ;
#32892=EDGE_CURVE ( 'NONE', #5361, #4140, #52432, .T. ) ;
#32896=EDGE_LOOP ( 'NONE', ( #34570, #6178, #73289, #7016 ) ) ;
#32914=CARTESIAN_POINT ( 'NONE',  ( -0.5314960629921393620, 2.755400581649068315, 3.831845081856512181 ) ) ;
#32917=VERTEX_POINT ( 'NONE', #52357 ) ;
#32935=DIRECTION ( 'NONE',  ( 0.000000000000000000, 1.000000000000000000, -0.000000000000000000 ) ) ;
#32952=CARTESIAN_POINT ( 'NONE',  ( 1.084078074602846664, 1.161389122953379260, -0.2896872109502376391 ) ) ;
#32955=CARTESIAN_POINT ( 'NONE',  ( 0.1527192119523664293, 1.087977008489718012, 3.934072827720677790 ) ) ;
#32968=CARTESIAN_POINT ( 'NONE',  ( 1.141392835773559211, 1.299212598425196985, 1.141392835773562764 ) ) ;
#32974=VECTOR ( 'NONE', #21571, 39.37007874015748143 ) ;
#32989=CARTESIAN_POINT ( 'NONE',  ( -0.4470386624395519815, 1.696927142811738287, -2.112798853176812042 ) ) ;
#33012=CARTESIAN_POINT ( 'NONE',  ( 1.530808498934191571E-16, 0.000000000000000000, 1.250000000000000000 ) ) ;
#33020=ORIENTED_EDGE ( 'NONE', *, *, #51302, .F. ) ;
#33030=AXIS2_PLACEMENT_3D ( 'NONE', #13259, #12418, #25439 ) ;
#33032=CARTESIAN_POINT ( 'NONE',  ( 0.000000000000000000, 2.559055118110236560, 0.000000000000000000 ) ) ;
#33047=ADVANCED_FACE ( 'NONE', ( #1048 ), #26702, .F. ) ;
#33064=ORIENTED_EDGE ( 'NONE', *, *, #70713, .T. ) ;
#33082=CARTESIAN_POINT ( 'NONE',  ( 0.4469586986358917158, 1.697151583350163806, 2.611754389584974856 ) ) ;
#33094=VECTOR ( 'NONE', #47723, 39.37007874015748143 ) ;
#33113=EDGE_LOOP ( 'NONE', ( #51123, #17614, #26039, #75865, #6701, #22047, #75320, #9211, #79948, #26468 ) ) ;
#33122=CARTESIAN_POINT ( 'NONE',  ( -0.03443470937339728616, 1.062992125984252079, -1.635441089090149402 ) ) ;
#33124=CARTESIAN_POINT ( 'NONE',  ( -0.03443470937343537375, 1.064243487142137568, -1.440673310089392478 ) ) ;
#33131=ORIENTED_EDGE ( 'NONE', *, *, #57575, .F. ) ;
#33137=CARTESIAN_POINT ( 'NONE',  ( 0.5314960629920917334, 2.755905511811024056, 3.264097702071378393 ) ) ;
#33148=CARTESIAN_POINT ( 'NONE',  ( -1.076935383196057527, 2.559055118110236560, 0.3149606299212596716 ) ) ;
#33161=VECTOR ( 'NONE', #36122, 39.37007874015748143 ) ;
#33166=LINE ( 'NONE', #6646, #73406 ) ;
#33172=DIRECTION ( 'NONE',  ( -0.000000000000000000, -1.000000000000000000, -0.000000000000000000 ) ) ;
#33182=EDGE_CURVE ( 'NONE', #5038, #51414, #33851, .T. ) ;
#33187=VERTEX_POINT ( 'NONE', #71740 ) ;
#33188=EDGE_CURVE ( 'NONE', #45259, #9709, #52628, .T. ) ;
#33189=CARTESIAN_POINT ( 'NONE',  ( 0.4697243008124812880, 1.606021484273581823, -2.565507813389724223 ) ) ;
#33198=CARTESIAN_POINT ( 'NONE',  ( 0.4441561269002810564, 1.369975275916394342, -3.911878359814730644 ) ) ;
#33199=CIRCLE ( 'NONE', #30550, 0.09842519685039351207 ) ;
#33201=CONICAL_SURFACE ( 'NONE', #25119, 2.637795275590551380, 0.7853981633974500554 ) ;
#33207=ORIENTED_EDGE ( 'NONE', *, *, #72797, .F. ) ;
#33223=ORIENTED_EDGE ( 'NONE', *, *, #28501, .T. ) ;
#33226=CARTESIAN_POINT ( 'NONE',  ( 2.571257611060531190, 1.453715418023198591, 0.4672341690643353473 ) ) ;
#33231=EDGE_CURVE ( 'NONE', #63414, #37754, #44558, .T. ) ;
#33257=CARTESIAN_POINT ( 'NONE',  ( -2.611722799339339485, 1.697109554835841472, -0.4469779880792068005 ) ) ;
#33260=CARTESIAN_POINT ( 'NONE',  ( 3.900966923095589678, 2.677165354330708791, 0.5314960629921260393 ) ) ;
#33266=AXIS2_PLACEMENT_3D ( 'NONE', #30048, #75101, #42259 ) ;
#33267=CIRCLE ( 'NONE', #80325, 0.1978346456692914035 ) ;
#33269=CARTESIAN_POINT ( 'NONE',  ( 3.937007874015748143, 1.537401574803149984, 2.901595197523589142E-16 ) ) ;
#33277=LINE ( 'NONE', #51344, #38061 ) ;
#33318=DIRECTION ( 'NONE',  ( -0.000000000000000000, -1.000000000000000000, -0.000000000000000000 ) ) ;
#33327=VERTEX_POINT ( 'NONE', #54864 ) ;
#33331=CONICAL_SURFACE ( 'NONE', #83055, 0.1978346456692914035, 0.8726646259971700959 ) ;
#33345=DIRECTION ( 'NONE',  ( 3.491481338843132961E-15, 0.000000000000000000, -1.000000000000000000 ) ) ;
#33346=VERTEX_POINT ( 'NONE', #67506 ) ;
#33355=LINE ( 'NONE', #33765, #20343 ) ;
#33369=CARTESIAN_POINT ( 'NONE',  ( -0.6299212598425059095, 2.165354330708661568, -3.937007874015764131 ) ) ;
#33379=DIRECTION ( 'NONE',  ( -0.000000000000000000, -1.000000000000000000, -0.000000000000000000 ) ) ;
#33381=CIRCLE ( 'NONE', #73714, 1.178877988035069047 ) ;
#33389=ADVANCED_FACE ( 'NONE', ( #80569 ), #74172, .F. ) ;
#33390=FACE_OUTER_BOUND ( 'NONE', #41093, .T. ) ;
#33416=CARTESIAN_POINT ( 'NONE',  ( 0.3250094633868885197, 1.191472453874008020, 1.074005115865686477 ) ) ;
#33438=ORIENTED_EDGE ( 'NONE', *, *, #47097, .F. ) ;
#33442=DIRECTION ( 'NONE',  ( 0.000000000000000000, 0.000000000000000000, 1.000000000000000000 ) ) ;
#33451=CARTESIAN_POINT ( 'NONE',  ( -1.038399629478160113, 1.326389387685770638, -0.4251810372651388392 ) ) ;
#33458=CARTESIAN_POINT ( 'NONE',  ( -0.5314960629921194890, 2.729653112167212736, -1.868118600003770391 ) ) ;
#33473=ADVANCED_FACE ( 'NONE', ( #2702 ), #41413, .F. ) ;
#33484=CYLINDRICAL_SURFACE ( 'NONE', #58187, 0.4744094488188972947 ) ;
#33485=EDGE_CURVE ( 'NONE', #37547, #63414, #54024, .T. ) ;
#33490=ORIENTED_EDGE ( 'NONE', *, *, #48506, .T. ) ;
#33503=DIRECTION ( 'NONE',  ( 0.000000000000000000, -0.7071067811865462405, -0.7071067811865486830 ) ) ;
#33513=CARTESIAN_POINT ( 'NONE',  ( 0.6299212598425337761, 2.755905511811024056, -3.886287458032460229 ) ) ;
#33540=LINE ( 'NONE', #33122, #14688 ) ;
#33542=CARTESIAN_POINT ( 'NONE',  ( 0.4734416007054343400, 1.572145545125848587, 2.167714792466635565 ) ) ;
#33549=VERTEX_POINT ( 'NONE', #48132 ) ;
#33554=CARTESIAN_POINT ( 'NONE',  ( -2.161121219943175742, 1.597527518877485786, 0.4706608522957222984 ) ) ;
#33577=CARTESIAN_POINT ( 'NONE',  ( -0.4485632242333278397, 1.695109487299527817, -1.028575266362750096 ) ) ;
#33600=ORIENTED_EDGE ( 'NONE', *, *, #27842, .F. ) ;
#33601=FACE_OUTER_BOUND ( 'NONE', #18834, .T. ) ;
#33602=EDGE_CURVE ( 'NONE', #38567, #30834, #48611, .T. ) ;
#33608=EDGE_CURVE ( 'NONE', #78998, #41007, #78903, .T. ) ;
#33611=CARTESIAN_POINT ( 'NONE',  ( 0.1229985535008144004, 1.078950944086593200, -3.935114172421038337 ) ) ;
#33612=CARTESIAN_POINT ( 'NONE',  ( 3.826707563893392283, 2.755905511811024500, 0.5314960629921261503 ) ) ;
#33636=CARTESIAN_POINT ( 'NONE',  ( 2.777177547361622256, 1.169463170161816779, 0.3010181502270526388 ) ) ;
#33639=EDGE_CURVE ( 'NONE', #28101, #65196, #80978, .T. ) ;
#33664=CIRCLE ( 'NONE', #59179, 3.937007874015748143 ) ;
#33670=DIRECTION ( 'NONE',  ( 0.000000000000000000, 0.000000000000000000, -1.000000000000000000 ) ) ;
#33697=MANIFOLD_SOLID_BREP ( 'Fillet2', #25857 ) ;
#33701=LINE ( 'NONE', #79583, #31349 ) ;
#33702=ORIENTED_EDGE ( 'NONE', *, *, #18159, .F. ) ;
#33708=CARTESIAN_POINT ( 'NONE',  ( -1.868118687985136805, 2.729653196743539567, 0.5314960629921260393 ) ) ;
#33725=CARTESIAN_POINT ( 'NONE',  ( 0.008867907465126901798, 1.063056921846344371, -1.625415946341134399 ) ) ;
#33728=VECTOR ( 'NONE', #7878, 39.37007874015748143 ) ;
#33750=AXIS2_PLACEMENT_3D ( 'NONE', #35780, #29460, #68195 ) ;
#33752=CARTESIAN_POINT ( 'NONE',  ( -0.5314960629921395840, 2.677165354330708791, 3.900966923095588346 ) ) ;
#33754=CARTESIAN_POINT ( 'NONE',  ( 3.911272252003783034, 1.384743710585661924, -0.4494451973059669370 ) ) ;
#33765=CARTESIAN_POINT ( 'NONE',  ( 3.924389226575468737, 2.755905511811024056, -0.3149606299212597271 ) ) ;
#33780=CARTESIAN_POINT ( 'NONE',  ( 0.000000000000000000, 2.755905511811024056, 0.000000000000000000 ) ) ;
#33788=VECTOR ( 'NONE', #69414, 39.37007874015748143 ) ;
#33800=CARTESIAN_POINT ( 'NONE',  ( -0.03443470937339819515, 1.064243487142144673, -1.633358474390059989 ) ) ;
#33807=DIRECTION ( 'NONE',  ( -3.491481338843133355E-15, -0.000000000000000000, 1.000000000000000000 ) ) ;
#33817=CARTESIAN_POINT ( 'NONE',  ( -3.184294706754630777, 2.755905511811024056, -0.5314960629921260393 ) ) ;
#33840=AXIS2_PLACEMENT_3D ( 'NONE', #37266, #24625, #75170 ) ;
#33849=CARTESIAN_POINT ( 'NONE',  ( -0.3149606299212458493, 2.165354330708661568, -3.937007874015763242 ) ) ;
#33851=LINE ( 'NONE', #46047, #12331 ) ;
#33853=EDGE_CURVE ( 'NONE', #57422, #75161, #192, .T. ) ;
#33884=CARTESIAN_POINT ( 'NONE',  ( 2.543486866223389153, 2.716535433070866645, 0.5314960629921260393 ) ) ;
#33900=CONICAL_SURFACE ( 'NONE', #59433, 2.559055118110236560, 0.7853981633974500554 ) ;
#33915=DIRECTION ( 'NONE',  ( -1.000000000000000000, -0.000000000000000000, -0.000000000000000000 ) ) ;
#33945=VERTEX_POINT ( 'NONE', #23290 ) ;
#33955=AXIS2_PLACEMENT_3D ( 'NONE', #30545, #19144, #30948 ) ;
#33956=EDGE_CURVE ( 'NONE', #39102, #11296, #79151, .T. ) ;
#33968=CARTESIAN_POINT ( 'NONE',  ( 0.000000000000000000, 0.03937007874015747977, -3.405511811023621771 ) ) ;
#33970=CARTESIAN_POINT ( 'NONE',  ( 2.000606668791046427, 1.230840736494993815, -0.3632157284009380760 ) ) ;
#33977=CARTESIAN_POINT ( 'NONE',  ( -0.5314960629921373636, 2.729657682812315134, 3.237502084714954709 ) ) ;
#33993=CARTESIAN_POINT ( 'NONE',  ( 0.4478265126066724999, 1.380810887145295096, -1.530100757606696060 ) ) ;
#33999=PLANE ( 'NONE',  #7611 ) ;
#34002=CONICAL_SURFACE ( 'NONE', #71673, 3.307086614173228689, 0.7853981633974500554 ) ;
#34010=DIRECTION ( 'NONE',  ( -0.000000000000000000, -1.000000000000000000, -0.000000000000000000 ) ) ;
#34015=VECTOR ( 'NONE', #61649, 39.37007874015748854 ) ;
#34018=CARTESIAN_POINT ( 'NONE',  ( -3.841955293929017135, 2.753420937170568461, -0.5314960629921260393 ) ) ;
#34027=CARTESIAN_POINT ( 'NONE',  ( 3.900966923095589678, 2.687614851728675092, 0.5314960629921259283 ) ) ;
#34044=VERTEX_POINT ( 'NONE', #71647 ) ;
#34046=ORIENTED_EDGE ( 'NONE', *, *, #59684, .F. ) ;
#34049=CARTESIAN_POINT ( 'NONE',  ( -1.467262695449858212, 1.144328835045041570, 0.2657261524766077465 ) ) ;
#34055=DIRECTION ( 'NONE',  ( 0.000000000000000000, 1.000000000000000000, 8.673617379884024625E-16 ) ) ;
#34061=ORIENTED_EDGE ( 'NONE', *, *, #20875, .F. ) ;
#34077=AXIS2_PLACEMENT_3D ( 'NONE', #46441, #72131, #8993 ) ;
#34082=EDGE_CURVE ( 'NONE', #29058, #22351, #26941, .T. ) ;
#34090=CARTESIAN_POINT ( 'NONE',  ( -1.850381573804679824, 1.062979042929935281, 0.007789085821720239007 ) ) ;
#34103=EDGE_CURVE ( 'NONE', #21631, #23049, #64914, .T. ) ;
#34111=DIRECTION ( 'NONE',  ( -0.000000000000000000, 1.000000000000000000, -0.000000000000000000 ) ) ;
#34119=AXIS2_PLACEMENT_3D ( 'NONE', #82038, #24352, #50842 ) ;
#34124=DIRECTION ( 'NONE',  ( -0.000000000000000000, 1.000000000000000000, -0.000000000000000000 ) ) ;
#34125=FACE_OUTER_BOUND ( 'NONE', #10458, .T. ) ;
#34129=DIRECTION ( 'NONE',  ( 0.000000000000000000, 1.000000000000000000, -8.673617379884024625E-16 ) ) ;
#34134=AXIS2_PLACEMENT_3D ( 'NONE', #47155, #61037, #61452 ) ;
#34151=EDGE_LOOP ( 'NONE', ( #46461, #47788, #69413, #71087 ) ) ;
#34168=CARTESIAN_POINT ( 'NONE',  ( -2.362204724409448620, 0.03937007874015751446, -0.5118110236220719811 ) ) ;
#34171=CARTESIAN_POINT ( 'NONE',  ( 3.937005118394719005, 1.063014994214472431, -0.03171225910627740313 ) ) ;
#34181=AXIS2_PLACEMENT_3D ( 'NONE', #17509, #43141, #24206 ) ;
#34206=CARTESIAN_POINT ( 'NONE',  ( 1.035593395983585907, 1.340617077144278024, -0.4319465832450602449 ) ) ;
#34233=EDGE_LOOP ( 'NONE', ( #73083, #2368, #62949, #56776, #78783, #5722, #57735, #81684, #80032, #56599, #77117, #53494 ) ) ;
#34235=CARTESIAN_POINT ( 'NONE',  ( 3.870235431238101764, 2.740199102106095186, -0.5314960629921260393 ) ) ;
#34245=CARTESIAN_POINT ( 'NONE',  ( 0.4259733500547865370, 1.326302081955849310, 1.038124814314992372 ) ) ;
#34251=VECTOR ( 'NONE', #1047, 39.37007874015748143 ) ;
#34263=ADVANCED_FACE ( 'NONE', ( #53112 ), #79658, .F. ) ;
#34274=EDGE_CURVE ( 'NONE', #66374, #32472, #21150, .T. ) ;
#34278=EDGE_LOOP ( 'NONE', ( #32227, #22264, #54634, #50056 ) ) ;
#34280=CARTESIAN_POINT ( 'NONE',  ( -1.024260578284143186, 1.413296633437248984, -0.4581541405492637331 ) ) ;
#34333=EDGE_CURVE ( 'NONE', #58442, #27207, #33664, .T. ) ;
#34346=ORIENTED_EDGE ( 'NONE', *, *, #3777, .T. ) ;
#34365=ORIENTED_EDGE ( 'NONE', *, *, #3552, .F. ) ;
#34373=CARTESIAN_POINT ( 'NONE',  ( -3.937007874015748143, 1.724409448818898127, -0.6299212598425202314 ) ) ;
#34381=CARTESIAN_POINT ( 'NONE',  ( 0.5314960629921392510, 2.753420937170568461, -3.841955293929014026 ) ) ;
#34387=CARTESIAN_POINT ( 'NONE',  ( -3.937007874015748143, 2.755905511811024056, 0.5314960629921260393 ) ) ;
#34394=CARTESIAN_POINT ( 'NONE',  ( 0.000000000000000000, 2.755905511811024056, 0.000000000000000000 ) ) ;
#34409=VECTOR ( 'NONE', #44301, 39.37007874015748143 ) ;
#34419=CARTESIAN_POINT ( 'NONE',  ( -3.937007874015748143, 1.537401574803149984, -0.4744094488188975722 ) ) ;
#34436=CARTESIAN_POINT ( 'NONE',  ( 1.141392835773559211, 0.3937007874015748254, 1.456353465694822491 ) ) ;
#34449=EDGE_LOOP ( 'NONE', ( #76891, #33207, #69773, #77641 ) ) ;
#34466=ORIENTED_EDGE ( 'NONE', *, *, #81028, .T. ) ;
#34471=CARTESIAN_POINT ( 'NONE',  ( 2.557132292622070757, 1.503024749832830631, 0.4732391302016651369 ) ) ;
#34477=LINE ( 'NONE', #2494, #33161 ) ;
#34482=ORIENTED_EDGE ( 'NONE', *, *, #45967, .T. ) ;
#34492=CONICAL_SURFACE ( 'NONE', #80171, 3.228346456692913424, 0.7853981633974500554 ) ;
#34511=CARTESIAN_POINT ( 'NONE',  ( -2.170146923806554273, 1.537401574803149984, -0.4744094488188975722 ) ) ;
#34519=DIRECTION ( 'NONE',  ( 0.000000000000000000, 0.000000000000000000, 1.000000000000000000 ) ) ;
#34541=PLANE ( 'NONE',  #10383 ) ;
#34546=DIRECTION ( 'NONE',  ( 0.000000000000000000, 0.000000000000000000, 1.000000000000000000 ) ) ;
#34547=DIRECTION ( 'NONE',  ( -3.491481338843132961E-15, -0.000000000000000000, 1.000000000000000000 ) ) ;
#34554=ORIENTED_EDGE ( 'NONE', *, *, #67320, .F. ) ;
#34560=CARTESIAN_POINT ( 'NONE',  ( 0.004535564325209356581, 1.062992125984248748, -1.627527093699462135 ) ) ;
#34570=ORIENTED_EDGE ( 'NONE', *, *, #42480, .F. ) ;
#34573=VERTEX_POINT ( 'NONE', #82124 ) ;
#34591=CARTESIAN_POINT ( 'NONE',  ( 3.918979230920996315, 1.247401896492644102, 0.3767456479477053755 ) ) ;
#34592=EDGE_CURVE ( 'NONE', #43965, #66126, #82757, .T. ) ;
#34593=CIRCLE ( 'NONE', #81638, 0.3149606299212597271 ) ;
#34597=CARTESIAN_POINT ( 'NONE',  ( 3.937007874015748143, 1.724409448818897905, -0.4359958488159719758 ) ) ;
#34603=DIRECTION ( 'NONE',  ( -3.491481338843132961E-15, 0.000000000000000000, 1.000000000000000000 ) ) ;
#34612=DIRECTION ( 'NONE',  ( 0.000000000000000000, 0.000000000000000000, -1.000000000000000000 ) ) ;
#34616=CARTESIAN_POINT ( 'NONE',  ( 0.5314960629920922885, 2.729659900128874828, 3.210901142567245348 ) ) ;
#34617=DIRECTION ( 'NONE',  ( 0.000000000000000000, 0.000000000000000000, -1.000000000000000000 ) ) ;
#34618=B_SPLINE_CURVE_WITH_KNOTS ( 'NONE', 3,
 ( #34667, #45603, #71297, #2678, #1433, #13645, #40143, #78038, #72960, #32989, #65828, #72549 ),
 .UNSPECIFIED., .F., .F.,
 ( 4, 2, 2, 2, 2, 4 ),
 ( 0.04729187226826467999, 0.04795755069747602989, 0.04862322912668737979, 0.04995458598511005877, 0.05128594284353273774, 0.05261729970195541672 ),
 .UNSPECIFIED. ) ;
#34626=DIRECTION ( 'NONE',  ( 0.000000000000000000, -1.000000000000000000, 0.000000000000000000 ) ) ;
#34656=CARTESIAN_POINT ( 'NONE',  ( 0.4102808022082889416, 1.299212598425196985, -1.382164990278189398 ) ) ;
#34659=EDGE_CURVE ( 'NONE', #19542, #16864, #50913, .T. ) ;
#34667=CARTESIAN_POINT ( 'NONE',  ( -0.4744094488188894121, 1.537401574803149984, -2.170146923806595574 ) ) ;
#34686=ADVANCED_FACE ( 'NONE', ( #61926 ), #49698, .F. ) ;
#34692=DIRECTION ( 'NONE',  ( -3.491481338843132961E-15, -0.000000000000000000, 1.000000000000000000 ) ) ;
#34698=ORIENTED_EDGE ( 'NONE', *, *, #40133, .F. ) ;
#34700=CARTESIAN_POINT ( 'NONE',  ( -1.102283499656470322, 1.111697496334393742, 0.2116636225555746376 ) ) ;
#34702=FACE_OUTER_BOUND ( 'NONE', #53871, .T. ) ;
#34725=B_SPLINE_CURVE_WITH_KNOTS ( 'NONE', 3,
 ( #76461, #57486, #67363, #69315, #30993, #11666, #24267, #25087, #61031, #9696, #3381, #62996, #56258, #29043, #80421, #22732, #48391, #82362, #81954, #75638, #50348, #43614, #5335, #46529, #1523, #20037, #1937, #19611, #77281, #59580, #19194, #46113, #20877, #65914, #25921, #78126, #51579, #20460, #45274, #59165 ),
 .UNSPECIFIED., .F., .F.,
 ( 4, 2, 2, 2, 2, 2, 2, 2, 2, 2, 2, 2, 2, 2, 2, 2, 2, 2, 2, 4 ),
 ( 0.000000000000000000, 0.002124304967526596203, 0.003186457451289890618, 0.003717533693171541295, 0.004248609935053191539, 0.005310762418816507638, 0.005841838660698156147, 0.006372914902579806390, 0.006903991144461454899, 0.007435067386343104275, 0.008497219870106381343, 0.009559372353869659278, 0.01009044859575129738, 0.01062152483763293374, 0.01168367732139621168, 0.01221475356327785672, 0.01274582980515950176, 0.01380798228892279184, 0.01487013477268608018, 0.01699443974021267595 ),
 .UNSPECIFIED. ) ;
#34736=DIRECTION ( 'NONE',  ( 1.000000000000000000, 0.000000000000000000, 3.455050906509825972E-15 ) ) ;
#34739=DIRECTION ( 'NONE',  ( -3.491481338843133355E-15, -0.000000000000000000, 1.000000000000000000 ) ) ;
#34741=ORIENTED_EDGE ( 'NONE', *, *, #4418, .F. ) ;
#34742=ADVANCED_FACE ( 'NONE', ( #69068 ), #51863, .T. ) ;
#34753=CYLINDRICAL_SURFACE ( 'NONE', #35899, 0.5118110236220472231 ) ;
#34769=ORIENTED_EDGE ( 'NONE', *, *, #18297, .F. ) ;
#34776=CARTESIAN_POINT ( 'NONE',  ( 0.4177787735907000366, 0.4110443821404751730, -1.559171609364239375 ) ) ;
#34788=ORIENTED_EDGE ( 'NONE', *, *, #51075, .T. ) ;
#34789=CARTESIAN_POINT ( 'NONE',  ( -1.622865925661502562, 1.365114174391409252, 0.4420857170566875327 ) ) ;
#34809=CARTESIAN_POINT ( 'NONE',  ( 1.894990545102974044, 1.111478976311914613, -0.2095522481616541033 ) ) ;
#34816=DIRECTION ( 'NONE',  ( 0.000000000000000000, 0.000000000000000000, -1.000000000000000000 ) ) ;
#34849=DIRECTION ( 'NONE',  ( -0.000000000000000000, -1.000000000000000000, -0.000000000000000000 ) ) ;
#34851=B_SPLINE_CURVE_WITH_KNOTS ( 'NONE', 3,
 ( #60377, #73853, #55291, #48983, #48568, #15784, #42252, #67119, #9450, #35121, #67947, #10289 ),
 .UNSPECIFIED., .F., .F.,
 ( 4, 2, 2, 2, 2, 4 ),
 ( 0.007992874908875390386, 0.009303755029337522353, 0.01061463514979965432, 0.01192551527026178629, 0.01258095533049285661, 0.01323639539072392866 ),
 .UNSPECIFIED. ) ;
#34855=DIRECTION ( 'NONE',  ( -0.000000000000000000, 1.000000000000000000, -0.000000000000000000 ) ) ;
#34865=AXIS2_PLACEMENT_3D ( 'NONE', #19876, #77115, #77541 ) ;
#34866=ORIENTED_EDGE ( 'NONE', *, *, #79768, .F. ) ;
#34868=VERTEX_POINT ( 'NONE', #20527 ) ;
#34887=CARTESIAN_POINT ( 'NONE',  ( 2.593354744918233923, 1.408268389154266220, 0.4567427728026669520 ) ) ;
#34898=ORIENTED_EDGE ( 'NONE', *, *, #13664, .T. ) ;
#34900=CARTESIAN_POINT ( 'NONE',  ( 0.5314960629920996160, 2.742784459617114923, 2.516666435443592142 ) ) ;
#34901=ORIENTED_EDGE ( 'NONE', *, *, #26367, .F. ) ;
#34919=DIRECTION ( 'NONE',  ( 0.000000000000000000, -1.000000000000000000, 1.408710688920637755E-15 ) ) ;
#34922=CARTESIAN_POINT ( 'NONE',  ( 2.362204724409448620, 1.724409448818898127, 0.5118110236220555498 ) ) ;
#34928=CARTESIAN_POINT ( 'NONE',  ( -0.5314960629921126056, 2.753838553078472362, -3.842312626974350831 ) ) ;
#34936=DIRECTION ( 'NONE',  ( 0.000000000000000000, -0.7071067811865496822, -0.7071067811865454633 ) ) ;
#34953=VERTEX_POINT ( 'NONE', #754 ) ;
#34958=DIRECTION ( 'NONE',  ( 0.000000000000000000, 1.000000000000000000, -0.000000000000000000 ) ) ;
#34961=CYLINDRICAL_SURFACE ( 'NONE', #61043, 0.3149606299212598381 ) ;
#34965=ORIENTED_EDGE ( 'NONE', *, *, #13087, .F. ) ;
#34979=CARTESIAN_POINT ( 'NONE',  ( 0.1654368116759125928, 1.092466590690394090, -2.846817106506551287 ) ) ;
#34982=VERTEX_POINT ( 'NONE', #20941 ) ;
#35002=LINE ( 'NONE', #53926, #10659 ) ;
#35013=CARTESIAN_POINT ( 'NONE',  ( 2.362204724409448620, 1.724409448818900570, 8.247593713802677664E-15 ) ) ;
#35020=CARTESIAN_POINT ( 'NONE',  ( -0.4026890765610274814, 1.286118078602604520, -1.047337338654595662 ) ) ;
#35049=DIRECTION ( 'NONE',  ( 0.000000000000000000, -0.5150380749100549327, -0.8571673007021117785 ) ) ;
#35058=ORIENTED_EDGE ( 'NONE', *, *, #82449, .T. ) ;
#35062=EDGE_CURVE ( 'NONE', #3377, #44828, #70682, .T. ) ;
#35063=CARTESIAN_POINT ( 'NONE',  ( 0.4128820156421557641, 1.303693191736402301, -1.389518450040436948 ) ) ;
#35086=CARTESIAN_POINT ( 'NONE',  ( -0.1654213697349098400, 1.092461187568469994, -2.846822072454109787 ) ) ;
#35088=DIRECTION ( 'NONE',  ( 0.000000000000000000, 0.000000000000000000, -1.000000000000000000 ) ) ;
#35091=ORIENTED_EDGE ( 'NONE', *, *, #51971, .T. ) ;
#35095=DIRECTION ( 'NONE',  ( -3.491481338843132961E-15, -0.000000000000000000, 1.000000000000000000 ) ) ;
#35096=CARTESIAN_POINT ( 'NONE',  ( -0.4744094488189107839, 1.569370081724417609, 3.908320185825790993 ) ) ;
#35121=CARTESIAN_POINT ( 'NONE',  ( 2.554860351194764956, 1.554815631980118074, -0.4741686481756392513 ) ) ;
#35125=CIRCLE ( 'NONE', #68706, 0.2165354330708659791 ) ;
#35143=CARTESIAN_POINT ( 'NONE',  ( 0.4177787735907000921, 0.000000000000000000, -1.244210979442979648 ) ) ;
#35148=ORIENTED_EDGE ( 'NONE', *, *, #14394, .F. ) ;
#35177=ORIENTED_EDGE ( 'NONE', *, *, #24957, .F. ) ;
#35186=DIRECTION ( 'NONE',  ( 0.000000000000000000, 1.000000000000000000, 0.000000000000000000 ) ) ;
#35194=ORIENTED_EDGE ( 'NONE', *, *, #32413, .T. ) ;
#35197=CARTESIAN_POINT ( 'NONE',  ( -1.542758472124253988, 1.384765482578574902, 0.4491926697227655585 ) ) ;
#35210=CARTESIAN_POINT ( 'NONE',  ( 0.5314960629921396951, 2.697992270790283698, -3.898836503597931991 ) ) ;
#35211=VERTEX_POINT ( 'NONE', #70936 ) ;
#35213=CARTESIAN_POINT ( 'NONE',  ( 0.000000000000000000, 2.677165354330708791, 0.000000000000000000 ) ) ;
#35238=B_SPLINE_CURVE_WITH_KNOTS ( 'NONE', 3,
 ( #69516, #11865, #18986, #37518 ),
 .UNSPECIFIED., .F., .F.,
 ( 4, 4 ),
 ( 2.857347768987377627E-07, 0.001436604392377181273 ),
 .UNSPECIFIED. ) ;
#35245=LINE ( 'NONE', #3261, #50197 ) ;
#35268=CARTESIAN_POINT ( 'NONE',  ( -3.908420089088291416, 1.569603073218160061, 0.4735885527812596085 ) ) ;
#35290=ORIENTED_EDGE ( 'NONE', *, *, #16168, .T. ) ;
#35295=CARTESIAN_POINT ( 'NONE',  ( 0.000000000000000000, 2.559055118110236560, 0.000000000000000000 ) ) ;
#35301=DIRECTION ( 'NONE',  ( -0.000000000000000000, -1.000000000000000000, -0.000000000000000000 ) ) ;
#35336=CARTESIAN_POINT ( 'NONE',  ( 0.5314960629920852941, 2.729333734409945755, 3.881246834694722203 ) ) ;
#35343=AXIS2_PLACEMENT_3D ( 'NONE', #35213, #29309, #16285 ) ;
#35362=CYLINDRICAL_SURFACE ( 'NONE', #77028, 0.09842519685039351207 ) ;
#35366=CARTESIAN_POINT ( 'NONE',  ( 0.2239781325220697450, 1.118900601684395202, 2.822659112694967831 ) ) ;
#35386=CARTESIAN_POINT ( 'NONE',  ( 0.008982673068357337198, 1.062992125984252523, -1.448165499020492186 ) ) ;
#35391=CARTESIAN_POINT ( 'NONE',  ( 0.2248141966262373892, 1.118402650174323609, -2.823092204040328568 ) ) ;
#35394=ORIENTED_EDGE ( 'NONE', *, *, #19351, .T. ) ;
#35403=CIRCLE ( 'NONE', #36700, 0.5118110236220471121 ) ;
#35455=CIRCLE ( 'NONE', #36765, 1.122047244094488194 ) ;
#35461=ADVANCED_FACE ( 'NONE', ( #45652 ), #46904, .F. ) ;
#35462=CARTESIAN_POINT ( 'NONE',  ( 2.543486866223389153, 2.716535433070866645, 0.5314960629921260393 ) ) ;
#35471=ORIENTED_EDGE ( 'NONE', *, *, #60504, .T. ) ;
#35486=DIRECTION ( 'NONE',  ( 0.000000000000000000, 0.000000000000000000, -1.000000000000000000 ) ) ;
#35503=CARTESIAN_POINT ( 'NONE',  ( 0.000000000000000000, 2.755905511811024056, 0.000000000000000000 ) ) ;
#35506=EDGE_LOOP ( 'NONE', ( #1159, #17208, #26998, #68946 ) ) ;
#35510=CARTESIAN_POINT ( 'NONE',  ( 1.348312163386739426, 0.2755905511811023723, 0.6402614161801758463 ) ) ;
#35521=ORIENTED_EDGE ( 'NONE', *, *, #21285, .F. ) ;
#35556=CARTESIAN_POINT ( 'NONE',  ( -0.03443470937339728616, 0.2755905511811023723, -1.537015892239756099 ) ) ;
#35577=CARTESIAN_POINT ( 'NONE',  ( -2.530077735013332330, 2.729661055914112566, 0.5314960629921260393 ) ) ;
#35597=LINE ( 'NONE', #9513, #63507 ) ;
#35600=ADVANCED_FACE ( 'NONE', ( #29221, #41023 ), #36360, .T. ) ;
#35606=ORIENTED_EDGE ( 'NONE', *, *, #77795, .T. ) ;
#35612=DIRECTION ( 'NONE',  ( -3.491481338843132961E-15, -0.000000000000000000, 1.000000000000000000 ) ) ;
#35613=CARTESIAN_POINT ( 'NONE',  ( -1.813482582612293559, 2.755905511811024056, -0.5314960629921260393 ) ) ;
#35629=CARTESIAN_POINT ( 'NONE',  ( 0.4177787735907000366, 1.299212598425196985, -1.559171609364239375 ) ) ;
#35630=EDGE_CURVE ( 'NONE', #44018, #23879, #45126, .T. ) ;
#35639=TOROIDAL_SURFACE ( 'NONE', #80001, 3.858267716535433323, 0.07874015748031495954 ) ;
#35657=CARTESIAN_POINT ( 'NONE',  ( 0.000000000000000000, 2.755905511811024056, 0.000000000000000000 ) ) ;
#35683=AXIS2_PLACEMENT_3D ( 'NONE', #37088, #63587, #12253 ) ;
#35685=ORIENTED_EDGE ( 'NONE', *, *, #76828, .T. ) ;
#35701=VERTEX_POINT ( 'NONE', #80593 ) ;
#35710=CARTESIAN_POINT ( 'NONE',  ( 0.6299212598425338872, 2.165354330708662012, -3.886287458032460229 ) ) ;
#35718=ORIENTED_EDGE ( 'NONE', *, *, #36840, .T. ) ;
#35732=EDGE_CURVE ( 'NONE', #44828, #72873, #34851, .T. ) ;
#35745=VECTOR ( 'NONE', #40490, 39.37007874015748143 ) ;
#35746=CARTESIAN_POINT ( 'NONE',  ( -1.857294464233399278, 1.070443199938749590, -0.08545185031209458215 ) ) ;
#35750=EDGE_CURVE ( 'NONE', #57500, #67621, #74731, .T. ) ;
#35767=CARTESIAN_POINT ( 'NONE',  ( -1.313877454013331780, 0.2755905511811023723, 0.7983292792091805090 ) ) ;
#35773=CARTESIAN_POINT ( 'NONE',  ( -3.237502121466738103, 2.729657719074700672, 0.5314960629921260393 ) ) ;
#35777=EDGE_CURVE ( 'NONE', #60543, #82716, #76108, .T. ) ;
#35780=CARTESIAN_POINT ( 'NONE',  ( 0.000000000000000000, 2.755905511811024056, 0.000000000000000000 ) ) ;
#35784=CIRCLE ( 'NONE', #16996, 0.5118110236220472231 ) ;
#35786=AXIS2_PLACEMENT_3D ( 'NONE', #23207, #56009, #17336 ) ;
#35789=ORIENTED_EDGE ( 'NONE', *, *, #27285, .T. ) ;
#35790=EDGE_CURVE ( 'NONE', #4444, #29055, #57201, .T. ) ;
#35804=FACE_OUTER_BOUND ( 'NONE', #32896, .T. ) ;
#35809=ORIENTED_EDGE ( 'NONE', *, *, #42337, .F. ) ;
#35812=ORIENTED_EDGE ( 'NONE', *, *, #48506, .F. ) ;
#35814=AXIS2_PLACEMENT_3D ( 'NONE', #83133, #57850, #38508 ) ;
#35847=CARTESIAN_POINT ( 'NONE',  ( -0.1539732359166575415, 1.088403462004246425, -1.111533894513872633 ) ) ;
#35855=CONICAL_SURFACE ( 'NONE', #884, 1.889763779527559251, 0.7853981633974500554 ) ;
#35856=AXIS2_PLACEMENT_3D ( 'NONE', #66761, #65514, #8674 ) ;
#35860=EDGE_CURVE ( 'NONE', #7002, #39742, #55898, .T. ) ;
#35882=DIRECTION ( 'NONE',  ( 0.000000000000000000, 0.000000000000000000, -1.000000000000000000 ) ) ;
#35895=CARTESIAN_POINT ( 'NONE',  ( -0.5314960629921393620, 2.755905511811024056, 3.821484228344191880 ) ) ;
#35899=AXIS2_PLACEMENT_3D ( 'NONE', #18181, #9901, #56045 ) ;
#35908=CARTESIAN_POINT ( 'NONE',  ( 0.4102808022082901629, 1.299212598425196985, -1.736178228450289573 ) ) ;
#35930=CARTESIAN_POINT ( 'NONE',  ( -1.019850064477911600, 1.617462848879257731, 0.4678763946775361671 ) ) ;
#35941=CARTESIAN_POINT ( 'NONE',  ( -1.018296575816956206, 1.474731146291503148, 0.4712826680561278958 ) ) ;
#35948=DIRECTION ( 'NONE',  ( -0.000000000000000000, 1.000000000000000000, -0.000000000000000000 ) ) ;
#35956=DIRECTION ( 'NONE',  ( 0.000000000000000000, -1.000000000000000000, -0.000000000000000000 ) ) ;
#35976=CARTESIAN_POINT ( 'NONE',  ( 0.4741693035498537601, 1.520070061304626075, 2.169550896612808977 ) ) ;
#35981=EDGE_LOOP ( 'NONE', ( #69849, #66962, #24923 ) ) ;
#36006=ORIENTED_EDGE ( 'NONE', *, *, #49134, .T. ) ;
#36021=VERTEX_POINT ( 'NONE', #19062 ) ;
#36023=VERTEX_POINT ( 'NONE', #12763 ) ;
#36027=DIRECTION ( 'NONE',  ( -0.8660254037844432595, 0.000000000000000000, 0.4999999999999918954 ) ) ;
#36043=EDGE_CURVE ( 'NONE', #37754, #60631, #17440, .T. ) ;
#36044=CARTESIAN_POINT ( 'NONE',  ( 0.3149606299212736049, 2.755905511811024056, -3.924389226575467404 ) ) ;
#36069=CARTESIAN_POINT ( 'NONE',  ( 3.210901142567240907, 2.729659900128873495, -0.5314960629921260393 ) ) ;
#36072=ORIENTED_EDGE ( 'NONE', *, *, #8432, .F. ) ;
#36122=DIRECTION ( 'NONE',  ( -0.000000000000000000, -1.000000000000000000, -0.000000000000000000 ) ) ;
#36130=ORIENTED_EDGE ( 'NONE', *, *, #67725, .F. ) ;
#36132=DIRECTION ( 'NONE',  ( 0.000000000000000000, 0.000000000000000000, 1.000000000000000000 ) ) ;
#36136=CARTESIAN_POINT ( 'NONE',  ( -0.03101036932649587838, 1.063748226153006682, 3.936916540055557245 ) ) ;
#36166=ADVANCED_FACE ( 'NONE', ( #6019 ), #83045, .F. ) ;
#36169=EDGE_CURVE ( 'NONE', #11296, #29058, #58606, .T. ) ;
#36175=DIRECTION ( 'NONE',  ( 0.000000000000000000, -1.000000000000000000, 0.000000000000000000 ) ) ;
#36188=CARTESIAN_POINT ( 'NONE',  ( 1.141392835773559211, 0.000000000000000000, 1.141392835773562764 ) ) ;
#36192=DIRECTION ( 'NONE',  ( 0.000000000000000000, 0.000000000000000000, -1.000000000000000000 ) ) ;
#36194=ADVANCED_FACE ( 'NONE', ( #24949 ), #3526, .T. ) ;
#36212=DIRECTION ( 'NONE',  ( 0.000000000000000000, 0.000000000000000000, -1.000000000000000000 ) ) ;
#36242=EDGE_CURVE ( 'NONE', #40260, #2780, #63265, .T. ) ;
#36246=DIRECTION ( 'NONE',  ( 0.000000000000000000, -1.000000000000000000, 0.000000000000000000 ) ) ;
#36253=CARTESIAN_POINT ( 'NONE',  ( -2.874027875014218747, 1.062979042929934392, -0.007789085821668992674 ) ) ;
#36256=CARTESIAN_POINT ( 'NONE',  ( -0.06095229741894689357, 1.066899628778971376, -1.625198944407316270 ) ) ;
#36257=ADVANCED_FACE ( 'NONE', ( #64102 ), #38413, .F. ) ;
#36270=LINE ( 'NONE', #79256, #32974 ) ;
#36274=CARTESIAN_POINT ( 'NONE',  ( -0.5314960629921171575, 2.716535433070866645, -2.543486866223390930 ) ) ;
#36285=CARTESIAN_POINT ( 'NONE',  ( -0.6299212598425062426, 2.165354330708661568, -3.886287458032464226 ) ) ;
#36308=CARTESIAN_POINT ( 'NONE',  ( 0.4573592755602257087, 1.664450716761304516, 3.910355061080106331 ) ) ;
#36309=FACE_OUTER_BOUND ( 'NONE', #45821, .T. ) ;
#36314=EDGE_CURVE ( 'NONE', #27310, #6933, #24551, .T. ) ;
#36333=FACE_OUTER_BOUND ( 'NONE', #14776, .T. ) ;
#36334=CARTESIAN_POINT ( 'NONE',  ( -3.937007874015748143, 1.724409448818897905, 0.6299212598425196763 ) ) ;
#36337=( CONVERSION_BASED_UNIT ( 'INCH', #75070 ) LENGTH_UNIT ( ) NAMED_UNIT ( #69059 ) );
#36349=CARTESIAN_POINT ( 'NONE',  ( -2.362204724409448620, 0.03937007874015751446, -2.474278114140802984E-14 ) ) ;
#36352=CARTESIAN_POINT ( 'NONE',  ( 0.000000000000000000, 0.000000000000000000, 0.000000000000000000 ) ) ;
#36360=PLANE ( 'NONE',  #59931 ) ;
#36382=FACE_OUTER_BOUND ( 'NONE', #76505, .T. ) ;
#36409=LINE ( 'NONE', #48208, #70741 ) ;
#36410=B_SPLINE_CURVE_WITH_KNOTS ( 'NONE', 3,
 ( #41509, #40261, #21321, #53702, #2800, #67194, #60448, #35197, #79001, #60858, #79411, #3212, #15017, #47393, #9117, #34789, #28874, #54536, #80252, #48229 ),
 .UNSPECIFIED., .F., .F.,
 ( 4, 2, 2, 2, 2, 2, 2, 2, 2, 4 ),
 ( 0.0005422360305776513902, 0.003127735116393569673, 0.004420484659301528868, 0.005066859430755498925, 0.005713234202209468982, 0.006036421587936466153, 0.006359608973663460722, 0.007005983745117451596, 0.008298733288025460231, 0.01088423237384148617 ),
 .UNSPECIFIED. ) ;
#36449=CARTESIAN_POINT ( 'NONE',  ( 2.138259192565330924, 1.653403552777526153, 0.4602852883866581646 ) ) ;
#36478=VERTEX_POINT ( 'NONE', #13599 ) ;
#36503=VERTEX_POINT ( 'NONE', #21158 ) ;
#36506=ADVANCED_FACE ( 'NONE', ( #77575 ), #78832, .F. ) ;
#36520=ORIENTED_EDGE ( 'NONE', *, *, #4112, .F. ) ;
#36526=B_SPLINE_CURVE_WITH_KNOTS ( 'NONE', 3,
 ( #34511, #60176, #15996, #73227, #15578, #67748, #40405, #41643, #2529, #59753, #28187, #67334, #2940, #41236, #27773, #42052, #28604, #54261, #79977, #61000, #3348, #72402, #29014, #80391, #22703, #35746, #3763, #80794, #8422, #34090, #23111, #29427, #79145, #36979, #24344, #31483, #42460, #61830, #69389, #31068, #62660, #69797, #23521, #23936, #37801, #29834, #49191, #74892, #17240, #81206, #11321, #42868, #74476, #57144, #50013, #37398, #55497, #68562, #56737, #5000 ),
 .UNSPECIFIED., .F., .F.,
 ( 4, 2, 2, 2, 2, 2, 2, 2, 2, 2, 2, 2, 2, 2, 2, 2, 2, 2, 2, 2, 2, 2, 2, 2, 2, 2, 2, 2, 2, 4 ),
 ( 0.01323639539072319141, 0.01388181161316683759, 0.01452722783561048205, 0.01581806028049779350, 0.01710889272538510322, 0.01839972517027241294, 0.02098139006004704626, 0.02356305494982167958, 0.02485388739470899278, 0.02614471983959630944, 0.02743555228448362263, 0.02872638472937093929, 0.03130804961914556567, 0.03259888206403287886, 0.03388971450892019205, 0.03453513073136384171, 0.03518054695380749830, 0.03647137939869481843, 0.03776221184358213162, 0.03905304428846944481, 0.04034387673335675800, 0.04163470917824407813, 0.04421637406801870451, 0.04679803895779334477, 0.04937970384756797115, 0.05067053629245528434, 0.05196136873734259753, 0.05325220118222991073, 0.05389761740467358120, 0.05454303362711723779 ),
 .UNSPECIFIED. ) ;
#36537=FACE_OUTER_BOUND ( 'NONE', #81560, .T. ) ;
#36538=ORIENTED_EDGE ( 'NONE', *, *, #59829, .F. ) ;
#36566=DIRECTION ( 'NONE',  ( -1.000000000000000000, -0.000000000000000000, -0.000000000000000000 ) ) ;
#36579=CARTESIAN_POINT ( 'NONE',  ( -3.933480768563217378, 1.093172257416577864, -0.1672395799304293440 ) ) ;
#36585=ORIENTED_EDGE ( 'NONE', *, *, #38333, .F. ) ;
#36587=AXIS2_PLACEMENT_3D ( 'NONE', #9381, #47667, #35882 ) ;
#36591=DIRECTION ( 'NONE',  ( -0.000000000000000000, -1.000000000000000000, -0.000000000000000000 ) ) ;
#36594=LINE ( 'NONE', #43307, #74518 ) ;
#36598=ORIENTED_EDGE ( 'NONE', *, *, #57736, .F. ) ;
#36611=DIRECTION ( 'NONE',  ( 0.000000000000000000, -1.000000000000000000, -0.000000000000000000 ) ) ;
#36612=CARTESIAN_POINT ( 'NONE',  ( -1.559171609364246924, 0.3937007874015748254, 0.7327394035119333404 ) ) ;
#36655=CARTESIAN_POINT ( 'NONE',  ( -2.808244076867886019, 1.134815007188475722, 0.2514610820057449070 ) ) ;
#36661=EDGE_CURVE ( 'NONE', #19658, #23658, #62441, .T. ) ;
#36690=CARTESIAN_POINT ( 'NONE',  ( 0.9881811337016640495, 0.000000000000000000, 0.5314960629921260393 ) ) ;
#36700=AXIS2_PLACEMENT_3D ( 'NONE', #18576, #45886, #39593 ) ;
#36715=DIRECTION ( 'NONE',  ( 1.000000000000000000, -0.000000000000000000, 1.224646799147353207E-16 ) ) ;
#36732=DIRECTION ( 'NONE',  ( 8.881784197001252323E-16, 1.460819769243627131E-15, -1.000000000000000000 ) ) ;
#36739=CARTESIAN_POINT ( 'NONE',  ( -1.022773273020813667, 1.648670715164695544, 0.4614513048051138155 ) ) ;
#36740=LINE ( 'NONE', #37979, #59948 ) ;
#36765=AXIS2_PLACEMENT_3D ( 'NONE', #19428, #81775, #76275 ) ;
#36768=DIRECTION ( 'NONE',  ( -3.491481338843132961E-15, -0.000000000000000000, 1.000000000000000000 ) ) ;
#36776=CARTESIAN_POINT ( 'NONE',  ( 1.122040030454554138, 1.063009187292368596, 0.03164884633124447760 ) ) ;
#36790=CARTESIAN_POINT ( 'NONE',  ( 0.4426149705447037230, 1.366040861858875077, 2.104991000353118480 ) ) ;
#36800=DIRECTION ( 'NONE',  ( -0.000000000000000000, -1.000000000000000000, -0.000000000000000000 ) ) ;
#36808=CARTESIAN_POINT ( 'NONE',  ( -0.4497483405553294178, 1.383294989906824313, 1.028048643305481846 ) ) ;
#36809=FACE_OUTER_BOUND ( 'NONE', #55318, .T. ) ;
#36810=AXIS2_PLACEMENT_3D ( 'NONE', #26972, #34129, #71597 ) ;
#36826=CIRCLE ( 'NONE', #82550, 0.5118110236220471121 ) ;
#36840=EDGE_CURVE ( 'NONE', #42095, #50308, #67999, .T. ) ;
#36842=VERTEX_POINT ( 'NONE', #78076 ) ;
#36848=CARTESIAN_POINT ( 'NONE',  ( 0.4177787735907000366, 1.299212598425196985, -1.559171609364239375 ) ) ;
#36850=CARTESIAN_POINT ( 'NONE',  ( -0.5314960629921146040, 2.742781086379890265, -3.250800424960315294 ) ) ;
#36863=CARTESIAN_POINT ( 'NONE',  ( 2.170146923806595129, 1.537401574803149984, 0.4744094488188975722 ) ) ;
#36867=CARTESIAN_POINT ( 'NONE',  ( 0.5314960629921062774, 2.742776604255995565, 1.881759016064410428 ) ) ;
#36869=DIRECTION ( 'NONE',  ( 1.000000000000000000, -0.000000000000000000, -0.000000000000000000 ) ) ;
#36894=VERTEX_POINT ( 'NONE', #26291 ) ;
#36906=CARTESIAN_POINT ( 'NONE',  ( 0.4725409811166971785, 1.494519345219279094, 2.558828502325778853 ) ) ;
#36944=AXIS2_PLACEMENT_3D ( 'NONE', #57012, #43146, #31346 ) ;
#36952=ORIENTED_EDGE ( 'NONE', *, *, #23423, .F. ) ;
#36954=DIRECTION ( 'NONE',  ( -0.000000000000000000, -1.000000000000000000, -0.000000000000000000 ) ) ;
#36955=ORIENTED_EDGE ( 'NONE', *, *, #67735, .F. ) ;
#36979=CARTESIAN_POINT ( 'NONE',  ( -1.854617417371079657, 1.067551433859871723, 0.06782095098400266198 ) ) ;
#36983=EDGE_CURVE ( 'NONE', #80344, #24500, #64004, .T. ) ;
#36999=CARTESIAN_POINT ( 'NONE',  ( -3.935204781620320169, 1.078156475484197685, 0.1229597680020024647 ) ) ;
#37004=FACE_OUTER_BOUND ( 'NONE', #60560, .T. ) ;
#37005=ORIENTED_EDGE ( 'NONE', *, *, #44178, .T. ) ;
#37014=PLANE ( 'NONE',  #63790 ) ;
#37021=ORIENTED_EDGE ( 'NONE', *, *, #42894, .F. ) ;
#37027=DIRECTION ( 'NONE',  ( -0.000000000000000000, -1.000000000000000000, -0.000000000000000000 ) ) ;
#37031=CARTESIAN_POINT ( 'NONE',  ( 0.4744094488189065095, 1.520194873416442549, -2.554262525012259477 ) ) ;
#37034=ORIENTED_EDGE ( 'NONE', *, *, #82019, .T. ) ;
#37070=CARTESIAN_POINT ( 'NONE',  ( -2.585342365690450617, 1.422987107291903364, -0.4606739315415587233 ) ) ;
#37088=CARTESIAN_POINT ( 'NONE',  ( 1.403614904275686858E-14, 1.537401574803149984, -3.937007874015761910 ) ) ;
#37092=AXIS2_PLACEMENT_3D ( 'NONE', #43894, #75092, #69591 ) ;
#37094=CARTESIAN_POINT ( 'NONE',  ( -0.01548461523783284562, 1.062992125984253411, -3.937007874015749476 ) ) ;
#37107=CARTESIAN_POINT ( 'NONE',  ( 0.000000000000000000, 0.000000000000000000, 0.000000000000000000 ) ) ;
#37108=CARTESIAN_POINT ( 'NONE',  ( -0.03443470937339728616, 1.062992125984252079, -1.537015892239756099 ) ) ;
#37112=VECTOR ( 'NONE', #20406, 39.37007874015748143 ) ;
#37132=CARTESIAN_POINT ( 'NONE',  ( -0.1341302950245069070, 1.082049466318360631, -1.868010872266428590 ) ) ;
#37133=VERTEX_POINT ( 'NONE', #71752 ) ;
#37152=ORIENTED_EDGE ( 'NONE', *, *, #31362, .T. ) ;
#37156=AXIS2_PLACEMENT_3D ( 'NONE', #25081, #18385, #13729 ) ;
#37158=CARTESIAN_POINT ( 'NONE',  ( 0.5314960629921068325, 2.742788234388598756, 1.827151616986595339 ) ) ;
#37162=SURFACE_STYLE_FILL_AREA ( #23703 ) ;
#37178=PLANE ( 'NONE',  #43861 ) ;
#37182=CARTESIAN_POINT ( 'NONE',  ( -0.5314960629921124946, 2.712196231959916215, -3.892860353355075631 ) ) ;
#37192=CARTESIAN_POINT ( 'NONE',  ( 1.119419862066250548, 1.069231759244661628, -0.07826300840915889623 ) ) ;
#37198=CARTESIAN_POINT ( 'NONE',  ( 0.9285414500055709786, 2.165354330708661568, -0.6299212598425196763 ) ) ;
#37207=EDGE_CURVE ( 'NONE', #23894, #42095, #46891, .T. ) ;
#37210=CIRCLE ( 'NONE', #47961, 0.5118110236220471121 ) ;
#37212=EDGE_CURVE ( 'NONE', #39102, #68390, #2211, .T. ) ;
#37219=CIRCLE ( 'NONE', #81578, 3.937007874015748143 ) ;
#37265=DIRECTION ( 'NONE',  ( -0.000000000000000000, -1.000000000000000000, -0.000000000000000000 ) ) ;
#37266=CARTESIAN_POINT ( 'NONE',  ( -0.6299212598425059095, 2.165354330708661568, -3.937007874015764131 ) ) ;
#37324=CARTESIAN_POINT ( 'NONE',  ( 0.3003296953575904649, 1.169860122871911434, 2.776875277198005421 ) ) ;
#37334=AXIS2_PLACEMENT_3D ( 'NONE', #30364, #21993, #47654 ) ;
#37335=DIRECTION ( 'NONE',  ( -1.776356839400250465E-15, 0.000000000000000000, -1.000000000000000000 ) ) ;
#37337=VERTEX_POINT ( 'NONE', #51952 ) ;
#37359=LINE ( 'NONE', #31031, #14927 ) ;
#37360=EDGE_CURVE ( 'NONE', #51592, #82476, #71335, .T. ) ;
#37367=ADVANCED_FACE ( 'NONE', ( #15349 ), #67935, .F. ) ;
#37375=FACE_OUTER_BOUND ( 'NONE', #9706, .T. ) ;
#37397=VECTOR ( 'NONE', #33915, 39.37007874015748143 ) ;
#37398=CARTESIAN_POINT ( 'NONE',  ( -2.165607527688992562, 1.494646310179102544, 0.4725519687354810539 ) ) ;
#37416=CARTESIAN_POINT ( 'NONE',  ( -3.908691076466078496, 1.475530872617185185, 0.4713832733224261329 ) ) ;
#37422=FACE_BOUND ( 'NONE', #57420, .T. ) ;
#37427=DIRECTION ( 'NONE',  ( -1.000000000000000000, -0.000000000000000000, -0.000000000000000000 ) ) ;
#37430=LINE ( 'NONE', #55944, #27512 ) ;
#37442=CARTESIAN_POINT ( 'NONE',  ( 0.4177787735907000366, 0.3937007874015748254, -1.559171609364239375 ) ) ;
#37446=CARTESIAN_POINT ( 'NONE',  ( 0.4672625608940805253, 1.453874696264120026, -2.571193713084665600 ) ) ;
#37449=ORIENTED_EDGE ( 'NONE', *, *, #36169, .F. ) ;
#37480=CARTESIAN_POINT ( 'NONE',  ( -3.886287458032462006, 1.724409448818898127, -0.6299212598425202314 ) ) ;
#37485=CARTESIAN_POINT ( 'NONE',  ( -2.759994995438131316, 1.188885443925050245, -0.3231744412229767272 ) ) ;
#37491=DIRECTION ( 'NONE',  ( 0.000000000000000000, 0.000000000000000000, 1.000000000000000000 ) ) ;
#37500=CARTESIAN_POINT ( 'NONE',  ( 0.3811349131313429006, 1.253490138500162443, -2.019723589772945527 ) ) ;
#37505=CARTESIAN_POINT ( 'NONE',  ( 5.818687728935708833E-24, 1.062992125984252745, -3.937007874015748143 ) ) ;
#37518=CARTESIAN_POINT ( 'NONE',  ( -2.118110236220477116, 0.000000000000000000, 0.4498537592782676509 ) ) ;
#37520=FACE_OUTER_BOUND ( 'NONE', #34233, .T. ) ;
#37526=ORIENTED_EDGE ( 'NONE', *, *, #19143, .F. ) ;
#37547=VERTEX_POINT ( 'NONE', #60775 ) ;
#37558=LINE ( 'NONE', #19026, #3293 ) ;
#37571=( NAMED_UNIT ( * ) PLANE_ANGLE_UNIT ( ) SI_UNIT ( $, .RADIAN. ) );
#37586=CARTESIAN_POINT ( 'NONE',  ( -0.4606233198248986804, 1.422786159591911348, 2.138962479395379646 ) ) ;
#37601=DIRECTION ( 'NONE',  ( 0.000000000000000000, 0.000000000000000000, 1.000000000000000000 ) ) ;
#37615=EDGE_CURVE ( 'NONE', #57884, #25547, #17000, .T. ) ;
#37618=ORIENTED_EDGE ( 'NONE', *, *, #10682, .T. ) ;
#37630=CARTESIAN_POINT ( 'NONE',  ( -0.2517570632375117912, 1.135012049176707949, 1.093517086496077262 ) ) ;
#37631=DIRECTION ( 'NONE',  ( -1.000000000000000000, -0.000000000000000000, -0.000000000000000000 ) ) ;
#37641=DIRECTION ( 'NONE',  ( -0.000000000000000000, -1.000000000000000000, -0.000000000000000000 ) ) ;
#37647=DIRECTION ( 'NONE',  ( 0.000000000000000000, -0.000000000000000000, 1.000000000000000000 ) ) ;
#37657=ORIENTED_EDGE ( 'NONE', *, *, #30323, .T. ) ;
#37660=LINE ( 'NONE', #10771, #39514 ) ;
#37664=DIRECTION ( 'NONE',  ( -0.000000000000000000, -1.000000000000000000, -0.000000000000000000 ) ) ;
#37665=FACE_OUTER_BOUND ( 'NONE', #76177, .T. ) ;
#37680=CARTESIAN_POINT ( 'NONE',  ( 2.129998074986495737, 1.668416680336017865, 0.4562095852119728012 ) ) ;
#37685=EDGE_LOOP ( 'NONE', ( #51100, #78071, #8262, #40629 ) ) ;
#37726=CARTESIAN_POINT ( 'NONE',  ( 0.4476898780826904511, 1.379730629998464631, 2.610432142638456465 ) ) ;
#37729=CIRCLE ( 'NONE', #6793, 0.1771653543307085410 ) ;
#37740=ORIENTED_EDGE ( 'NONE', *, *, #6951, .F. ) ;
#37748=VECTOR ( 'NONE', #34124, 39.37007874015748143 ) ;
#37754=VERTEX_POINT ( 'NONE', #71499 ) ;
#37756=ORIENTED_EDGE ( 'NONE', *, *, #82229, .F. ) ;
#37763=CARTESIAN_POINT ( 'NONE',  ( 2.516666435443586813, 2.742784459617114923, -0.5314960629921260393 ) ) ;
#37775=EDGE_LOOP ( 'NONE', ( #6196, #13015, #11078, #59096, #1634, #30188, #32492, #10222 ) ) ;
#37796=AXIS2_PLACEMENT_3D ( 'NONE', #65610, #7940, #40742 ) ;
#37797=CARTESIAN_POINT ( 'NONE',  ( -3.197598486322605016, 2.742783266281798138, -0.5314960629921260393 ) ) ;
#37801=CARTESIAN_POINT ( 'NONE',  ( -1.964414453380826986, 1.188885443925074004, 0.3231744412230012631 ) ) ;
#37811=AXIS2_PLACEMENT_3D ( 'NONE', #6676, #26869, #374 ) ;
#37834=DIRECTION ( 'NONE',  ( -1.000000000000000000, -1.734723475976808080E-16, -3.491481338843132961E-15 ) ) ;
#37841=ORIENTED_EDGE ( 'NONE', *, *, #511, .F. ) ;
#37858=ORIENTED_EDGE ( 'NONE', *, *, #60347, .F. ) ;
#37866=EDGE_CURVE ( 'NONE', #27190, #79281, #7613, .T. ) ;
#37894=CARTESIAN_POINT ( 'NONE',  ( -2.873110008490984413, 1.063968899401426693, 0.03484477857464209766 ) ) ;
#37908=VECTOR ( 'NONE', #77916, 39.37007874015748143 ) ;
#37910=CARTESIAN_POINT ( 'NONE',  ( -0.4359958488159792478, 1.724409448818897683, 2.094141031014984389 ) ) ;
#37915=CARTESIAN_POINT ( 'NONE',  ( 0.000000000000000000, 2.755905511811024056, 0.000000000000000000 ) ) ;
#37944=CARTESIAN_POINT ( 'NONE',  ( 1.141392835773559211, 0.000000000000000000, 1.456353465694822491 ) ) ;
#37953=CARTESIAN_POINT ( 'NONE',  ( 0.5314960629921395840, 2.755905511811024056, -3.900966923095588346 ) ) ;
#37954=EDGE_LOOP ( 'NONE', ( #21092, #59381, #64170, #65004, #42844, #72213, #78059, #6086, #29289, #20507, #50458, #12117, #75667, #48304, #25513, #75254, #73491, #33064, #54216, #7091, #46954, #47506, #14170, #55044, #42906, #27945, #21914, #15548, #77827, #63222, #397, #47347, #22478, #59192, #81681, #77101 ) ) ;
#37979=CARTESIAN_POINT ( 'NONE',  ( 0.4359958488159307310, 1.724409448818897905, 3.937007874015793885 ) ) ;
#37997=CARTESIAN_POINT ( 'NONE',  ( -0.4741706889230301036, 1.520077057622760464, 2.169554232157526297 ) ) ;
#38012=CARTESIAN_POINT ( 'NONE',  ( 2.611722799339308843, 1.697109554835841916, 0.4469779880792065785 ) ) ;
#38019=DIRECTION ( 'NONE',  ( -0.000000000000000000, 1.000000000000000000, -0.000000000000000000 ) ) ;
#38024=CIRCLE ( 'NONE', #73008, 0.5118110236220472231 ) ;
#38061=VECTOR ( 'NONE', #58937, 39.37007874015748143 ) ;
#38069=EDGE_LOOP ( 'NONE', ( #70659, #24906, #27913, #24107 ) ) ;
#38076=CARTESIAN_POINT ( 'NONE',  ( -1.313877454013331780, 0.2755905511811023723, 0.7983292792091805090 ) ) ;
#38080=CIRCLE ( 'NONE', #16664, 1.122047244094488194 ) ;
#38086=VERTEX_POINT ( 'NONE', #73162 ) ;
#38087=CARTESIAN_POINT ( 'NONE',  ( 2.630268417803912406, 1.724409448818900570, -0.4359958488159719758 ) ) ;
#38090=DIRECTION ( 'NONE',  ( -3.491481338843132961E-15, -0.000000000000000000, 1.000000000000000000 ) ) ;
#38121=AXIS2_PLACEMENT_3D ( 'NONE', #10912, #68981, #63487 ) ;
#38141=EDGE_CURVE ( 'NONE', #57006, #15098, #81544, .T. ) ;
#38163=ADVANCED_FACE ( 'NONE', ( #79082 ), #7529, .F. ) ;
#38166=ORIENTED_EDGE ( 'NONE', *, *, #6316, .T. ) ;
#38168=ORIENTED_EDGE ( 'NONE', *, *, #44178, .F. ) ;
#38178=CARTESIAN_POINT ( 'NONE',  ( 0.9881811337016640495, 2.755905511811024056, 0.5314960629921260393 ) ) ;
#38192=CARTESIAN_POINT ( 'NONE',  ( 1.964921794496066632, 1.189595890467126882, 0.3229789317950442218 ) ) ;
#38201=AXIS2_PLACEMENT_3D ( 'NONE', #53370, #28535, #28948 ) ;
#38230=CARTESIAN_POINT ( 'NONE',  ( -3.931483604541833987, 1.111096610303996091, 0.2104479119174702539 ) ) ;
#38234=CARTESIAN_POINT ( 'NONE',  ( -0.4678115244718906163, 1.617859111677685924, 1.019879954333916761 ) ) ;
#38236=ORIENTED_EDGE ( 'NONE', *, *, #66367, .F. ) ;
#38238=FACE_BOUND ( 'NONE', #44962, .T. ) ;
#38251=ORIENTED_EDGE ( 'NONE', *, *, #67725, .T. ) ;
#38297=EDGE_CURVE ( 'NONE', #50786, #21089, #78826, .T. ) ;
#38316=CIRCLE ( 'NONE', #73252, 0.09842519685039351207 ) ;
#38321=DIRECTION ( 'NONE',  ( 1.000000000000000000, 0.000000000000000000, 3.455050906509825972E-15 ) ) ;
#38323=ADVANCED_FACE ( 'NONE', ( #83189 ), #69327, .F. ) ;
#38325=CARTESIAN_POINT ( 'NONE',  ( 0.4672528563079797470, 1.453807508635538870, -2.153192469889489757 ) ) ;
#38333=EDGE_CURVE ( 'NONE', #2585, #39954, #44044, .T. ) ;
#38353=VERTEX_POINT ( 'NONE', #77719 ) ;
#38368=DIRECTION ( 'NONE',  ( 0.000000000000000000, 0.000000000000000000, 1.000000000000000000 ) ) ;
#38369=CARTESIAN_POINT ( 'NONE',  ( -0.03443470937339728616, 0.2755905511811023723, -1.537015892239756099 ) ) ;
#38388=ORIENTED_EDGE ( 'NONE', *, *, #58809, .T. ) ;
#38393=CARTESIAN_POINT ( 'NONE',  ( -0.03443470937339728616, 0.2755905511811023723, -1.537015892239756099 ) ) ;
#38413=CONICAL_SURFACE ( 'NONE', #14294, 2.637795275590551380, 0.7853981633974500554 ) ;
#38415=CARTESIAN_POINT ( 'NONE',  ( -0.4732338166266092383, 1.502938029856535795, 2.167264197069282528 ) ) ;
#38416=CARTESIAN_POINT ( 'NONE',  ( 0.5314960629921324786, 2.716535433070866645, -1.854472803289050509 ) ) ;
#38420=DIRECTION ( 'NONE',  ( 0.000000000000000000, -1.000000000000000000, 0.000000000000000000 ) ) ;
#38440=FACE_OUTER_BOUND ( 'NONE', #12096, .T. ) ;
#38456=CARTESIAN_POINT ( 'NONE',  ( 1.348312163386739426, 1.062992125984252079, 0.8371118098809627872 ) ) ;
#38490=AXIS2_PLACEMENT_3D ( 'NONE', #58380, #26398, #13367 ) ;
#38494=DIRECTION ( 'NONE',  ( 0.000000000000000000, 1.000000000000000000, 0.000000000000000000 ) ) ;
#38498=EDGE_CURVE ( 'NONE', #29599, #44548, #6210, .T. ) ;
#38504=ORIENTED_EDGE ( 'NONE', *, *, #40133, .T. ) ;
#38508=DIRECTION ( 'NONE',  ( 0.000000000000000000, 0.000000000000000000, 1.000000000000000000 ) ) ;
#38512=ORIENTED_EDGE ( 'NONE', *, *, #7858, .F. ) ;
#38536=CARTESIAN_POINT ( 'NONE',  ( 0.000000000000000000, 0.4177165354330708569, 0.000000000000000000 ) ) ;
#38541=ORIENTED_EDGE ( 'NONE', *, *, #2416, .F. ) ;
#38567=VERTEX_POINT ( 'NONE', #27187 ) ;
#38579=VECTOR ( 'NONE', #58552, 39.37007874015748143 ) ;
#38580=EDGE_CURVE ( 'NONE', #45100, #27310, #79389, .T. ) ;
#38583=ORIENTED_EDGE ( 'NONE', *, *, #30705, .F. ) ;
#38585=VECTOR ( 'NONE', #63981, 39.37007874015748143 ) ;
#38586=ORIENTED_EDGE ( 'NONE', *, *, #9419, .T. ) ;
#38593=CARTESIAN_POINT ( 'NONE',  ( 3.937007874015748143, 2.755905511811024056, 0.5314960629921260393 ) ) ;
#38609=CARTESIAN_POINT ( 'NONE',  ( 2.001206130748399925, 1.231544801320224369, 0.3638227417423782195 ) ) ;
#38622=CARTESIAN_POINT ( 'NONE',  ( -0.09709680097443590396, 1.072984620235833075, -1.483320890666278480 ) ) ;
#38646=AXIS2_PLACEMENT_3D ( 'NONE', #13126, #32047, #7648 ) ;
#38654=CARTESIAN_POINT ( 'NONE',  ( -0.4744094488189005143, 1.537401574803149984, 1.016821367227982220 ) ) ;
#38671=ORIENTED_EDGE ( 'NONE', *, *, #53241, .T. ) ;
#38682=CARTESIAN_POINT ( 'NONE',  ( 0.4698620426710066744, 1.469755830210690117, -2.565186897544956324 ) ) ;
#38688=ORIENTED_EDGE ( 'NONE', *, *, #79768, .T. ) ;
#38709=VECTOR ( 'NONE', #34010, 39.37007874015748143 ) ;
#38748=CARTESIAN_POINT ( 'NONE',  ( -0.4029448339610336438, 1.286526487772640115, -3.916342797992894198 ) ) ;
#38764=DIRECTION ( 'NONE',  ( -0.000000000000000000, -1.000000000000000000, -0.000000000000000000 ) ) ;
#38768=VERTEX_POINT ( 'NONE', #4425 ) ;
#38787=VERTEX_POINT ( 'NONE', #28853 ) ;
#38790=EDGE_LOOP ( 'NONE', ( #77079, #50185, #31340, #78141, #67792, #32876, #69963, #18092 ) ) ;
#38804=EDGE_CURVE ( 'NONE', #69251, #11040, #36409, .T. ) ;
#38806=FACE_OUTER_BOUND ( 'NONE', #27955, .T. ) ;
#38812=DIRECTION ( 'NONE',  ( 1.047444401652940007E-14, -0.000000000000000000, -1.000000000000000000 ) ) ;
#38817=CARTESIAN_POINT ( 'NONE',  ( 0.4359958488159610956, 1.724409448818897461, 1.033875059083681158 ) ) ;
#38832=CARTESIAN_POINT ( 'NONE',  ( -0.3227188174119199338, 1.189353863002643896, 1.964709871421637555 ) ) ;
#38846=CARTESIAN_POINT ( 'NONE',  ( 0.000000000000000000, 2.755905511811024056, 0.000000000000000000 ) ) ;
#38867=VECTOR ( 'NONE', #948, 39.37007874015748143 ) ;
#38868=EDGE_CURVE ( 'NONE', #41210, #39595, #47906, .T. ) ;
#38909=LINE ( 'NONE', #33012, #34251 ) ;
#38918=CARTESIAN_POINT ( 'NONE',  ( -1.119414574269209650, 1.069244457019925765, -0.07832840781635802552 ) ) ;
#38921=DIRECTION ( 'NONE',  ( 0.000000000000000000, -1.000000000000000000, 0.000000000000000000 ) ) ;
#38925=ORIENTED_EDGE ( 'NONE', *, *, #82772, .F. ) ;
#38979=ORIENTED_EDGE ( 'NONE', *, *, #25459, .T. ) ;
#38996=ORIENTED_EDGE ( 'NONE', *, *, #66014, .T. ) ;
#39020=CARTESIAN_POINT ( 'NONE',  ( 2.105021046755494396, 1.366082762360720348, 0.4426340671871338284 ) ) ;
#39063=CARTESIAN_POINT ( 'NONE',  ( -3.910145899155770710, 1.414046480882519941, -0.4591600588675787686 ) ) ;
#39070=ORIENTED_EDGE ( 'NONE', *, *, #15443, .F. ) ;
#39071=CIRCLE ( 'NONE', #21664, 2.204724409448819422 ) ;
#39072=CYLINDRICAL_SURFACE ( 'NONE', #56591, 0.5118110236220471121 ) ;
#39102=VERTEX_POINT ( 'NONE', #41891 ) ;
#39116=CARTESIAN_POINT ( 'NONE',  ( -2.554860351194724544, 1.554815631980118740, 0.4741686481756392513 ) ) ;
#39133=AXIS2_PLACEMENT_3D ( 'NONE', #74150, #79648, #55175 ) ;
#39164=CARTESIAN_POINT ( 'NONE',  ( -0.6299212598425228959, 1.724409448818897905, 0.9285414500055694242 ) ) ;
#39174=DIRECTION ( 'NONE',  ( -0.000000000000000000, 1.000000000000000000, -0.000000000000000000 ) ) ;
#39198=CARTESIAN_POINT ( 'NONE',  ( 0.5314960629921350321, 2.755905511811024056, -2.583694225513478937 ) ) ;
#39205=EDGE_LOOP ( 'NONE', ( #52352, #26863, #46541, #32491 ) ) ;
#39220=CARTESIAN_POINT ( 'NONE',  ( 0.3149606299212736604, 2.559055118110236560, -3.937007874015761022 ) ) ;
#39223=ORIENTED_EDGE ( 'NONE', *, *, #21721, .T. ) ;
#39239=AXIS2_PLACEMENT_3D ( 'NONE', #66606, #8942, #34617 ) ;
#39249=PLANE ( 'NONE',  #76156 ) ;
#39253=CARTESIAN_POINT ( 'NONE',  ( -0.03443470937339728616, 0.2755905511811023723, -1.537015892239756099 ) ) ;
#39260=CARTESIAN_POINT ( 'NONE',  ( 1.028050040965491130, 1.383304877436015490, -0.4497434709457576729 ) ) ;
#39263=CARTESIAN_POINT ( 'NONE',  ( 0.2506648432407165838, 1.134319890641129813, 3.929041500980708701 ) ) ;
#39276=DIRECTION ( 'NONE',  ( 1.000000000000000000, 0.000000000000000000, 3.455050906509825972E-15 ) ) ;
#39331=ORIENTED_EDGE ( 'NONE', *, *, #40826, .T. ) ;
#39333=DIRECTION ( 'NONE',  ( 0.000000000000000000, 1.000000000000000000, -8.673617379884024625E-16 ) ) ;
#39339=EDGE_LOOP ( 'NONE', ( #55027, #22744, #80448, #4340 ) ) ;
#39340=CARTESIAN_POINT ( 'NONE',  ( -1.881759047730065859, 2.742776634745604625, -0.5314960629921260393 ) ) ;
#39342=EDGE_CURVE ( 'NONE', #46748, #30815, #69424, .T. ) ;
#39351=ADVANCED_FACE ( 'NONE', ( #77195 ), #78882, .F. ) ;
#39374=EDGE_CURVE ( 'NONE', #29467, #21709, #29174, .T. ) ;
#39402=ORIENTED_EDGE ( 'NONE', *, *, #79045, .T. ) ;
#39403=ORIENTED_EDGE ( 'NONE', *, *, #3774, .F. ) ;
#39410=CARTESIAN_POINT ( 'NONE',  ( 0.5314960629920847390, 2.755905511811024056, 3.937007874015794773 ) ) ;
#39419=VERTEX_POINT ( 'NONE', #30913 ) ;
#39445=CARTESIAN_POINT ( 'NONE',  ( -0.4744094488189105063, 1.521916954317726667, 3.908320185825789217 ) ) ;
#39473=FACE_OUTER_BOUND ( 'NONE', #78112, .T. ) ;
#39474=CIRCLE ( 'NONE', #12618, 1.122047244094488194 ) ;
#39480=CARTESIAN_POINT ( 'NONE',  ( -1.559171609364246924, 0.3937007874015747699, 0.4177787735906735578 ) ) ;
#39489=DIRECTION ( 'NONE',  ( 1.000000000000000000, -0.000000000000000000, -0.000000000000000000 ) ) ;
#39491=CARTESIAN_POINT ( 'NONE',  ( 0.4563452811745912219, 0.01305114060239447211, 2.130073781772667374 ) ) ;
#39504=CARTESIAN_POINT ( 'NONE',  ( 0.3765731398154819609, 1.248435479399690573, -3.918969628814140904 ) ) ;
#39508=ORIENTED_EDGE ( 'NONE', *, *, #82082, .T. ) ;
#39514=VECTOR ( 'NONE', #74751, 39.37007874015748143 ) ;
#39525=ORIENTED_EDGE ( 'NONE', *, *, #6951, .T. ) ;
#39528=CARTESIAN_POINT ( 'NONE',  ( 2.585342365690415978, 1.422987107291905362, 0.4606739315415591673 ) ) ;
#39533=VECTOR ( 'NONE', #9290, 39.37007874015748143 ) ;
#39562=CARTESIAN_POINT ( 'NONE',  ( 1.150409065943327480, 0.1377952755905511861, 0.8265612839971842041 ) ) ;
#39579=CIRCLE ( 'NONE', #81295, 0.5118110236220472231 ) ;
#39587=FACE_OUTER_BOUND ( 'NONE', #11796, .T. ) ;
#39593=DIRECTION ( 'NONE',  ( 0.000000000000000000, -1.601283208593976204E-15, -1.000000000000000000 ) ) ;
#39595=VERTEX_POINT ( 'NONE', #13882 ) ;
#39601=LINE ( 'NONE', #8453, #37748 ) ;
#39611=ORIENTED_EDGE ( 'NONE', *, *, #1240, .F. ) ;
#39618=DIRECTION ( 'NONE',  ( 0.000000000000000000, 0.000000000000000000, -1.000000000000000000 ) ) ;
#39626=CARTESIAN_POINT ( 'NONE',  ( -0.3149606299212459048, 2.165354330708661568, -3.924389226575469625 ) ) ;
#39629=ORIENTED_EDGE ( 'NONE', *, *, #46415, .T. ) ;
#39647=CARTESIAN_POINT ( 'NONE',  ( 0.4177787735907000366, 0.3937007874015748254, -1.736336963694947944 ) ) ;
#39649=VERTEX_POINT ( 'NONE', #58901 ) ;
#39679=CARTESIAN_POINT ( 'NONE',  ( -0.4744094488189043446, 1.546132656481028933, 2.170146923806632433 ) ) ;
#39685=CARTESIAN_POINT ( 'NONE',  ( 1.016821367227983997, 1.521771543437157481, -0.4744094488188971281 ) ) ;
#39688=DIRECTION ( 'NONE',  ( -0.000000000000000000, -1.000000000000000000, -0.000000000000000000 ) ) ;
#39702=CYLINDRICAL_SURFACE ( 'NONE', #11073, 0.4744094488188972947 ) ;
#39722=CARTESIAN_POINT ( 'NONE',  ( 0.4114485906785895208, 1.299212774617487076, 1.044049266805401999 ) ) ;
#39742=VERTEX_POINT ( 'NONE', #26909 ) ;
#39745=CARTESIAN_POINT ( 'NONE',  ( 2.118110236220474007, 0.000000000000000000, -0.4498537592782824723 ) ) ;
#39747=DIRECTION ( 'NONE',  ( 0.000000000000000000, 0.000000000000000000, -1.000000000000000000 ) ) ;
#39750=CARTESIAN_POINT ( 'NONE',  ( 1.141392835773559211, 0.3937007874015748254, 1.141392835773562764 ) ) ;
#39753=ORIENTED_EDGE ( 'NONE', *, *, #9731, .F. ) ;
#39755=CARTESIAN_POINT ( 'NONE',  ( 0.000000000000000000, 0.4201155382560080032, -1.198416298106748767 ) ) ;
#39757=CARTESIAN_POINT ( 'NONE',  ( -3.937007874015748143, 1.724409448818898127, -0.6299212598425202314 ) ) ;
#39758=DIRECTION ( 'NONE',  ( 1.000000000000000000, -0.000000000000000000, -0.000000000000000000 ) ) ;
#39762=CIRCLE ( 'NONE', #26296, 0.1771653543307085410 ) ;
#39764=CARTESIAN_POINT ( 'NONE',  ( -0.5314960629921194890, 2.716535433070866645, -1.854472803289054283 ) ) ;
#39765=DIRECTION ( 'NONE',  ( 0.000000000000000000, -1.000000000000000000, 0.000000000000000000 ) ) ;
#39791=CARTESIAN_POINT ( 'NONE',  ( 1.403614904275686858E-14, 1.537401574803149984, -3.937007874015761910 ) ) ;
#39798=EDGE_CURVE ( 'NONE', #19015, #53614, #22199, .T. ) ;
#39801=AXIS2_PLACEMENT_3D ( 'NONE', #70930, #45646, #19152 ) ;
#39806=AXIS2_PLACEMENT_3D ( 'NONE', #65572, #8315, #47426 ) ;
#39814=CARTESIAN_POINT ( 'NONE',  ( 0.4744094488188886904, 1.537401574803149984, 2.554262525012303886 ) ) ;
#39829=EDGE_LOOP ( 'NONE', ( #14790, #61786, #16447, #69659 ) ) ;
#39845=ORIENTED_EDGE ( 'NONE', *, *, #22547, .T. ) ;
#39856=CARTESIAN_POINT ( 'NONE',  ( 0.4668652553835576646, 1.622068519643046436, 2.152447471807370061 ) ) ;
#39862=ORIENTED_EDGE ( 'NONE', *, *, #54110, .F. ) ;
#39867=( NAMED_UNIT ( * ) SI_UNIT ( $, .STERADIAN. ) SOLID_ANGLE_UNIT ( ) );
#39870=CARTESIAN_POINT ( 'NONE',  ( 2.058022911372368480, 1.301102360844744510, 0.4123394245947664682 ) ) ;
#39875=AXIS2_PLACEMENT_3D ( 'NONE', #15634, #30299, #55139 ) ;
#39880=CARTESIAN_POINT ( 'NONE',  ( -0.5314960629921372526, 2.716535433070866645, 3.224202737261813834 ) ) ;
#39895=CARTESIAN_POINT ( 'NONE',  ( -0.4736019971540468276, 1.569430237215018176, -1.017199299814984359 ) ) ;
#39897=CARTESIAN_POINT ( 'NONE',  ( 0.3149606299212636684, 2.559055118110236560, -1.076935383196056195 ) ) ;
#39901=LINE ( 'NONE', #26845, #66741 ) ;
#39907=EDGE_CURVE ( 'NONE', #76998, #45287, #81579, .T. ) ;
#39913=CARTESIAN_POINT ( 'NONE',  ( -0.9881811337016640495, 2.559055118110236560, -0.5314960629921260393 ) ) ;
#39919=ORIENTED_EDGE ( 'NONE', *, *, #61425, .F. ) ;
#39920=CARTESIAN_POINT ( 'NONE',  ( 0.4470386624395689124, 1.696927142811738287, -2.611610595642054999 ) ) ;
#39923=VECTOR ( 'NONE', #33503, 39.37007874015748854 ) ;
#39929=CARTESIAN_POINT ( 'NONE',  ( -3.912791665790199769, 1.724409448818897905, 0.4359958488159718093 ) ) ;
#39930=AXIS2_PLACEMENT_3D ( 'NONE', #56496, #57313, #83011 ) ;
#39932=CARTESIAN_POINT ( 'NONE',  ( 3.884512598959606322, 2.725419031863056230, 0.5314960629921259283 ) ) ;
#39938=ORIENTED_EDGE ( 'NONE', *, *, #80504, .T. ) ;
#39944=ADVANCED_FACE ( 'NONE', ( #10476 ), #61802, .T. ) ;
#39954=VERTEX_POINT ( 'NONE', #80362 ) ;
#39957=CARTESIAN_POINT ( 'NONE',  ( -1.428351447576950095, 1.168345958003150331, 0.2981497428225624580 ) ) ;
#39989=LINE ( 'NONE', #31995, #49345 ) ;
#39997=FACE_OUTER_BOUND ( 'NONE', #63429, .T. ) ;
#40005=DIRECTION ( 'NONE',  ( 0.000000000000000000, 0.000000000000000000, -1.000000000000000000 ) ) ;
#40020=DIRECTION ( 'NONE',  ( -0.000000000000000000, -1.000000000000000000, -0.000000000000000000 ) ) ;
#40032=CARTESIAN_POINT ( 'NONE',  ( 0.6299212598424790421, 1.724409448818897905, 3.886287458032468667 ) ) ;
#40036=ORIENTED_EDGE ( 'NONE', *, *, #52190, .T. ) ;
#40068=CARTESIAN_POINT ( 'NONE',  ( -0.5314960629921392510, 2.753420937170568461, 3.841955293929014026 ) ) ;
#40070=CARTESIAN_POINT ( 'NONE',  ( 3.926395708098648907, 1.160952188075316860, -0.2891268611046654002 ) ) ;
#40078=B_SPLINE_CURVE_WITH_KNOTS ( 'NONE', 3,
 ( #77748, #57939, #71427, #19652, #45731, #33124 ),
 .UNSPECIFIED., .F., .F.,
 ( 4, 2, 4 ),
 ( 0.008003512672130536076, 0.008448156958474645206, 0.008892801244818756071 ),
 .UNSPECIFIED. ) ;
#40104=FACE_OUTER_BOUND ( 'NONE', #79621, .T. ) ;
#40106=VECTOR ( 'NONE', #42387, 39.37007874015748143 ) ;
#40108=CARTESIAN_POINT ( 'NONE',  ( 0.3567026107877686592, 1.224237700298272502, 3.920828153186683096 ) ) ;
#40121=ADVANCED_FACE ( 'NONE', ( #15550 ), #73626, .F. ) ;
#40133=EDGE_CURVE ( 'NONE', #46648, #29487, #74031, .T. ) ;
#40143=CARTESIAN_POINT ( 'NONE',  ( -0.4670044181572561293, 1.622388320715300702, -2.152632970815978375 ) ) ;
#40163=VERTEX_POINT ( 'NONE', #42024 ) ;
#40166=CARTESIAN_POINT ( 'NONE',  ( 1.141392835773559211, 0.3937007874015748254, 0.9642274814428540841 ) ) ;
#40167=CARTESIAN_POINT ( 'NONE',  ( -0.4732412630952499977, 1.503056026428865710, 2.557127100491988880 ) ) ;
#40171=CARTESIAN_POINT ( 'NONE',  ( -3.937007874015748143, 2.165354330708661568, 0.3149606299212595606 ) ) ;
#40174=ORIENTED_EDGE ( 'NONE', *, *, #60737, .T. ) ;
#40179=DIRECTION ( 'NONE',  ( 0.000000000000000000, 0.000000000000000000, -1.000000000000000000 ) ) ;
#40185=CARTESIAN_POINT ( 'NONE',  ( 2.362204724409448620, 0.03937007874015751446, 8.247593713802677664E-15 ) ) ;
#40191=EDGE_CURVE ( 'NONE', #64262, #12714, #20106, .T. ) ;
#40204=AXIS2_PLACEMENT_3D ( 'NONE', #13991, #13155, #70802 ) ;
#40231=CARTESIAN_POINT ( 'NONE',  ( 3.937007874015748143, 2.559055118110236560, -0.5314960629921260393 ) ) ;
#40243=ORIENTED_EDGE ( 'NONE', *, *, #14729, .F. ) ;
#40258=ORIENTED_EDGE ( 'NONE', *, *, #47021, .F. ) ;
#40260=VERTEX_POINT ( 'NONE', #55468 ) ;
#40261=CARTESIAN_POINT ( 'NONE',  ( -1.409919628453981888, 1.316123991182629460, 0.4200987300965431936 ) ) ;
#40277=ORIENTED_EDGE ( 'NONE', *, *, #21499, .T. ) ;
#40309=B_SPLINE_CURVE_WITH_KNOTS ( 'NONE', 3,
 ( #42593, #68293, #60715, #67876, #80923, #9379, #42997, #61958, #4298, #41365, #29961, #4702, #75021, #48489, #16952, #73781, #10213, #54392, #55626, #16117, #47665, #67046 ),
 .UNSPECIFIED., .F., .F.,
 ( 4, 2, 2, 2, 2, 2, 2, 2, 2, 2, 4 ),
 ( 0.000000000000000000, 0.002126047124880315557, 0.003189070687320475720, 0.003720582468540548429, 0.004252094249760621572, 0.005315117812200776531, 0.005846629593420847940, 0.006378141374640921082, 0.006909653155860992491, 0.007441164937081065633, 0.008504188499521210184 ),
 .UNSPECIFIED. ) ;
#40316=DIRECTION ( 'NONE',  ( 0.000000000000000000, 0.000000000000000000, -1.000000000000000000 ) ) ;
#40318=CARTESIAN_POINT ( 'NONE',  ( -1.382164990278195615, 1.299212598425196985, 0.4102808022082835571 ) ) ;
#40333=CARTESIAN_POINT ( 'NONE',  ( -3.826707563893392283, 2.755905511811024500, -0.5314960629921261503 ) ) ;
#40336=EDGE_CURVE ( 'NONE', #72978, #50169, #11716, .T. ) ;
#40366=CARTESIAN_POINT ( 'NONE',  ( 2.846947862837586829, 1.092324130688943296, 0.1650676745531752254 ) ) ;
#40392=EDGE_CURVE ( 'NONE', #4444, #41297, #42158, .T. ) ;
#40399=DIRECTION ( 'NONE',  ( 1.000000000000000000, -0.000000000000000000, -0.000000000000000000 ) ) ;
#40405=CARTESIAN_POINT ( 'NONE',  ( -2.153082335389848279, 1.453547212638083952, -0.4672029448317642775 ) ) ;
#40438=CARTESIAN_POINT ( 'NONE',  ( -3.937007874015748143, 1.724409448818897905, 0.4359958488159719758 ) ) ;
#40450=VERTEX_POINT ( 'NONE', #10876 ) ;
#40464=ADVANCED_FACE ( 'NONE', ( #36537 ), #33201, .F. ) ;
#40470=VERTEX_POINT ( 'NONE', #30221 ) ;
#40487=CARTESIAN_POINT ( 'NONE',  ( 3.913920805910253264, 1.327648775429739025, -0.4258039130830911789 ) ) ;
#40490=DIRECTION ( 'NONE',  ( 0.000000000000000000, -1.000000000000000000, 0.000000000000000000 ) ) ;
#40496=DIRECTION ( 'NONE',  ( -0.000000000000000000, -1.000000000000000000, -0.000000000000000000 ) ) ;
#40503=CARTESIAN_POINT ( 'NONE',  ( -0.4253597317562083369, 1.326753431064211952, -1.038326151780470497 ) ) ;
#40510=CARTESIAN_POINT ( 'NONE',  ( 0.000000000000000000, 2.677165354330708791, 0.000000000000000000 ) ) ;
#40519=AXIS2_PLACEMENT_3D ( 'NONE', #26864, #20974, #72329 ) ;
#40522=CARTESIAN_POINT ( 'NONE',  ( 1.077407372805332830, 1.181077650421485936, -0.3135877947998832460 ) ) ;
#40525=CARTESIAN_POINT ( 'NONE',  ( 0.4441491729173822067, 1.369957082458975739, 3.911879148534922024 ) ) ;
#40538=DIRECTION ( 'NONE',  ( 0.000000000000000000, 1.000000000000000000, -0.000000000000000000 ) ) ;
#40547=CARTESIAN_POINT ( 'NONE',  ( 3.821484228344193657, 2.755905511811024056, -0.5314960629921260393 ) ) ;
#40556=CARTESIAN_POINT ( 'NONE',  ( 0.4744094488188940750, 1.537401574803149984, 1.016821367227985329 ) ) ;
#40578=CARTESIAN_POINT ( 'NONE',  ( 3.237502119437988046, 2.729657717072965006, -0.5314960629921260393 ) ) ;
#40579=CARTESIAN_POINT ( 'NONE',  ( 0.5314960629920921775, 2.716535433070866645, 3.224202737261820939 ) ) ;
#40586=VERTEX_POINT ( 'NONE', #23912 ) ;
#40588=CARTESIAN_POINT ( 'NONE',  ( -1.063894186419820809, 1.223759533161110635, -0.3572641188300489934 ) ) ;
#40595=ORIENTED_EDGE ( 'NONE', *, *, #44899, .F. ) ;
#40597=PLANE ( 'NONE',  #23694 ) ;
#40629=ORIENTED_EDGE ( 'NONE', *, *, #53064, .F. ) ;
#40670=ORIENTED_EDGE ( 'NONE', *, *, #58210, .F. ) ;
#40672=ORIENTED_EDGE ( 'NONE', *, *, #25177, .T. ) ;
#40673=LINE ( 'NONE', #67606, #15323 ) ;
#40679=FACE_BOUND ( 'NONE', #16176, .T. ) ;
#40687=CARTESIAN_POINT ( 'NONE',  ( 0.5314960629921395840, 2.716830163678111365, -3.890345922373657839 ) ) ;
#40688=ORIENTED_EDGE ( 'NONE', *, *, #82913, .T. ) ;
#40693=CARTESIAN_POINT ( 'NONE',  ( 2.169549780153825047, 1.520054044952883210, -0.4741688556381175590 ) ) ;
#40694=EDGE_CURVE ( 'NONE', #47373, #38567, #61238, .T. ) ;
#40717=CARTESIAN_POINT ( 'NONE',  ( 0.4436160793303255412, 1.369148167000072247, -1.503412402614913379 ) ) ;
#40727=EDGE_CURVE ( 'NONE', #45287, #66126, #46644, .T. ) ;
#40740=VECTOR ( 'NONE', #8859, 39.37007874015748143 ) ;
#40742=DIRECTION ( 'NONE',  ( 0.000000000000000000, 0.000000000000000000, -1.000000000000000000 ) ) ;
#40769=ORIENTED_EDGE ( 'NONE', *, *, #66014, .F. ) ;
#40771=EDGE_LOOP ( 'NONE', ( #14565, #71518 ) ) ;
#40774=CARTESIAN_POINT ( 'NONE',  ( -1.441491218394533647, 1.158252404499417576, 0.2851933289425553353 ) ) ;
#40802=VECTOR ( 'NONE', #67704, 39.37007874015748143 ) ;
#40816=CARTESIAN_POINT ( 'NONE',  ( -0.5314960629921124946, 2.740199102106095186, -3.870235431238102208 ) ) ;
#40826=EDGE_CURVE ( 'NONE', #79281, #28871, #47971, .T. ) ;
#40858=ORIENTED_EDGE ( 'NONE', *, *, #44641, .F. ) ;
#40860=CIRCLE ( 'NONE', #51577, 2.637795275590551380 ) ;
#40881=VERTEX_POINT ( 'NONE', #73051 ) ;
#40903=CARTESIAN_POINT ( 'NONE',  ( -0.5314960629921323676, 2.755905511811024056, 1.813482582612291560 ) ) ;
#40909=DIRECTION ( 'NONE',  ( -0.8660254037844433705, 0.000000000000000000, 0.4999999999999920064 ) ) ;
#40920=EDGE_CURVE ( 'NONE', #11040, #36023, #15401, .T. ) ;
#40927=AXIS2_PLACEMENT_3D ( 'NONE', #79749, #9440, #80990 ) ;
#40934=ADVANCED_FACE ( 'NONE', ( #23352 ), #62074, .F. ) ;
#40935=CARTESIAN_POINT ( 'NONE',  ( -0.03443470937343537375, 1.064243487142137568, -1.440673310089392478 ) ) ;
#40960=EDGE_LOOP ( 'NONE', ( #49542, #79185, #24729, #79531 ) ) ;
#40974=CARTESIAN_POINT ( 'NONE',  ( 0.2389359915688108460, 1.126391250279107137, 1.096629699561409987 ) ) ;
#40981=AXIS2_PLACEMENT_3D ( 'NONE', #75582, #37265, #70065 ) ;
#41001=DIRECTION ( 'NONE',  ( 0.000000000000000000, 1.000000000000000000, 0.000000000000000000 ) ) ;
#41007=VERTEX_POINT ( 'NONE', #28842 ) ;
#41011=DIRECTION ( 'NONE',  ( 0.000000000000000000, 8.326672684688674053E-16, 1.000000000000000000 ) ) ;
#41016=CARTESIAN_POINT ( 'NONE',  ( -0.5314960629921122726, 2.559055118110236560, -3.937007874015763687 ) ) ;
#41023=FACE_OUTER_BOUND ( 'NONE', #3319, .T. ) ;
#41037=VECTOR ( 'NONE', #23372, 39.37007874015748143 ) ;
#41042=DIRECTION ( 'NONE',  ( -3.491481338843133355E-15, -0.000000000000000000, 1.000000000000000000 ) ) ;
#41045=CARTESIAN_POINT ( 'NONE',  ( -1.813482582612293559, 2.755905511811024056, 0.5314960629921260393 ) ) ;
#41075=ORIENTED_EDGE ( 'NONE', *, *, #60880, .T. ) ;
#41081=DIRECTION ( 'NONE',  ( -8.673617379884021667E-16, 1.000000000000000000, -3.028377322213054317E-30 ) ) ;
#41093=EDGE_LOOP ( 'NONE', ( #16851, #28043, #62836, #56246, #67271, #4634, #79602, #5836, #368, #16264, #80765, #21230, #52133, #61457 ) ) ;
#41100=CARTESIAN_POINT ( 'NONE',  ( 1.840814904541342001, 2.729664745829105232, -0.5314960629921260393 ) ) ;
#41114=CARTESIAN_POINT ( 'NONE',  ( 1.851423525050895247, 1.064103292658514777, -0.03357545743408756056 ) ) ;
#41121=DIRECTION ( 'NONE',  ( -0.000000000000000000, 1.000000000000000000, -0.000000000000000000 ) ) ;
#41135=VECTOR ( 'NONE', #54958, 39.37007874015748143 ) ;
#41145=LINE ( 'NONE', #3676, #77065 ) ;
#41150=CIRCLE ( 'NONE', #54537, 0.09842519685039351207 ) ;
#41156=CARTESIAN_POINT ( 'NONE',  ( 0.3149606299212185379, 2.559055118110236560, 3.924389226575471845 ) ) ;
#41170=CARTESIAN_POINT ( 'NONE',  ( 3.821484228344193657, 2.755905511811024056, 0.5314960629921260393 ) ) ;
#41175=EDGE_CURVE ( 'NONE', #9799, #16468, #3653, .T. ) ;
#41189=ORIENTED_EDGE ( 'NONE', *, *, #22645, .F. ) ;
#41191=EDGE_LOOP ( 'NONE', ( #52870, #17795, #27130, #70073 ) ) ;
#41196=DIRECTION ( 'NONE',  ( 0.8660254037844361541, 0.000000000000000000, 0.5000000000000043299 ) ) ;
#41202=CARTESIAN_POINT ( 'NONE',  ( -3.924389226575468737, 2.559055118110236560, 0.3149606299212596716 ) ) ;
#41210=VERTEX_POINT ( 'NONE', #83084 ) ;
#41218=AXIS2_PLACEMENT_3D ( 'NONE', #79226, #68952, #11723 ) ;
#41236=CARTESIAN_POINT ( 'NONE',  ( -2.020039340939639771, 1.253873987468399509, -0.3814095263789812895 ) ) ;
#41242=EDGE_CURVE ( 'NONE', #34982, #44828, #17884, .T. ) ;
#41257=CARTESIAN_POINT ( 'NONE',  ( 3.937007874015748143, 2.165354330708662012, 0.6299212598425202314 ) ) ;
#41276=VERTEX_POINT ( 'NONE', #50665 ) ;
#41285=CARTESIAN_POINT ( 'NONE',  ( 0.05803841145411302999, 1.066555667699313759, -1.527167351498692538 ) ) ;
#41291=CARTESIAN_POINT ( 'NONE',  ( -1.559171609364246924, 1.299212598425196985, 0.5949441279213820710 ) ) ;
#41297=VERTEX_POINT ( 'NONE', #56976 ) ;
#41310=EDGE_CURVE ( 'NONE', #21631, #28101, #58238, .T. ) ;
#41314=EDGE_CURVE ( 'NONE', #21419, #24203, #73338, .T. ) ;
#41317=CARTESIAN_POINT ( 'NONE',  ( 3.933488357682179970, 1.093105643167624930, 0.1670540113780165925 ) ) ;
#41336=CARTESIAN_POINT ( 'NONE',  ( -0.06298769380853883049, 1.066927083894429140, -1.120388281904474814 ) ) ;
#41365=CARTESIAN_POINT ( 'NONE',  ( -1.690245196119324333, 1.168079626289185269, 0.2980098697639514405 ) ) ;
#41367=CARTESIAN_POINT ( 'NONE',  ( -0.5314960629921349211, 2.742779892193532909, 2.570293763077048155 ) ) ;
#41380=CARTESIAN_POINT ( 'NONE',  ( -0.1243525380209066500, 1.078522938818520238, 1.115555442254801077 ) ) ;
#41383=EDGE_CURVE ( 'NONE', #72444, #6265, #30492, .T. ) ;
#41404=CARTESIAN_POINT ( 'NONE',  ( 0.000000000000000000, 1.724409448818897461, 0.000000000000000000 ) ) ;
#41406=ORIENTED_EDGE ( 'NONE', *, *, #49802, .F. ) ;
#41407=ORIENTED_EDGE ( 'NONE', *, *, #20457, .T. ) ;
#41410=CYLINDRICAL_SURFACE ( 'NONE', #49811, 0.4744094488188972947 ) ;
#41411=LINE ( 'NONE', #78484, #779 ) ;
#41413=CYLINDRICAL_SURFACE ( 'NONE', #17692, 0.09842519685039351207 ) ;
#41419=ORIENTED_EDGE ( 'NONE', *, *, #9160, .F. ) ;
#41425=FACE_OUTER_BOUND ( 'NONE', #63094, .T. ) ;
#41427=AXIS2_PLACEMENT_3D ( 'NONE', #38846, #6863, #58196 ) ;
#41428=DIRECTION ( 'NONE',  ( 0.000000000000000000, 1.000000000000000000, -0.000000000000000000 ) ) ;
#41448=EDGE_CURVE ( 'NONE', #4880, #38353, #31729, .T. ) ;
#41456=CARTESIAN_POINT ( 'NONE',  ( 0.4606976121171817429, 1.423084236280321324, 2.139116380834042541 ) ) ;
#41459=EDGE_CURVE ( 'NONE', #51397, #30609, #72198, .T. ) ;
#41488=ORIENTED_EDGE ( 'NONE', *, *, #6986, .F. ) ;
#41491=EDGE_CURVE ( 'NONE', #74617, #60812, #12050, .T. ) ;
#41496=DIRECTION ( 'NONE',  ( 0.000000000000000000, 0.000000000000000000, -1.000000000000000000 ) ) ;
#41506=ORIENTED_EDGE ( 'NONE', *, *, #32892, .T. ) ;
#41509=CARTESIAN_POINT ( 'NONE',  ( -1.382164990278195615, 1.299212598425196985, 0.4102808022082835571 ) ) ;
#41549=ADVANCED_FACE ( 'NONE', ( #36809 ), #24176, .F. ) ;
#41556=DIRECTION ( 'NONE',  ( 0.000000000000000000, 0.000000000000000000, -1.000000000000000000 ) ) ;
#41604=B_SPLINE_CURVE_WITH_KNOTS ( 'NONE', 3,
 ( #66884, #71944, #14296, #60548, #27313, #8795, #66459, #34049, #78686, #40774, #73613, #39957, #52972, #21009, #72363, #59712, #29387, #68522, #24303, #74018 ),
 .UNSPECIFIED., .F., .F.,
 ( 4, 2, 2, 2, 2, 2, 2, 2, 2, 4 ),
 ( 0.008504188499521210184, 0.009565469904607836610, 0.01009611060715114028, 0.01062675130969444395, 0.01168803271478104956, 0.01221867341732434456, 0.01274931411986764129, 0.01381059552495423129, 0.01487187693004082129, 0.01699443974021398046 ),
 .UNSPECIFIED. ) ;
#41613=ORIENTED_EDGE ( 'NONE', *, *, #38580, .T. ) ;
#41616=VERTEX_POINT ( 'NONE', #46008 ) ;
#41641=EDGE_CURVE ( 'NONE', #12714, #22431, #15737, .T. ) ;
#41643=CARTESIAN_POINT ( 'NONE',  ( -2.139011644334197104, 1.422882880004775918, -0.4606469518571241206 ) ) ;
#41671=CARTESIAN_POINT ( 'NONE',  ( 0.2510736293007090891, 1.134572453438782214, 2.808463035490861071 ) ) ;
#41682=ORIENTED_EDGE ( 'NONE', *, *, #4697, .F. ) ;
#41688=CARTESIAN_POINT ( 'NONE',  ( -0.4732141852945584981, 1.572163861244849636, -2.557193068050839013 ) ) ;
#41705=AXIS2_PLACEMENT_3D ( 'NONE', #78064, #20394, #19135 ) ;
#41725=LINE ( 'NONE', #61915, #75446 ) ;
#41747=CARTESIAN_POINT ( 'NONE',  ( 6.372542394380578105E-15, 1.062992125984252523, -1.629220936382730134 ) ) ;
#41761=VECTOR ( 'NONE', #74024, 39.37007874015748143 ) ;
#41790=CARTESIAN_POINT ( 'NONE',  ( -0.03443470937339728616, 0.2929341459200028863, -1.635441089090149402 ) ) ;
#41808=VERTEX_POINT ( 'NONE', #64973 ) ;
#41811=LINE ( 'NONE', #20916, #33728 ) ;
#41812=DIRECTION ( 'NONE',  ( -3.491481338843132961E-15, -0.000000000000000000, 1.000000000000000000 ) ) ;
#41814=CARTESIAN_POINT ( 'NONE',  ( -0.4744094488189106174, 1.537401574803149984, 3.908320185825790105 ) ) ;
#41823=CIRCLE ( 'NONE', #47171, 1.122047244094488194 ) ;
#41825=CARTESIAN_POINT ( 'NONE',  ( -1.028258860871784197, 1.383740025641660543, 0.4491090030276655432 ) ) ;
#41827=DIRECTION ( 'NONE',  ( 1.000000000000000000, -0.000000000000000000, -0.000000000000000000 ) ) ;
#41828=CARTESIAN_POINT ( 'NONE',  ( -3.937007874015748143, 2.559055118110236560, 0.3149606299212596716 ) ) ;
#41833=DIRECTION ( 'NONE',  ( -0.000000000000000000, -1.000000000000000000, -0.000000000000000000 ) ) ;
#41860=DIRECTION ( 'NONE',  ( -3.491481338843132961E-15, -0.000000000000000000, 1.000000000000000000 ) ) ;
#41865=VERTEX_POINT ( 'NONE', #61038 ) ;
#41891=CARTESIAN_POINT ( 'NONE',  ( 0.4498537592782897998, 0.000000000000000000, -2.118110236220472675 ) ) ;
#41909=ORIENTED_EDGE ( 'NONE', *, *, #30007, .F. ) ;
#41912=CARTESIAN_POINT ( 'NONE',  ( 0.3149606299212184823, 2.165354330708661568, 3.924389226575471845 ) ) ;
#41917=DIRECTION ( 'NONE',  ( 0.000000000000000000, 1.408710688920637755E-15, -1.000000000000000000 ) ) ;
#41919=EDGE_CURVE ( 'NONE', #27207, #69303, #32558, .T. ) ;
#41932=CARTESIAN_POINT ( 'NONE',  ( 2.077234194078037000, 1.326002914239475805, -0.4256865378621398355 ) ) ;
#41956=FACE_OUTER_BOUND ( 'NONE', #6941, .T. ) ;
#41957=EDGE_CURVE ( 'NONE', #51378, #53614, #4664, .T. ) ;
#41961=CARTESIAN_POINT ( 'NONE',  ( -3.892860353355074299, 2.712196231959916659, 0.5314960629921260393 ) ) ;
#41971=LINE ( 'NONE', #62577, #74791 ) ;
#41992=CIRCLE ( 'NONE', #19156, 0.5118110236220471121 ) ;
#42000=CIRCLE ( 'NONE', #5705, 0.2165354330708659791 ) ;
#42010=CARTESIAN_POINT ( 'NONE',  ( -2.362204724409448620, 1.929133858267716661, -0.5118110236220719811 ) ) ;
#42018=PLANE ( 'NONE',  #74692 ) ;
#42024=CARTESIAN_POINT ( 'NONE',  ( 1.076935383196057527, 2.165354330708661568, 0.3149606299212600047 ) ) ;
#42025=EDGE_LOOP ( 'NONE', ( #48593, #29789, #20826, #57004 ) ) ;
#42052=CARTESIAN_POINT ( 'NONE',  ( -1.973869084197696910, 1.199841186584403863, -0.3336616047370135063 ) ) ;
#42058=VECTOR ( 'NONE', #40020, 39.37007874015748143 ) ;
#42072=CARTESIAN_POINT ( 'NONE',  ( 0.000000000000000000, 2.755905511811024056, 0.000000000000000000 ) ) ;
#42078=LINE ( 'NONE', #17666, #43413 ) ;
#42082=DIRECTION ( 'NONE',  ( 0.000000000000000000, -1.000000000000000000, 0.000000000000000000 ) ) ;
#42095=VERTEX_POINT ( 'NONE', #55587 ) ;
#42158=B_SPLINE_CURVE_WITH_KNOTS ( 'NONE', 3,
 ( #63449, #81178, #49987, #42843 ),
 .UNSPECIFIED., .F., .F.,
 ( 4, 4 ),
 ( 0.1666213495636641451, 0.1680035684901380333 ),
 .UNSPECIFIED. ) ;
#42170=CARTESIAN_POINT ( 'NONE',  ( 0.4744094488188900782, 1.537401574803149984, 2.170146923806596906 ) ) ;
#42174=CIRCLE ( 'NONE', #24679, 0.09842519685039351207 ) ;
#42189=ORIENTED_EDGE ( 'NONE', *, *, #52769, .F. ) ;
#42194=CARTESIAN_POINT ( 'NONE',  ( -0.03443470937339725840, 0.2755905511811023723, -1.320480459168889897 ) ) ;
#42203=EDGE_CURVE ( 'NONE', #80344, #23166, #17126, .T. ) ;
#42206=CARTESIAN_POINT ( 'NONE',  ( 0.000000000000000000, 2.677165354330708791, 0.000000000000000000 ) ) ;
#42230=DIRECTION ( 'NONE',  ( 0.000000000000000000, -1.000000000000000000, 0.000000000000000000 ) ) ;
#42238=CARTESIAN_POINT ( 'NONE',  ( -1.030578161883458410, 1.368986870467494565, 0.4437799316085911383 ) ) ;
#42252=CARTESIAN_POINT ( 'NONE',  ( 2.565525098582239316, 1.606100245667704929, -0.4697171261335975623 ) ) ;
#42259=DIRECTION ( 'NONE',  ( 0.000000000000000000, 0.000000000000000000, 1.000000000000000000 ) ) ;
#42276=VERTEX_POINT ( 'NONE', #63155 ) ;
#42287=AXIS2_PLACEMENT_3D ( 'NONE', #50571, #5558, #19011 ) ;
#42320=EDGE_LOOP ( 'NONE', ( #28967, #3805, #11360, #34741 ) ) ;
#42321=CARTESIAN_POINT ( 'NONE',  ( 0.4177787735907000366, 0.3937007874015748254, -1.874132239285499324 ) ) ;
#42325=LINE ( 'NONE', #4860, #15512 ) ;
#42326=PLANE ( 'NONE',  #28839 ) ;
#42337=EDGE_CURVE ( 'NONE', #312, #41865, #46353, .T. ) ;
#42339=CARTESIAN_POINT ( 'NONE',  ( -1.813482582612293559, 2.755905511811024056, 0.5314960629921260393 ) ) ;
#42342=ADVANCED_FACE ( 'NONE', ( #17733 ), #56003, .F. ) ;
#42365=CARTESIAN_POINT ( 'NONE',  ( 0.5314960629921156032, 2.755905511811024056, 0.9881811337016697117 ) ) ;
#42374=DIRECTION ( 'NONE',  ( 0.000000000000000000, 0.000000000000000000, -1.000000000000000000 ) ) ;
#42379=LINE ( 'NONE', #49107, #68059 ) ;
#42387=DIRECTION ( 'NONE',  ( -1.000000000000000000, -0.000000000000000000, -0.000000000000000000 ) ) ;
#42398=ORIENTED_EDGE ( 'NONE', *, *, #55727, .F. ) ;
#42409=EDGE_CURVE ( 'NONE', #19971, #26979, #16273, .T. ) ;
#42413=ORIENTED_EDGE ( 'NONE', *, *, #37207, .F. ) ;
#42431=CARTESIAN_POINT ( 'NONE',  ( 0.5314960629920997270, 2.755905511811024056, 2.503252890251021601 ) ) ;
#42444=AXIS2_PLACEMENT_3D ( 'NONE', #49288, #74991, #68660 ) ;
#42459=CIRCLE ( 'NONE', #80109, 3.228346456692913424 ) ;
#42460=CARTESIAN_POINT ( 'NONE',  ( -1.867828664896301616, 1.081851677178498949, 0.1334749385307871794 ) ) ;
#42480=EDGE_CURVE ( 'NONE', #35701, #10674, #19786, .T. ) ;
#42491=DIRECTION ( 'NONE',  ( 0.000000000000000000, 1.000000000000000000, 0.000000000000000000 ) ) ;
#42494=CARTESIAN_POINT ( 'NONE',  ( 3.908320185825791881, 1.537401574803149984, -0.4744094488188970171 ) ) ;
#42495=CIRCLE ( 'NONE', #822, 1.122047244094488194 ) ;
#42496=CONICAL_SURFACE ( 'NONE', #77419, 0.1771653543307085410, 1.029744258676653645 ) ;
#42497=AXIS2_PLACEMENT_3D ( 'NONE', #26352, #70136, #37335 ) ;
#42501=VERTEX_POINT ( 'NONE', #71552 ) ;
#42510=CYLINDRICAL_SURFACE ( 'NONE', #60174, 1.122047244094488194 ) ;
#42551=CARTESIAN_POINT ( 'NONE',  ( 2.583694225513480713, 2.755905511811024056, 0.5314960629921260393 ) ) ;
#42557=CARTESIAN_POINT ( 'NONE',  ( -2.647193076292303715, 1.325969025732688600, 0.4256800600601930440 ) ) ;
#42560=CARTESIAN_POINT ( 'NONE',  ( -0.1109416432469456093, 1.076146463964301692, -1.548361104749216510 ) ) ;
#42563=CIRCLE ( 'NONE', #13011, 1.122047244094488194 ) ;
#42565=AXIS2_PLACEMENT_3D ( 'NONE', #35657, #61320, #23021 ) ;
#42566=AXIS2_PLACEMENT_3D ( 'NONE', #30510, #37641, #24187 ) ;
#42581=DIRECTION ( 'NONE',  ( 0.000000000000000000, 1.000000000000000000, 0.000000000000000000 ) ) ;
#42584=EDGE_CURVE ( 'NONE', #32057, #12593, #20627, .T. ) ;
#42593=CARTESIAN_POINT ( 'NONE',  ( -1.736178228450298011, 1.299212598425196985, 0.4102808022082834460 ) ) ;
#42595=CARTESIAN_POINT ( 'NONE',  ( 2.112686649479616374, 1.697109554835843914, -0.4469779880792056348 ) ) ;
#42618=CARTESIAN_POINT ( 'NONE',  ( 0.000000000000000000, 1.929133858267716661, -2.874015748031495843 ) ) ;
#42622=AXIS2_PLACEMENT_3D ( 'NONE', #81714, #50506, #11412 ) ;
#42641=FACE_OUTER_BOUND ( 'NONE', #22102, .T. ) ;
#42660=DIRECTION ( 'NONE',  ( 0.000000000000000000, 0.000000000000000000, -1.000000000000000000 ) ) ;
#42689=CARTESIAN_POINT ( 'NONE',  ( 0.3634034883589535303, 1.231066118352841521, 2.000797776986567467 ) ) ;
#42693=VERTEX_POINT ( 'NONE', #6733 ) ;
#42697=CARTESIAN_POINT ( 'NONE',  ( -2.103514684734978601, 1.710972922415816999, -0.4417590601942929518 ) ) ;
#42732=EDGE_LOOP ( 'NONE', ( #81892, #83, #18514 ) ) ;
#42734=ORIENTED_EDGE ( 'NONE', *, *, #75585, .F. ) ;
#42735=LINE ( 'NONE', #42321, #75816 ) ;
#42738=CARTESIAN_POINT ( 'NONE',  ( -3.886287458032462006, 2.755905511811024056, -0.6299212598425202314 ) ) ;
#42739=DIRECTION ( 'NONE',  ( -3.491481338843132961E-15, -0.000000000000000000, 1.000000000000000000 ) ) ;
#42741=DIRECTION ( 'NONE',  ( 0.000000000000000000, 0.000000000000000000, 1.000000000000000000 ) ) ;
#42784=EDGE_LOOP ( 'NONE', ( #45674, #31022, #5284, #60240 ) ) ;
#42797=EDGE_CURVE ( 'NONE', #4140, #82716, #58919, .T. ) ;
#42839=DIRECTION ( 'NONE',  ( -0.000000000000000000, 1.000000000000000000, -0.000000000000000000 ) ) ;
#42843=CARTESIAN_POINT ( 'NONE',  ( -0.5314960629921169355, 2.755905511811024056, -2.583694225513482490 ) ) ;
#42844=ORIENTED_EDGE ( 'NONE', *, *, #1933, .T. ) ;
#42846=CARTESIAN_POINT ( 'NONE',  ( 1.141392835773559211, 0.4110443821404751730, 0.9642274814428540841 ) ) ;
#42850=CARTESIAN_POINT ( 'NONE',  ( -0.4256212168908878879, 1.327274814196968133, 3.913940744879238487 ) ) ;
#42868=CARTESIAN_POINT ( 'NONE',  ( -2.131054703900732150, 1.408268389154270883, 0.4567427728026676181 ) ) ;
#42873=CARTESIAN_POINT ( 'NONE',  ( 3.937007874015748143, 2.559055118110236560, -0.3149606299212596716 ) ) ;
#42877=CARTESIAN_POINT ( 'NONE',  ( 1.141392835773559211, 1.299212598425196985, 1.318558190104271333 ) ) ;
#42886=CARTESIAN_POINT ( 'NONE',  ( 0.5314960629920993940, 2.716535433070866645, 2.543486866223394482 ) ) ;
#42894=EDGE_CURVE ( 'NONE', #65196, #15966, #58142, .T. ) ;
#42899=CYLINDRICAL_SURFACE ( 'NONE', #25667, 0.4744094488188972947 ) ;
#42902=DIRECTION ( 'NONE',  ( -0.000000000000000000, 1.000000000000000000, -0.000000000000000000 ) ) ;
#42906=ORIENTED_EDGE ( 'NONE', *, *, #41175, .T. ) ;
#42909=ORIENTED_EDGE ( 'NONE', *, *, #80976, .F. ) ;
#42926=ORIENTED_EDGE ( 'NONE', *, *, #16862, .F. ) ;
#42955=CARTESIAN_POINT ( 'NONE',  ( 1.348312163386739426, 0.2929341459200028863, 0.6402614161801758463 ) ) ;
#42960=CARTESIAN_POINT ( 'NONE',  ( 0.4735649329124898554, 1.569965579892641960, -1.017216587056824162 ) ) ;
#42963=CARTESIAN_POINT ( 'NONE',  ( -2.867261597185507327, 1.070284760220065579, -0.08454815954496505692 ) ) ;
#42966=CARTESIAN_POINT ( 'NONE',  ( -0.1021718162100117705, 1.074111179983719744, -1.580847797370428687 ) ) ;
#42974=CARTESIAN_POINT ( 'NONE',  ( 0.06247320855440641890, 1.066079912482593262, -1.120731204487458665 ) ) ;
#42979=CARTESIAN_POINT ( 'NONE',  ( 0.06838555148300280717, 1.067631514832606543, -1.854691556240662731 ) ) ;
#42997=CARTESIAN_POINT ( 'NONE',  ( -1.710644741211760467, 1.192425108176624615, 0.3257230034225878645 ) ) ;
#42998=DIRECTION ( 'NONE',  ( 0.000000000000000000, 0.000000000000000000, 1.000000000000000000 ) ) ;
#43005=VERTEX_POINT ( 'NONE', #37198 ) ;
#43010=CARTESIAN_POINT ( 'NONE',  ( 2.154527559055117170, 0.03937007874015747977, 0.4677827689124997024 ) ) ;
#43015=B_SPLINE_CURVE_WITH_KNOTS ( 'NONE', 3,
 ( #44718, #64111, #43489, #12355, #75515, #62452, #49815, #6028, #50225, #38012, #82644, #4788 ),
 .UNSPECIFIED., .F., .F.,
 ( 4, 2, 2, 2, 2, 4 ),
 ( 0.05454303362711803577, 0.05585633982237159234, 0.05651299291999837410, 0.05716964601762515585, 0.05848295221287872631, 0.05979625840813228982 ),
 .UNSPECIFIED. ) ;
#43041=ORIENTED_EDGE ( 'NONE', *, *, #61425, .T. ) ;
#43070=CARTESIAN_POINT ( 'NONE',  ( 0.000000000000000000, 0.03937007874015747977, 0.000000000000000000 ) ) ;
#43078=DIRECTION ( 'NONE',  ( -0.000000000000000000, -1.000000000000000000, -0.000000000000000000 ) ) ;
#43094=CONICAL_SURFACE ( 'NONE', #53855, 0.1771653543307085410, 1.029744258676653645 ) ;
#43131=VECTOR ( 'NONE', #81075, 39.37007874015748143 ) ;
#43138=ORIENTED_EDGE ( 'NONE', *, *, #64406, .T. ) ;
#43141=DIRECTION ( 'NONE',  ( -0.000000000000000000, -1.000000000000000000, -0.000000000000000000 ) ) ;
#43146=DIRECTION ( 'NONE',  ( 0.000000000000000000, 1.734723475976808327E-16, -1.000000000000000000 ) ) ;
#43153=CIRCLE ( 'NONE', #69372, 3.267716535433071279 ) ;
#43157=CARTESIAN_POINT ( 'NONE',  ( -0.4677827689124922084, 0.03937007874015747977, -2.154527559055118946 ) ) ;
#43163=CARTESIAN_POINT ( 'NONE',  ( 0.5314960629921063884, 2.729653127095272414, 1.868118615532837756 ) ) ;
#43188=ORIENTED_EDGE ( 'NONE', *, *, #14047, .T. ) ;
#43215=ORIENTED_EDGE ( 'NONE', *, *, #33608, .F. ) ;
#43225=EDGE_CURVE ( 'NONE', #1055, #26552, #56135, .T. ) ;
#43237=CYLINDRICAL_SURFACE ( 'NONE', #76736, 0.5118110236220471121 ) ;
#43238=CARTESIAN_POINT ( 'NONE',  ( -1.313877454013331780, 0.2755905511811023723, 0.6999040823587869831 ) ) ;
#43248=EDGE_LOOP ( 'NONE', ( #31543, #60116, #63238, #18682 ) ) ;
#43250=CIRCLE ( 'NONE', #6971, 3.858267716535433323 ) ;
#43255=CARTESIAN_POINT ( 'NONE',  ( 4.821444151489972621E-16, 1.062992125984252745, 3.937007874015748143 ) ) ;
#43269=EDGE_CURVE ( 'NONE', #31620, #45375, #17041, .T. ) ;
#43274=CARTESIAN_POINT ( 'NONE',  ( 0.000000000000000000, 0.07874015748031502893, 0.000000000000000000 ) ) ;
#43293=DIRECTION ( 'NONE',  ( -0.000000000000000000, -1.000000000000000000, -0.000000000000000000 ) ) ;
#43304=DIRECTION ( 'NONE',  ( 0.000000000000000000, 0.000000000000000000, 1.000000000000000000 ) ) ;
#43307=CARTESIAN_POINT ( 'NONE',  ( -1.313877454013331780, 0.2755905511811023723, 0.9174237673981568975 ) ) ;
#43311=ORIENTED_EDGE ( 'NONE', *, *, #53064, .T. ) ;
#43314=ORIENTED_EDGE ( 'NONE', *, *, #75903, .T. ) ;
#43323=CARTESIAN_POINT ( 'NONE',  ( 0.4252607725274244466, 1.326635381343778120, -2.647232528933507467 ) ) ;
#43329=ORIENTED_EDGE ( 'NONE', *, *, #72867, .T. ) ;
#43358=CARTESIAN_POINT ( 'NONE',  ( 0.9285414500055708675, 1.724409448818898127, 0.6299212598425202314 ) ) ;
#43365=CARTESIAN_POINT ( 'NONE',  ( -2.619388402063342891, 1.366082762360727454, 0.4426340671871359933 ) ) ;
#43379=CARTESIAN_POINT ( 'NONE',  ( 0.4744094488189011805, 1.537401574803149984, -1.016821367227981998 ) ) ;
#43384=CARTESIAN_POINT ( 'NONE',  ( 0.4258029703577317915, 1.326239216270299393, -2.077409958192426132 ) ) ;
#43390=CARTESIAN_POINT ( 'NONE',  ( 1.881759016064405099, 2.742776604255995565, -0.5314960629921260393 ) ) ;
#43411=ORIENTED_EDGE ( 'NONE', *, *, #51390, .T. ) ;
#43413=VECTOR ( 'NONE', #80821, 39.37007874015748143 ) ;
#43429=CARTESIAN_POINT ( 'NONE',  ( -0.01706770257043029385, 1.062992125984252967, -1.850393700787401619 ) ) ;
#43445=CARTESIAN_POINT ( 'NONE',  ( 3.909109051758220321, 1.617477308826748228, -0.4678760369123936003 ) ) ;
#43446=EDGE_CURVE ( 'NONE', #21338, #55552, #51045, .T. ) ;
#43450=VERTEX_POINT ( 'NONE', #18671 ) ;
#43453=CARTESIAN_POINT ( 'NONE',  ( -1.033875059083676939, 1.724409448818897905, 0.4359958488159718093 ) ) ;
#43474=CARTESIAN_POINT ( 'NONE',  ( 0.5314960629920921775, 2.716535433070866645, 3.224202737261820939 ) ) ;
#43489=CARTESIAN_POINT ( 'NONE',  ( 2.556694656352263006, 1.572145545125845922, 0.4734416007054421116 ) ) ;
#43501=LINE ( 'NONE', #25805, #78419 ) ;
#43509=CARTESIAN_POINT ( 'NONE',  ( -2.152711368484068188, 1.622209144264166847, -0.4670403427556032994 ) ) ;
#43520=AXIS2_PLACEMENT_3D ( 'NONE', #59099, #57832, #70060 ) ;
#43535=CIRCLE ( 'NONE', #54305, 0.5118110236220471121 ) ;
#43553=DIRECTION ( 'NONE',  ( 0.000000000000000000, 0.000000000000000000, 1.000000000000000000 ) ) ;
#43557=CARTESIAN_POINT ( 'NONE',  ( -0.5314960629921323676, 2.729664787007372695, 1.840814861705235783 ) ) ;
#43558=DIRECTION ( 'NONE',  ( 0.000000000000000000, -1.000000000000000000, 0.000000000000000000 ) ) ;
#43559=CARTESIAN_POINT ( 'NONE',  ( 0.000000000000000000, 2.716535433070866645, 0.000000000000000000 ) ) ;
#43570=LINE ( 'NONE', #69271, #3546 ) ;
#43575=DIRECTION ( 'NONE',  ( -1.408710688920637755E-15, 1.000000000000000000, -4.918487082195260922E-30 ) ) ;
#43582=CIRCLE ( 'NONE', #14058, 0.3149606299212597271 ) ;
#43601=VERTEX_POINT ( 'NONE', #49655 ) ;
#43614=CARTESIAN_POINT ( 'NONE',  ( 0.2405914015988345200, 1.128524939042355069, -1.573041762559489687 ) ) ;
#43626=EDGE_LOOP ( 'NONE', ( #16681, #41506, #57184, #37740, #1124, #65059, #10125 ) ) ;
#43641=VERTEX_POINT ( 'NONE', #5050 ) ;
#43650=CIRCLE ( 'NONE', #10108, 3.858267716535433323 ) ;
#43660=CARTESIAN_POINT ( 'NONE',  ( 0.000000000000000000, 2.755905511811024056, 0.000000000000000000 ) ) ;
#43661=EDGE_LOOP ( 'NONE', ( #9835, #5559, #44801, #11696 ) ) ;
#43663=PLANE ( 'NONE',  #47578 ) ;
#43682=CARTESIAN_POINT ( 'NONE',  ( -0.9881811337016640495, 2.559055118110236560, 0.5314960629921260393 ) ) ;
#43689=LINE ( 'NONE', #50424, #46521 ) ;
#43705=CARTESIAN_POINT ( 'NONE',  ( -3.911274423169837089, 1.384680224527505166, 0.4494265461045906518 ) ) ;
#43709=CARTESIAN_POINT ( 'NONE',  ( -3.250800430253136586, 2.742781091603911925, 0.5314960629921260393 ) ) ;
#43710=EDGE_CURVE ( 'NONE', #17817, #57422, #31293, .T. ) ;
#43720=FACE_OUTER_BOUND ( 'NONE', #71504, .T. ) ;
#43732=FACE_OUTER_BOUND ( 'NONE', #75476, .T. ) ;
#43760=VECTOR ( 'NONE', #27948, 39.37007874015748143 ) ;
#43770=DIRECTION ( 'NONE',  ( 0.000000000000000000, 0.000000000000000000, 1.000000000000000000 ) ) ;
#43776=CARTESIAN_POINT ( 'NONE',  ( -2.872342878167415403, 1.064797240280314083, -0.04222672046125293399 ) ) ;
#43792=LINE ( 'NONE', #62774, #80056 ) ;
#43797=AXIS2_PLACEMENT_3D ( 'NONE', #72599, #71347, #14945 ) ;
#43799=CARTESIAN_POINT ( 'NONE',  ( -0.4744094488188833059, 1.537401574803149984, -3.908320185825793658 ) ) ;
#43811=DIRECTION ( 'NONE',  ( -0.000000000000000000, -1.000000000000000000, -0.000000000000000000 ) ) ;
#43816=CIRCLE ( 'NONE', #38490, 3.444881889763779625 ) ;
#43838=CARTESIAN_POINT ( 'NONE',  ( -0.03443470937339728616, 1.062992125984252079, -1.537015892239756099 ) ) ;
#43839=CARTESIAN_POINT ( 'NONE',  ( 4.725015209308685971E-16, 0.07874015748031502893, -3.858267716535433323 ) ) ;
#43840=ORIENTED_EDGE ( 'NONE', *, *, #29666, .T. ) ;
#43858=ORIENTED_EDGE ( 'NONE', *, *, #46418, .T. ) ;
#43861=AXIS2_PLACEMENT_3D ( 'NONE', #5600, #58180, #62857 ) ;
#43865=AXIS2_PLACEMENT_3D ( 'NONE', #59114, #59527, #20822 ) ;
#43869=DIRECTION ( 'NONE',  ( 0.000000000000000000, 0.000000000000000000, 1.000000000000000000 ) ) ;
#43870=CARTESIAN_POINT ( 'NONE',  ( 0.4177787735907000366, 0.000000000000000000, -1.559171609364239375 ) ) ;
#43886=AXIS2_PLACEMENT_3D ( 'NONE', #15348, #28372, #79326 ) ;
#43894=CARTESIAN_POINT ( 'NONE',  ( 0.000000000000000000, 2.716535433070866645, 0.000000000000000000 ) ) ;
#43908=CARTESIAN_POINT ( 'NONE',  ( -0.5314960629921224866, 0.000000000000000000, -0.9881811337016660479 ) ) ;
#43930=CONICAL_SURFACE ( 'NONE', #7678, 0.09842519685039351207, 1.029744258676651647 ) ;
#43936=CARTESIAN_POINT ( 'NONE',  ( -0.3132167369146011682, 1.180756483954326752, 1.077514311222549814 ) ) ;
#43937=CARTESIAN_POINT ( 'NONE',  ( 3.908320185825791881, 1.569734778958133514, 0.4744094488188976277 ) ) ;
#43953=CARTESIAN_POINT ( 'NONE',  ( -0.3149606299212458493, 2.165354330708661568, -3.937007874015763242 ) ) ;
#43965=VERTEX_POINT ( 'NONE', #55792 ) ;
#43972=DIRECTION ( 'NONE',  ( -3.491481338843132961E-15, -0.000000000000000000, 1.000000000000000000 ) ) ;
#43981=CARTESIAN_POINT ( 'NONE',  ( 0.5314960629921156032, 2.559055118110236560, 0.9881811337016696006 ) ) ;
#43993=EDGE_CURVE ( 'NONE', #38787, #36842, #63502, .T. ) ;
#43999=ADVANCED_FACE ( 'NONE', ( #66800, #2816 ), #22168, .T. ) ;
#44018=VERTEX_POINT ( 'NONE', #42339 ) ;
#44032=CARTESIAN_POINT ( 'NONE',  ( 0.000000000000000000, 0.4374015748031496176, 0.000000000000000000 ) ) ;
#44043=VECTOR ( 'NONE', #53864, 39.37007874015748143 ) ;
#44044=LINE ( 'NONE', #69736, #66742 ) ;
#44067=FACE_OUTER_BOUND ( 'NONE', #38790, .T. ) ;
#44069=B_SPLINE_CURVE_WITH_KNOTS ( 'NONE', 3,
 ( #14677, #40333, #79073, #34018, #59678, #21389, #71490, #72737, #60102, #15501, #2034, #47458, #28114, #27699, #8761, #21795 ),
 .UNSPECIFIED., .F., .F.,
 ( 4, 2, 2, 2, 2, 2, 2, 4 ),
 ( 0.000000000000000000, 0.0003923911760484627724, 0.0007847823520969255447, 0.001177173528145388209, 0.001569564704193851089, 0.001961955880242313970, 0.002354347056290776417, 0.003139129408387686133 ),
 .UNSPECIFIED. ) ;
#44086=CARTESIAN_POINT ( 'NONE',  ( -0.5314960629921122726, 2.755905511811024056, -3.937007874015763687 ) ) ;
#44105=CARTESIAN_POINT ( 'NONE',  ( 0.5314960629920993940, 2.716535433070866645, 2.543486866223394482 ) ) ;
#44123=CARTESIAN_POINT ( 'NONE',  ( -3.920805145893436539, 1.223994253877878302, -0.3574943889377464323 ) ) ;
#44127=CARTESIAN_POINT ( 'NONE',  ( -0.4359958488159755841, 1.724409448818897905, 1.033875059083675163 ) ) ;
#44129=ORIENTED_EDGE ( 'NONE', *, *, #42894, .T. ) ;
#44135=CARTESIAN_POINT ( 'NONE',  ( 3.937007874015748143, 1.537401574803149984, 2.901595197523589142E-16 ) ) ;
#44144=ORIENTED_EDGE ( 'NONE', *, *, #49461, .F. ) ;
#44178=EDGE_CURVE ( 'NONE', #55060, #26586, #24569, .T. ) ;
#44194=CARTESIAN_POINT ( 'NONE',  ( -2.873989802184792719, 1.063020117359138705, 0.01785754392583522449 ) ) ;
#44206=DIRECTION ( 'NONE',  ( -3.491481338843133355E-15, -0.000000000000000000, 1.000000000000000000 ) ) ;
#44214=CARTESIAN_POINT ( 'NONE',  ( 1.868118615532832649, 2.729653127095272414, -0.5314960629921260393 ) ) ;
#44227=FACE_OUTER_BOUND ( 'NONE', #76300, .T. ) ;
#44231=PLANE ( 'NONE',  #44825 ) ;
#44236=EDGE_LOOP ( 'NONE', ( #65340, #22729, #56790, #72850 ) ) ;
#44243=CYLINDRICAL_SURFACE ( 'NONE', #45366, 0.4744094488188972947 ) ;
#44252=CARTESIAN_POINT ( 'NONE',  ( -0.2516118885077178735, 1.134065313995066493, -1.915546005056554035 ) ) ;
#44256=ORIENTED_EDGE ( 'NONE', *, *, #80061, .F. ) ;
#44268=DIRECTION ( 'NONE',  ( 0.000000000000000000, 1.000000000000000000, -0.000000000000000000 ) ) ;
#44301=DIRECTION ( 'NONE',  ( -3.491481338843132961E-15, -0.000000000000000000, 1.000000000000000000 ) ) ;
#44381=ORIENTED_EDGE ( 'NONE', *, *, #58316, .F. ) ;
#44384=FACE_OUTER_BOUND ( 'NONE', #18916, .T. ) ;
#44389=ORIENTED_EDGE ( 'NONE', *, *, #22408, .T. ) ;
#44416=ORIENTED_EDGE ( 'NONE', *, *, #75806, .F. ) ;
#44434=VECTOR ( 'NONE', #69354, 39.37007874015748143 ) ;
#44436=CARTESIAN_POINT ( 'NONE',  ( 0.3149606299212482918, 2.165354330708661568, 1.076935383196061080 ) ) ;
#44444=ADVANCED_FACE ( 'NONE', ( #17932 ), #55439, .F. ) ;
#44453=EDGE_CURVE ( 'NONE', #40881, #19658, #41992, .T. ) ;
#44461=ORIENTED_EDGE ( 'NONE', *, *, #21276, .F. ) ;
#44463=EDGE_LOOP ( 'NONE', ( #13326, #22333 ) ) ;
#44473=DIRECTION ( 'NONE',  ( -1.000000000000000000, -1.734723475976808080E-16, -3.491481338843132961E-15 ) ) ;
#44532=DIRECTION ( 'NONE',  ( 0.000000000000000000, 0.000000000000000000, -1.000000000000000000 ) ) ;
#44534=VERTEX_POINT ( 'NONE', #43981 ) ;
#44546=ADVANCED_FACE ( 'NONE', ( #69678 ), #31357, .F. ) ;
#44548=VERTEX_POINT ( 'NONE', #43157 ) ;
#44550=VERTEX_POINT ( 'NONE', #5688 ) ;
#44558=CIRCLE ( 'NONE', #67258, 1.122047244094488194 ) ;
#44568=CARTESIAN_POINT ( 'NONE',  ( 2.666386537446502558, 1.301102360844750727, -0.4123394245947693548 ) ) ;
#44598=CARTESIAN_POINT ( 'NONE',  ( 0.4359958488159859091, 1.724409448818897905, -3.912791665790197992 ) ) ;
#44611=CARTESIAN_POINT ( 'NONE',  ( 0.1239563933494705478, 1.079204589967275085, -1.115281408855063550 ) ) ;
#44613=AXIS2_PLACEMENT_3D ( 'NONE', #7703, #27041, #21562 ) ;
#44615=CARTESIAN_POINT ( 'NONE',  ( 0.4477123500622125496, 1.379796003448449326, -2.114018334261799303 ) ) ;
#44621=DIRECTION ( 'NONE',  ( -0.000000000000000000, -1.000000000000000000, -0.000000000000000000 ) ) ;
#44638=DIRECTION ( 'NONE',  ( 1.000000000000000000, 0.000000000000000000, -0.000000000000000000 ) ) ;
#44641=EDGE_CURVE ( 'NONE', #7205, #9834, #82717, .T. ) ;
#44643=ORIENTED_EDGE ( 'NONE', *, *, #63199, .F. ) ;
#44648=CARTESIAN_POINT ( 'NONE',  ( -0.03443470937339725840, 0.000000000000000000, -1.320480459168889897 ) ) ;
#44659=PLANE ( 'NONE',  #42287 ) ;
#44660=ORIENTED_EDGE ( 'NONE', *, *, #24957, .T. ) ;
#44663=EDGE_LOOP ( 'NONE', ( #66979, #17991, #31393, #8677 ) ) ;
#44676=CARTESIAN_POINT ( 'NONE',  ( 3.908813327757459266, 1.601535082192234727, -0.4703318888109126461 ) ) ;
#44679=ORIENTED_EDGE ( 'NONE', *, *, #41491, .F. ) ;
#44718=CARTESIAN_POINT ( 'NONE',  ( 2.554262525012302110, 1.537401574803149984, 0.4744094488188975722 ) ) ;
#44729=VECTOR ( 'NONE', #57683, 39.37007874015748143 ) ;
#44736=ADVANCED_FACE ( 'NONE', ( #76409 ), #5287, .T. ) ;
#44748=DIRECTION ( 'NONE',  ( 0.000000000000000000, 1.000000000000000000, 0.000000000000000000 ) ) ;
#44783=CARTESIAN_POINT ( 'NONE',  ( -0.4606976121171968419, 1.423084236280317993, 2.585293067984823612 ) ) ;
#44786=CIRCLE ( 'NONE', #34077, 3.267716535433071279 ) ;
#44792=VERTEX_POINT ( 'NONE', #56615 ) ;
#44793=DIRECTION ( 'NONE',  ( 0.000000000000000000, 0.000000000000000000, 1.000000000000000000 ) ) ;
#44798=B_SPLINE_CURVE_WITH_KNOTS ( 'NONE', 3,
 ( #42551, #67419, #68254, #72899 ),
 .UNSPECIFIED., .F., .F.,
 ( 4, 4 ),
 ( 0.07610408314619493408, 0.07753336624204351657 ),
 .UNSPECIFIED. ) ;
#44801=ORIENTED_EDGE ( 'NONE', *, *, #70218, .F. ) ;
#44825=AXIS2_PLACEMENT_3D ( 'NONE', #18990, #50960, #44638 ) ;
#44828=VERTEX_POINT ( 'NONE', #38087 ) ;
#44843=CARTESIAN_POINT ( 'NONE',  ( 0.4741686481756308691, 1.554815631980118740, 2.554860351194805368 ) ) ;
#44847=LINE ( 'NONE', #76050, #5129 ) ;
#44854=DIRECTION ( 'NONE',  ( -0.000000000000000000, -1.000000000000000000, -0.000000000000000000 ) ) ;
#44862=CARTESIAN_POINT ( 'NONE',  ( 0.000000000000000000, 2.755905511811024056, 0.000000000000000000 ) ) ;
#44880=CYLINDRICAL_SURFACE ( 'NONE', #49868, 0.5118110236220472231 ) ;
#44886=AXIS2_PLACEMENT_3D ( 'NONE', #25294, #38764, #31202 ) ;
#44898=CARTESIAN_POINT ( 'NONE',  ( -2.112686649479645684, 1.697109554835842804, 0.4469779880792058568 ) ) ;
#44899=EDGE_CURVE ( 'NONE', #79813, #82661, #1700, .T. ) ;
#44939=CARTESIAN_POINT ( 'NONE',  ( -1.559171609364246924, 0.3937007874015748254, 0.4177787735906735578 ) ) ;
#44948=AXIS2_PLACEMENT_3D ( 'NONE', #33032, #45645, #46481 ) ;
#44949=DIRECTION ( 'NONE',  ( 0.000000000000000000, 0.000000000000000000, -1.000000000000000000 ) ) ;
#44962=EDGE_LOOP ( 'NONE', ( #80346, #63110, #35394, #2167 ) ) ;
#44981=ORIENTED_EDGE ( 'NONE', *, *, #60079, .F. ) ;
#44985=CARTESIAN_POINT ( 'NONE',  ( -0.5314960629921395840, 2.677165354330708791, 3.900966923095588346 ) ) ;
#44991=CARTESIAN_POINT ( 'NONE',  ( 0.5314960629921348101, 2.729661042438510599, -2.530077748780001023 ) ) ;
#45017=LINE ( 'NONE', #77035, #23821 ) ;
#45026=EDGE_CURVE ( 'NONE', #69303, #49578, #26288, .T. ) ;
#45027=CIRCLE ( 'NONE', #30269, 2.637795275590551380 ) ;
#45032=CARTESIAN_POINT ( 'NONE',  ( 0.000000000000000000, 2.755905511811024056, 0.000000000000000000 ) ) ;
#45034=EDGE_CURVE ( 'NONE', #76998, #43965, #25879, .T. ) ;
#45047=CARTESIAN_POINT ( 'NONE',  ( -3.937007874015748143, 2.755905511811024056, -0.5314960629921260393 ) ) ;
#45055=DIRECTION ( 'NONE',  ( 0.000000000000000000, -0.000000000000000000, 1.000000000000000000 ) ) ;
#45063=ORIENTED_EDGE ( 'NONE', *, *, #40694, .T. ) ;
#45066=ORIENTED_EDGE ( 'NONE', *, *, #27285, .F. ) ;
#45080=CARTESIAN_POINT ( 'NONE',  ( -0.4744094488188891900, 1.520194873416442993, -2.170146923806593797 ) ) ;
#45097=B_SPLINE_CURVE_WITH_KNOTS ( 'NONE', 3,
 ( #68476, #17960, #49924, #29745, #81528, #41961, #49097, #10814, #74801, #11230, #54589, #62149, #17552, #11648 ),
 .UNSPECIFIED., .F., .F.,
 ( 4, 2, 2, 2, 2, 2, 4 ),
 ( 0.000000000000000000, 0.0003923887041693346835, 0.0007847774083386693670, 0.001177166112508004105, 0.001569554816677338734, 0.002354332225016037266, 0.003139109633354736015 ),
 .UNSPECIFIED. ) ;
#45099=FACE_BOUND ( 'NONE', #54099, .T. ) ;
#45100=VERTEX_POINT ( 'NONE', #59524 ) ;
#45126=CIRCLE ( 'NONE', #78762, 1.889763779527559251 ) ;
#45134=CARTESIAN_POINT ( 'NONE',  ( -0.4725026149319510593, 1.580736828574223596, 2.165487897237754034 ) ) ;
#45141=CARTESIAN_POINT ( 'NONE',  ( 1.102250182176885085, 1.111780926165008898, -0.2118791181513735022 ) ) ;
#45144=CIRCLE ( 'NONE', #16957, 0.2165354330708659791 ) ;
#45182=AXIS2_PLACEMENT_3D ( 'NONE', #49244, #55549, #36212 ) ;
#45200=ORIENTED_EDGE ( 'NONE', *, *, #61964, .T. ) ;
#45202=ORIENTED_EDGE ( 'NONE', *, *, #77795, .F. ) ;
#45209=CARTESIAN_POINT ( 'NONE',  ( -0.4744094488189058989, 1.537401574803149984, 2.554262525012261253 ) ) ;
#45218=CARTESIAN_POINT ( 'NONE',  ( -1.030590969126516265, 1.368909816122638512, -0.4437501211348749419 ) ) ;
#45228=DIRECTION ( 'NONE',  ( 0.000000000000000000, -1.000000000000000000, 0.000000000000000000 ) ) ;
#45247=AXIS2_PLACEMENT_3D ( 'NONE', #47508, #28985, #53816 ) ;
#45254=PLANE ( 'NONE',  #53318 ) ;
#45259=VERTEX_POINT ( 'NONE', #78496 ) ;
#45274=CARTESIAN_POINT ( 'NONE',  ( 0.3961547706187970030, 1.274880491790000292, -1.735579852066672979 ) ) ;
#45286=EDGE_LOOP ( 'NONE', ( #68113, #61059, #14144, #43858 ) ) ;
#45287=VERTEX_POINT ( 'NONE', #39755 ) ;
#45314=CARTESIAN_POINT ( 'NONE',  ( 0.4677827689124922084, 0.03937007874015747977, 2.154527559055118946 ) ) ;
#45328=CARTESIAN_POINT ( 'NONE',  ( -2.138346301250427572, 1.653225543546886778, 0.4603267246303517357 ) ) ;
#45341=CARTESIAN_POINT ( 'NONE',  ( -0.1091324866932888854, 1.075701271242782919, -1.559683122296843250 ) ) ;
#45351=CARTESIAN_POINT ( 'NONE',  ( 1.854472803289052507, 2.716535433070866645, 0.5314960629921260393 ) ) ;
#45359=CARTESIAN_POINT ( 'NONE',  ( 0.000000000000000000, 2.755905511811024056, 0.000000000000000000 ) ) ;
#45360=EDGE_CURVE ( 'NONE', #43601, #49366, #54398, .T. ) ;
#45366=AXIS2_PLACEMENT_3D ( 'NONE', #18194, #56881, #17784 ) ;
#45375=VERTEX_POINT ( 'NONE', #47722 ) ;
#45407=ORIENTED_EDGE ( 'NONE', *, *, #6791, .F. ) ;
#45409=CARTESIAN_POINT ( 'NONE',  ( 2.558820304884363406, 1.494558157769223961, -0.4725443725032419939 ) ) ;
#45420=CARTESIAN_POINT ( 'NONE',  ( -2.571698080334722025, 1.622209144264171066, 0.4670403427556019671 ) ) ;
#45438=CARTESIAN_POINT ( 'NONE',  ( -1.076935383196057305, 5.463695987328539379E-17, -0.3149606299212603933 ) ) ;
#45455=CARTESIAN_POINT ( 'NONE',  ( 0.000000000000000000, 2.165354330708661568, 0.000000000000000000 ) ) ;
#45459=CARTESIAN_POINT ( 'NONE',  ( 0.01707598052245543063, 1.062992125984252745, -1.850393700787402729 ) ) ;
#45478=DIRECTION ( 'NONE',  ( -0.000000000000000000, -1.000000000000000000, -0.000000000000000000 ) ) ;
#45479=DIRECTION ( 'NONE',  ( 0.000000000000000000, 0.000000000000000000, 1.000000000000000000 ) ) ;
#45487=ORIENTED_EDGE ( 'NONE', *, *, #55596, .T. ) ;
#45523=CARTESIAN_POINT ( 'NONE',  ( 1.141392835773559211, 0.4110443821404751730, 1.318558190104271333 ) ) ;
#45527=ORIENTED_EDGE ( 'NONE', *, *, #3893, .T. ) ;
#45547=ADVANCED_FACE ( 'NONE', ( #14563 ), #72620, .T. ) ;
#45552=CARTESIAN_POINT ( 'NONE',  ( 0.5314960629920926216, 2.755905511811024056, 3.184294706754636106 ) ) ;
#45603=CARTESIAN_POINT ( 'NONE',  ( -0.4744094488188895231, 1.546135192374304745, -2.170146923806595574 ) ) ;
#45608=EDGE_CURVE ( 'NONE', #9070, #7002, #29244, .T. ) ;
#45622=ORIENTED_EDGE ( 'NONE', *, *, #48595, .T. ) ;
#45627=FACE_OUTER_BOUND ( 'NONE', #28740, .T. ) ;
#45628=CARTESIAN_POINT ( 'NONE',  ( -0.3013144171194466203, 1.169708940200700820, 2.776959576054383927 ) ) ;
#45633=CYLINDRICAL_SURFACE ( 'NONE', #4953, 0.3149606299212598381 ) ;
#45636=ORIENTED_EDGE ( 'NONE', *, *, #6668, .T. ) ;
#45644=EDGE_LOOP ( 'NONE', ( #5461, #47919, #6555, #63634 ) ) ;
#45645=DIRECTION ( 'NONE',  ( 0.000000000000000000, -1.000000000000000000, -0.000000000000000000 ) ) ;
#45646=DIRECTION ( 'NONE',  ( -8.673617379884022653E-16, 1.000000000000000000, -3.028377322213053966E-30 ) ) ;
#45652=FACE_OUTER_BOUND ( 'NONE', #67175, .T. ) ;
#45674=ORIENTED_EDGE ( 'NONE', *, *, #83038, .T. ) ;
#45702=EDGE_CURVE ( 'NONE', #74865, #41210, #61223, .T. ) ;
#45703=ORIENTED_EDGE ( 'NONE', *, *, #26367, .T. ) ;
#45731=CARTESIAN_POINT ( 'NONE',  ( -0.02863813702883717324, 1.063821633877343631, -1.439971228356280220 ) ) ;
#45737=ORIENTED_EDGE ( 'NONE', *, *, #35750, .F. ) ;
#45745=CARTESIAN_POINT ( 'NONE',  ( -0.4705803914132928312, 1.475246498736264344, 3.908783377261402681 ) ) ;
#45768=LINE ( 'NONE', #58407, #16999 ) ;
#45774=DIRECTION ( 'NONE',  ( 0.000000000000000000, 1.000000000000000000, -0.000000000000000000 ) ) ;
#45786=CARTESIAN_POINT ( 'NONE',  ( 0.4498537592782897998, 0.000000000000000000, 2.118110236220472675 ) ) ;
#45791=AXIS2_PLACEMENT_3D ( 'NONE', #74926, #34958, #74094 ) ;
#45798=EDGE_CURVE ( 'NONE', #11714, #44018, #13113, .T. ) ;
#45801=CARTESIAN_POINT ( 'NONE',  ( 5.818687728935708833E-24, 1.062992125984252745, -3.937007874015748143 ) ) ;
#45807=VERTEX_POINT ( 'NONE', #15809 ) ;
#45819=EDGE_LOOP ( 'NONE', ( #56207, #56051, #74520 ) ) ;
#45821=EDGE_LOOP ( 'NONE', ( #75983, #70955, #19412, #31243 ) ) ;
#45824=CARTESIAN_POINT ( 'NONE',  ( 2.800715669567023003, 1.143166703770569281, -0.2643333500026459060 ) ) ;
#45886=DIRECTION ( 'NONE',  ( 0.000000000000000000, -1.000000000000000000, 1.408710688920637755E-15 ) ) ;
#45913=DIRECTION ( 'NONE',  ( 0.000000000000000000, 0.000000000000000000, 1.000000000000000000 ) ) ;
#45919=DIRECTION ( 'NONE',  ( 0.000000000000000000, 0.000000000000000000, 1.000000000000000000 ) ) ;
#45925=ORIENTED_EDGE ( 'NONE', *, *, #25308, .F. ) ;
#45935=CARTESIAN_POINT ( 'NONE',  ( 2.583694225513480713, 2.755905511811024056, -0.5314960629921260393 ) ) ;
#45943=ORIENTED_EDGE ( 'NONE', *, *, #41383, .T. ) ;
#45967=EDGE_CURVE ( 'NONE', #19542, #40260, #54908, .T. ) ;
#45971=DIRECTION ( 'NONE',  ( 0.000000000000000000, 1.000000000000000000, -0.000000000000000000 ) ) ;
#45972=CARTESIAN_POINT ( 'NONE',  ( -3.886287458032462006, 2.165354330708661568, 0.6299212598425196763 ) ) ;
#45984=CARTESIAN_POINT ( 'NONE',  ( 2.503252890251015828, 2.755905511811024056, -0.5314960629921260393 ) ) ;
#45996=B_SPLINE_CURVE_WITH_KNOTS ( 'NONE', 3,
 ( #75921, #18260, #19070, #6445, #24958, #50630, #31699, #57358, #17854, #69599, #32116, #57774, #137, #63275, #25793, #17448, #51453, #68775, #11119, #30872, #30465, #5208, #5615, #24145, #36776, #56128, #69184, #11535, #37192, #56539, #82240, #24559, #59456, #45141, #6860, #1807, #32952, #40522, #27053, #58618, #51876, #78838, #77582, #71677, #34206, #39260, #14029, #986, #52295, #78423, #39685, #65377 ),
 .UNSPECIFIED., .F., .F.,
 ( 4, 2, 2, 2, 2, 2, 2, 2, 2, 2, 2, 2, 2, 2, 2, 2, 2, 2, 2, 2, 2, 2, 2, 2, 2, 4 ),
 ( 0.000000000000000000, 0.002382837996120773603, 0.003574256994181160187, 0.004765675992241547206, 0.007148513988362320375, 0.008339932986422706959, 0.009531351984483092676, 0.01072277098254347839, 0.01191418998060386758, 0.01429702797672463208, 0.01548844697478501606, 0.01667986597284539657, 0.01906270396896615066, 0.02025412296702652770, 0.02144554196508690821, 0.02263696096314728873, 0.02382837996120766577, 0.02621121795732841986, 0.02740263695538880037, 0.02859405595344917742, 0.03097689394956994538, 0.03216831294763032589, 0.03335973194569070988, 0.03574256994181145702, 0.03693398893987184101, 0.03812540793793221805 ),
 .UNSPECIFIED. ) ;
#46001=CARTESIAN_POINT ( 'NONE',  ( 0.9881811337016640495, 0.000000000000000000, -0.5314960629921260393 ) ) ;
#46008=CARTESIAN_POINT ( 'NONE',  ( 3.924389226575468737, 2.559055118110236560, -0.3149606299212596716 ) ) ;
#46015=EDGE_CURVE ( 'NONE', #2910, #29808, #18171, .T. ) ;
#46020=CARTESIAN_POINT ( 'NONE',  ( 0.4713250013438510799, 1.474963701727497467, 1.018277200043820274 ) ) ;
#46039=ORIENTED_EDGE ( 'NONE', *, *, #24992, .T. ) ;
#46044=DIRECTION ( 'NONE',  ( 0.000000000000000000, 0.000000000000000000, -1.000000000000000000 ) ) ;
#46045=AXIS2_PLACEMENT_3D ( 'NONE', #63859, #57534, #83225 ) ;
#46046=CARTESIAN_POINT ( 'NONE',  ( -0.4426149705447187110, 1.366040861858872635, 2.619418448465752558 ) ) ;
#46047=CARTESIAN_POINT ( 'NONE',  ( 0.4177787735907000366, 0.3937007874015747699, -1.757006255033530806 ) ) ;
#46056=CARTESIAN_POINT ( 'NONE',  ( -1.016821367227983552, 1.537401574803149984, -0.4744094488188975722 ) ) ;
#46064=CARTESIAN_POINT ( 'NONE',  ( -3.937007874015748143, 2.559055118110236560, 0.5314960629921260393 ) ) ;
#46112=AXIS2_PLACEMENT_3D ( 'NONE', #72207, #2747, #20438 ) ;
#46113=CARTESIAN_POINT ( 'NONE',  ( 0.2980541528757573722, 1.168268747105946970, -1.689904592075601952 ) ) ;
#46125=VERTEX_POINT ( 'NONE', #22926 ) ;
#46143=EDGE_LOOP ( 'NONE', ( #76278, #69009, #5363, #26695 ) ) ;
#46144=CARTESIAN_POINT ( 'NONE',  ( 3.937007874015748143, 2.755905511811024056, 0.5314960629921260393 ) ) ;
#46161=ORIENTED_EDGE ( 'NONE', *, *, #53975, .T. ) ;
#46166=CARTESIAN_POINT ( 'NONE',  ( -2.149112266099376445, 1.629972608277048485, 0.4653577321740515194 ) ) ;
#46199=CARTESIAN_POINT ( 'NONE',  ( -2.570293866835912766, 2.742779993824306484, -0.5314960629921260393 ) ) ;
#46215=EDGE_LOOP ( 'NONE', ( #81667, #70111, #83129, #26774, #16759 ) ) ;
#46216=CARTESIAN_POINT ( 'NONE',  ( 2.362204724409448620, 1.929133858267716661, -0.5118110236220390075 ) ) ;
#46224=CARTESIAN_POINT ( 'NONE',  ( 0.4744094488189112835, 1.537401574803149984, -3.908320185825791881 ) ) ;
#46234=CIRCLE ( 'NONE', #11289, 0.3149606299212597826 ) ;
#46245=VERTEX_POINT ( 'NONE', #47344 ) ;
#46253=AXIS2_PLACEMENT_3D ( 'NONE', #43274, #4577, #63070 ) ;
#46255=LINE ( 'NONE', #46676, #69448 ) ;
#46288=CARTESIAN_POINT ( 'NONE',  ( -0.5314960629921123836, 2.677165354330708791, -3.900966923095591454 ) ) ;
#46293=ADVANCED_FACE ( 'NONE', ( #73877 ), #16216, .F. ) ;
#46314=LINE ( 'NONE', #28630, #40740 ) ;
#46321=CARTESIAN_POINT ( 'NONE',  ( 0.4670766846051074284, 1.622013716815571716, -2.152792308923968889 ) ) ;
#46326=CARTESIAN_POINT ( 'NONE',  ( -1.559171609364246924, 0.2755905511811023723, 0.4177787735906735578 ) ) ;
#46329=ORIENTED_EDGE ( 'NONE', *, *, #23423, .T. ) ;
#46349=ORIENTED_EDGE ( 'NONE', *, *, #61973, .F. ) ;
#46353=B_SPLINE_CURVE_WITH_KNOTS ( 'NONE', 3,
 ( #75387, #30337, #74985, #48872, #5495, #42960, #49692, #68654 ),
 .UNSPECIFIED., .F., .F.,
 ( 4, 2, 2, 4 ),
 ( 0.07134069304684194368, 0.07377942048615132586, 0.07499878420580602389, 0.07621814792546072193 ),
 .UNSPECIFIED. ) ;
#46410=CARTESIAN_POINT ( 'NONE',  ( -3.184294706754630777, 2.755905511811024056, 0.5314960629921260393 ) ) ;
#46415=EDGE_CURVE ( 'NONE', #53272, #74015, #35403, .T. ) ;
#46418=EDGE_CURVE ( 'NONE', #32355, #69205, #70286, .T. ) ;
#46422=DIRECTION ( 'NONE',  ( 0.000000000000000000, -1.000000000000000000, 1.408710688920637755E-15 ) ) ;
#46441=CARTESIAN_POINT ( 'NONE',  ( 0.000000000000000000, 2.716535433070866645, 0.000000000000000000 ) ) ;
#46461=ORIENTED_EDGE ( 'NONE', *, *, #52742, .T. ) ;
#46465=CARTESIAN_POINT ( 'NONE',  ( -0.3634034883589671860, 1.231066118352837968, 2.723611671832316006 ) ) ;
#46474=CARTESIAN_POINT ( 'NONE',  ( 1.076935383196057305, 2.559055118110236560, 0.3149606299212599492 ) ) ;
#46475=CARTESIAN_POINT ( 'NONE',  ( 0.000000000000000000, 2.755905511811024056, 0.000000000000000000 ) ) ;
#46480=ORIENTED_EDGE ( 'NONE', *, *, #27052, .T. ) ;
#46481=DIRECTION ( 'NONE',  ( 0.000000000000000000, 0.000000000000000000, -1.000000000000000000 ) ) ;
#46521=VECTOR ( 'NONE', #82847, 39.37007874015748143 ) ;
#46529=CARTESIAN_POINT ( 'NONE',  ( 0.2470981898865924897, 1.132419612620494842, -1.607172560345370149 ) ) ;
#46541=ORIENTED_EDGE ( 'NONE', *, *, #3802, .T. ) ;
#46542=ORIENTED_EDGE ( 'NONE', *, *, #25459, .F. ) ;
#46548=DIRECTION ( 'NONE',  ( 0.000000000000000000, 1.000000000000000000, 0.000000000000000000 ) ) ;
#46567=DIRECTION ( 'NONE',  ( -0.000000000000000000, 1.000000000000000000, -0.000000000000000000 ) ) ;
#46574=EDGE_CURVE ( 'NONE', #21301, #82069, #19821, .T. ) ;
#46584=CARTESIAN_POINT ( 'NONE',  ( 2.153151837758401577, 1.453715418023198147, -0.4672341690643350698 ) ) ;
#46586=TOROIDAL_SURFACE ( 'NONE', #21061, 3.858267716535433323, 0.07874015748031495954 ) ;
#46607=EDGE_CURVE ( 'NONE', #55113, #2780, #13897, .T. ) ;
#46613=EDGE_CURVE ( 'NONE', #62933, #17581, #65297, .T. ) ;
#46617=CARTESIAN_POINT ( 'NONE',  ( -1.313877454013331780, 0.2929341459200028863, 0.7983292792091805090 ) ) ;
#46629=CARTESIAN_POINT ( 'NONE',  ( -0.4359958488159856316, 1.724409448818897905, 3.912791665790197992 ) ) ;
#46633=FACE_BOUND ( 'NONE', #20577, .T. ) ;
#46636=VECTOR ( 'NONE', #4705, 39.37007874015748143 ) ;
#46642=PLANE ( 'NONE',  #38201 ) ;
#46644=CIRCLE ( 'NONE', #2265, 1.198416298106748767 ) ;
#46645=CARTESIAN_POINT ( 'NONE',  ( 3.937007874015748143, 1.537401574803149984, 2.901595197523589142E-16 ) ) ;
#46648=VERTEX_POINT ( 'NONE', #39164 ) ;
#46669=CARTESIAN_POINT ( 'NONE',  ( 2.867261597185502442, 1.070284760220068687, 0.08454815954498202946 ) ) ;
#46676=CARTESIAN_POINT ( 'NONE',  ( -0.5314960629921122726, 2.755905511811024056, -3.937007874015763687 ) ) ;
#46682=CARTESIAN_POINT ( 'NONE',  ( -2.557182324916528859, 1.572090529166661588, 0.4732185887570796723 ) ) ;
#46708=AXIS2_PLACEMENT_3D ( 'NONE', #3882, #42581, #49307 ) ;
#46710=CARTESIAN_POINT ( 'NONE',  ( -0.5314960629921123836, 2.702643891907236195, -3.896872718254348111 ) ) ;
#46717=DIRECTION ( 'NONE',  ( -0.000000000000000000, -1.000000000000000000, -0.000000000000000000 ) ) ;
#46748=VERTEX_POINT ( 'NONE', #47980 ) ;
#46751=ORIENTED_EDGE ( 'NONE', *, *, #6175, .T. ) ;
#46757=CARTESIAN_POINT ( 'NONE',  ( 0.05807346738891932397, 1.066559990163497229, -1.546459320796472303 ) ) ;
#46764=EDGE_CURVE ( 'NONE', #6265, #40586, #46314, .T. ) ;
#46784=DIRECTION ( 'NONE',  ( -3.491481338843132961E-15, -0.000000000000000000, 1.000000000000000000 ) ) ;
#46820=CARTESIAN_POINT ( 'NONE',  ( -1.559171609364246924, 1.299212598425196985, 0.4177787735906735578 ) ) ;
#46823=CARTESIAN_POINT ( 'NONE',  ( 4.821444151489972621E-16, 1.062992125984252745, 3.937007874015748143 ) ) ;
#46829=CARTESIAN_POINT ( 'NONE',  ( -3.210901144579272781, 2.729659898143634411, 0.5314960629921260393 ) ) ;
#46845=CARTESIAN_POINT ( 'NONE',  ( 3.890406373195415490, 2.716724272663529227, -0.5314960629921260393 ) ) ;
#46853=EDGE_CURVE ( 'NONE', #20068, #65211, #33701, .T. ) ;
#46855=DIRECTION ( 'NONE',  ( 0.000000000000000000, 0.000000000000000000, -1.000000000000000000 ) ) ;
#46872=ORIENTED_EDGE ( 'NONE', *, *, #26230, .T. ) ;
#46891=LINE ( 'NONE', #14106, #29119 ) ;
#46904=CYLINDRICAL_SURFACE ( 'NONE', #43797, 0.3149606299212597826 ) ;
#46916=AXIS2_PLACEMENT_3D ( 'NONE', #71425, #51204, #83217 ) ;
#46930=B_SPLINE_CURVE_WITH_KNOTS ( 'NONE', 3,
 ( #36274, #61946, #4286, #24459 ),
 .UNSPECIFIED., .F., .F.,
 ( 4, 4 ),
 ( 9.992028926250184212E-07, 0.001428690226504376057 ),
 .UNSPECIFIED. ) ;
#46954=ORIENTED_EDGE ( 'NONE', *, *, #38297, .T. ) ;
#46971=EDGE_LOOP ( 'NONE', ( #43329, #81496, #73403, #37756, #29892, #14811 ) ) ;
#46979=CARTESIAN_POINT ( 'NONE',  ( 3.886287458032462006, 2.165354330708661568, -0.6299212598425196763 ) ) ;
#46990=ORIENTED_EDGE ( 'NONE', *, *, #50488, .T. ) ;
#46997=CARTESIAN_POINT ( 'NONE',  ( 1.964414453380805892, 1.188885443925065566, -0.3231744412229926033 ) ) ;
#47004=CARTESIAN_POINT ( 'NONE',  ( -0.4706608522957314578, 1.597527518877483788, 2.563288228875758801 ) ) ;
#47021=EDGE_CURVE ( 'NONE', #15514, #31453, #21898, .T. ) ;
#47054=DIRECTION ( 'NONE',  ( -1.000000000000000000, -0.000000000000000000, -0.000000000000000000 ) ) ;
#47056=ORIENTED_EDGE ( 'NONE', *, *, #48666, .F. ) ;
#47069=ADVANCED_FACE ( 'NONE', ( #79169 ), #79757, .F. ) ;
#47075=ORIENTED_EDGE ( 'NONE', *, *, #26715, .F. ) ;
#47078=CARTESIAN_POINT ( 'NONE',  ( 2.841478809456089216, 1.098283573398297852, 0.1802708669123707919 ) ) ;
#47097=EDGE_CURVE ( 'NONE', #34868, #10035, #5752, .T. ) ;
#47112=CONICAL_SURFACE ( 'NONE', #56534, 0.1190944881889763746, 0.8726646259971682085 ) ;
#47120=CARTESIAN_POINT ( 'NONE',  ( -0.5314960629921124946, 2.725289161120229675, -3.884611959489590483 ) ) ;
#47141=EDGE_CURVE ( 'NONE', #32861, #60543, #38024, .T. ) ;
#47151=CARTESIAN_POINT ( 'NONE',  ( 0.4562819726585566893, 1.668167360224330986, -2.130140035730256454 ) ) ;
#47155=CARTESIAN_POINT ( 'NONE',  ( 0.000000000000000000, 2.755905511811024056, 0.000000000000000000 ) ) ;
#47168=CARTESIAN_POINT ( 'NONE',  ( -0.4697362858026991606, 1.605934398054998047, -2.565479853601120297 ) ) ;
#47171=AXIS2_PLACEMENT_3D ( 'NONE', #76147, #32343, #18487 ) ;
#47178=ORIENTED_EDGE ( 'NONE', *, *, #60737, .F. ) ;
#47181=ORIENTED_EDGE ( 'NONE', *, *, #2120, .F. ) ;
#47193=CONICAL_SURFACE ( 'NONE', #64616, 2.165354330708661568, 0.7853981633974500554 ) ;
#47236=CARTESIAN_POINT ( 'NONE',  ( 0.4177787735907000366, 0.4110443821404751730, -1.382006255033530806 ) ) ;
#47258=ORIENTED_EDGE ( 'NONE', *, *, #32702, .F. ) ;
#47261=CARTESIAN_POINT ( 'NONE',  ( 3.842312626974349943, 2.753838553078471918, -0.5314960629921259283 ) ) ;
#47271=LINE ( 'NONE', #42618, #51643 ) ;
#47286=CIRCLE ( 'NONE', #75549, 3.858267716535433323 ) ;
#47289=ORIENTED_EDGE ( 'NONE', *, *, #26230, .F. ) ;
#47291=EDGE_LOOP ( 'NONE', ( #4600, #67684, #22131 ) ) ;
#47294=FACE_OUTER_BOUND ( 'NONE', #74001, .T. ) ;
#47296=DIRECTION ( 'NONE',  ( 0.000000000000000000, 0.000000000000000000, 1.000000000000000000 ) ) ;
#47302=ORIENTED_EDGE ( 'NONE', *, *, #67469, .F. ) ;
#47313=DIRECTION ( 'NONE',  ( 0.000000000000000000, 0.000000000000000000, -1.000000000000000000 ) ) ;
#47329=ADVANCED_FACE ( 'NONE', ( #29039 ), #35362, .F. ) ;
#47344=CARTESIAN_POINT ( 'NONE',  ( 2.543486866223389153, 2.716535433070866645, -0.5314960629921260393 ) ) ;
#47346=CIRCLE ( 'NONE', #60754, 3.937007874015748143 ) ;
#47347=ORIENTED_EDGE ( 'NONE', *, *, #80947, .T. ) ;
#47373=VERTEX_POINT ( 'NONE', #3790 ) ;
#47393=CARTESIAN_POINT ( 'NONE',  ( -1.592472994958951560, 1.379238946755884987, 0.4472770027453138453 ) ) ;
#47399=CARTESIAN_POINT ( 'NONE',  ( 3.184294706754630777, 2.755905511811024056, -0.5314960629921260393 ) ) ;
#47410=ORIENTED_EDGE ( 'NONE', *, *, #39907, .T. ) ;
#47426=DIRECTION ( 'NONE',  ( 1.000000000000000000, 1.601283208593976204E-15, 0.000000000000000000 ) ) ;
#47438=DIRECTION ( 'NONE',  ( 0.000000000000000000, 0.000000000000000000, -1.000000000000000000 ) ) ;
#47444=DIRECTION ( 'NONE',  ( -0.000000000000000000, -1.000000000000000000, -0.000000000000000000 ) ) ;
#47458=CARTESIAN_POINT ( 'NONE',  ( -3.890345922373659615, 2.716830163678111365, -0.5314960629921260393 ) ) ;
#47465=EDGE_CURVE ( 'NONE', #16450, #78262, #42078, .T. ) ;
#47494=CARTESIAN_POINT ( 'NONE',  ( 2.873989802184792719, 1.063020117359137817, -0.01785754392581748520 ) ) ;
#47503=AXIS2_PLACEMENT_3D ( 'NONE', #68168, #16832, #10511 ) ;
#47506=ORIENTED_EDGE ( 'NONE', *, *, #12502, .T. ) ;
#47508=CARTESIAN_POINT ( 'NONE',  ( 0.000000000000000000, 2.755905511811024056, 0.000000000000000000 ) ) ;
#47509=ORIENTED_EDGE ( 'NONE', *, *, #19828, .T. ) ;
#47523=AXIS2_PLACEMENT_3D ( 'NONE', #35295, #4129, #80754 ) ;
#47530=CARTESIAN_POINT ( 'NONE',  ( 0.000000000000000000, 2.716535433070866645, 0.000000000000000000 ) ) ;
#47536=CARTESIAN_POINT ( 'NONE',  ( 0.5314960629920856272, 2.753838553078471918, 3.842312626974355716 ) ) ;
#47538=EDGE_CURVE ( 'NONE', #76587, #42095, #29681, .T. ) ;
#47561=DIRECTION ( 'NONE',  ( -0.000000000000000000, 1.000000000000000000, -0.000000000000000000 ) ) ;
#47563=AXIS2_PLACEMENT_3D ( 'NONE', #4855, #62104, #43553 ) ;
#47568=PLANE ( 'NONE',  #8215 ) ;
#47571=LINE ( 'NONE', #80427, #39533 ) ;
#47578=AXIS2_PLACEMENT_3D ( 'NONE', #11298, #17619, #55471 ) ;
#47586=CARTESIAN_POINT ( 'NONE',  ( -3.886287458032462006, 2.165354330708662012, -0.6299212598425202314 ) ) ;
#47592=DIRECTION ( 'NONE',  ( 0.000000000000000000, 0.000000000000000000, -1.000000000000000000 ) ) ;
#47598=ORIENTED_EDGE ( 'NONE', *, *, #28057, .F. ) ;
#47614=CARTESIAN_POINT ( 'NONE',  ( 3.913952425448613770, 1.327060745706139411, 0.4255134223640585911 ) ) ;
#47621=ADVANCED_FACE ( 'NONE', ( #37004 ), #69412, .F. ) ;
#47634=CARTESIAN_POINT ( 'NONE',  ( -0.07848924910222174200, 1.069269829744720290, -1.119403926637735358 ) ) ;
#47636=CARTESIAN_POINT ( 'NONE',  ( 3.937007874015748143, 2.165354330708661568, -0.3149606299212595606 ) ) ;
#47643=CIRCLE ( 'NONE', #67853, 0.5118110236220472231 ) ;
#47654=DIRECTION ( 'NONE',  ( 0.000000000000000000, 0.000000000000000000, 1.000000000000000000 ) ) ;
#47665=CARTESIAN_POINT ( 'NONE',  ( -1.573327616418469521, 1.128537896298102305, 0.2406134192599649613 ) ) ;
#47667=DIRECTION ( 'NONE',  ( 0.000000000000000000, -1.000000000000000000, 0.000000000000000000 ) ) ;
#47674=ORIENTED_EDGE ( 'NONE', *, *, #51210, .F. ) ;
#47678=DIRECTION ( 'NONE',  ( -1.000000000000000000, -0.000000000000000000, -0.000000000000000000 ) ) ;
#47704=LINE ( 'NONE', #74232, #62763 ) ;
#47707=EDGE_LOOP ( 'NONE', ( #6804, #74446, #77083 ) ) ;
#47710=CARTESIAN_POINT ( 'NONE',  ( 0.4653577321740434147, 1.629972608277053148, 2.149112266099304502 ) ) ;
#47711=CARTESIAN_POINT ( 'NONE',  ( -0.4478287522207295979, 1.694786963789534084, 3.911458005082129041 ) ) ;
#47720=ORIENTED_EDGE ( 'NONE', *, *, #17120, .F. ) ;
#47722=CARTESIAN_POINT ( 'NONE',  ( -1.313877454013331780, 1.062992125984252079, 0.8967544760595740350 ) ) ;
#47723=DIRECTION ( 'NONE',  ( -0.000000000000000000, -1.000000000000000000, -0.000000000000000000 ) ) ;
#47736=CARTESIAN_POINT ( 'NONE',  ( 1.348312163386739426, 0.2755905511811023723, 0.7386866130305692613 ) ) ;
#47746=AXIS2_PLACEMENT_3D ( 'NONE', #28715, #34626, #61533 ) ;
#47752=VECTOR ( 'NONE', #22961, 39.37007874015748143 ) ;
#47762=EDGE_LOOP ( 'NONE', ( #58156, #14291, #21808, #18501 ) ) ;
#47788=ORIENTED_EDGE ( 'NONE', *, *, #4386, .T. ) ;
#47806=EDGE_LOOP ( 'NONE', ( #7018, #82584, #49367, #65553 ) ) ;
#47810=VECTOR ( 'NONE', #81800, 39.37007874015748143 ) ;
#47814=CARTESIAN_POINT ( 'NONE',  ( 1.016821367227983774, 1.537401574803149984, -0.4744094488188970171 ) ) ;
#47818=EDGE_CURVE ( 'NONE', #60402, #21709, #71068, .T. ) ;
#47824=CARTESIAN_POINT ( 'NONE',  ( 0.5314960629921396951, 2.729373344522950440, -3.881211926161856507 ) ) ;
#47825=ORIENTED_EDGE ( 'NONE', *, *, #62552, .F. ) ;
#47829=CARTESIAN_POINT ( 'NONE',  ( 1.877461585981321068, 1.092324130688948181, -0.1650676745531886869 ) ) ;
#47858=CARTESIAN_POINT ( 'NONE',  ( 0.000000000000000000, 2.165354330708661568, 0.000000000000000000 ) ) ;
#47874=LINE ( 'NONE', #73578, #40106 ) ;
#47880=CARTESIAN_POINT ( 'NONE',  ( -2.543486866223389153, 2.716535433070866645, -0.5314960629921260393 ) ) ;
#47902=VECTOR ( 'NONE', #83139, 39.37007874015748143 ) ;
#47903=ORIENTED_EDGE ( 'NONE', *, *, #6316, .F. ) ;
#47906=CIRCLE ( 'NONE', #22398, 1.289370078740159409 ) ;
#47908=CARTESIAN_POINT ( 'NONE',  ( 1.141392835773558767, 1.405664282898583473, 1.141392835773562764 ) ) ;
#47914=DIRECTION ( 'NONE',  ( 0.000000000000000000, 0.000000000000000000, 1.000000000000000000 ) ) ;
#47919=ORIENTED_EDGE ( 'NONE', *, *, #83070, .F. ) ;
#47922=VERTEX_POINT ( 'NONE', #12168 ) ;
#47932=VECTOR ( 'NONE', #41827, 39.37007874015748143 ) ;
#47946=CARTESIAN_POINT ( 'NONE',  ( 1.141392835773559211, 0.3937007874015747699, 0.9435581901042713326 ) ) ;
#47961=AXIS2_PLACEMENT_3D ( 'NONE', #70125, #63812, #74091 ) ;
#47971=CIRCLE ( 'NONE', #23762, 0.5118110236220471121 ) ;
#47974=DIRECTION ( 'NONE',  ( 0.000000000000000000, 0.000000000000000000, -1.000000000000000000 ) ) ;
#47980=CARTESIAN_POINT ( 'NONE',  ( -3.886287458032462006, 1.724409448818897905, 0.6299212598425196763 ) ) ;
#47984=ADVANCED_FACE ( 'NONE', ( #18485 ), #63093, .F. ) ;
#47987=CARTESIAN_POINT ( 'NONE',  ( 0.5314960629920851831, 2.755905511811024056, 3.900966923095595451 ) ) ;
#47994=ORIENTED_EDGE ( 'NONE', *, *, #80559, .T. ) ;
#48008=CARTESIAN_POINT ( 'NONE',  ( 0.2516118885077293643, 1.134065313995062718, -2.808863443762336765 ) ) ;
#48011=ORIENTED_EDGE ( 'NONE', *, *, #75818, .F. ) ;
#48033=VECTOR ( 'NONE', #40399, 39.37007874015748143 ) ;
#48043=DIRECTION ( 'NONE',  ( 1.047444401652940007E-14, 0.000000000000000000, -1.000000000000000000 ) ) ;
#48050=DIRECTION ( 'NONE',  ( -0.000000000000000000, -1.000000000000000000, -0.000000000000000000 ) ) ;
#48057=CARTESIAN_POINT ( 'NONE',  ( -1.291027602697912169, 0.000000000000000000, 0.5830028338522510456 ) ) ;
#48082=CARTESIAN_POINT ( 'NONE',  ( 0.000000000000000000, 2.755905511811024056, 0.000000000000000000 ) ) ;
#48094=DIRECTION ( 'NONE',  ( 1.000000000000000000, 0.000000000000000000, 3.455050906509825972E-15 ) ) ;
#48095=EDGE_CURVE ( 'NONE', #32357, #24500, #17975, .T. ) ;
#48121=CARTESIAN_POINT ( 'NONE',  ( -0.03416814150274047335, 1.063911309852950682, -2.873163370116321946 ) ) ;
#48123=CARTESIAN_POINT ( 'NONE',  ( -0.03443470937339727228, 0.2755905511811023723, -1.417921404050779710 ) ) ;
#48124=EDGE_CURVE ( 'NONE', #32589, #13567, #4483, .T. ) ;
#48126=VERTEX_POINT ( 'NONE', #7088 ) ;
#48132=CARTESIAN_POINT ( 'NONE',  ( -1.313877454013331780, 0.2755905511811023723, 0.6792347910202041206 ) ) ;
#48143=CARTESIAN_POINT ( 'NONE',  ( 0.000000000000000000, 2.755905511811024056, 0.000000000000000000 ) ) ;
#48151=LINE ( 'NONE', #73846, #66805 ) ;
#48166=DIRECTION ( 'NONE',  ( -0.000000000000000000, 1.000000000000000000, -0.000000000000000000 ) ) ;
#48177=CARTESIAN_POINT ( 'NONE',  ( 0.4477177017962634675, 1.379801381128189064, 2.114025566600534312 ) ) ;
#48196=CARTESIAN_POINT ( 'NONE',  ( -2.516666444179625373, 2.742784451071572427, 0.5314960629921260393 ) ) ;
#48208=CARTESIAN_POINT ( 'NONE',  ( -1.559171609364246924, 0.3937007874015748254, 0.2406134192599649890 ) ) ;
#48210=ORIENTED_EDGE ( 'NONE', *, *, #82633, .F. ) ;
#48226=ORIENTED_EDGE ( 'NONE', *, *, #5997, .T. ) ;
#48229=CARTESIAN_POINT ( 'NONE',  ( -1.736178228450298011, 1.299212598425196985, 0.4102808022082834460 ) ) ;
#48232=FACE_OUTER_BOUND ( 'NONE', #13549, .T. ) ;
#48247=CARTESIAN_POINT ( 'NONE',  ( 1.850381573804679158, 1.062979042929935058, -0.007789085821702718300 ) ) ;
#48298=CARTESIAN_POINT ( 'NONE',  ( -3.908320185825790993, 1.553415232435839677, 0.4744094488188969616 ) ) ;
#48302=ORIENTED_EDGE ( 'NONE', *, *, #67409, .T. ) ;
#48304=ORIENTED_EDGE ( 'NONE', *, *, #42584, .T. ) ;
#48318=VERTEX_POINT ( 'NONE', #8161 ) ;
#48321=CARTESIAN_POINT ( 'NONE',  ( -0.5314960629921373636, 2.755905511811024056, 3.264097702071371288 ) ) ;
#48356=CARTESIAN_POINT ( 'NONE',  ( 0.000000000000000000, 1.724409448818897461, -2.362204724409448620 ) ) ;
#48361=CARTESIAN_POINT ( 'NONE',  ( 0.5314960629920855162, 2.740199102106095186, 3.870235431238107981 ) ) ;
#48370=CARTESIAN_POINT ( 'NONE',  ( 0.5314960629921325896, 2.755905511811024056, -1.895394334970790018 ) ) ;
#48374=EDGE_CURVE ( 'NONE', #32076, #35211, #34618, .T. ) ;
#48387=CARTESIAN_POINT ( 'NONE',  ( -3.224202737261815166, 2.716535433070866645, 0.5314960629921260393 ) ) ;
#48388=VERTEX_POINT ( 'NONE', #1024 ) ;
#48391=CARTESIAN_POINT ( 'NONE',  ( 0.2540590912309962368, 1.136744334959988389, -1.491123965641447002 ) ) ;
#48397=CARTESIAN_POINT ( 'NONE',  ( -3.900966923095589678, 2.559055118110236560, -0.5314960629921260393 ) ) ;
#48410=CARTESIAN_POINT ( 'NONE',  ( -0.4744094488188832504, 1.537401574803149984, -3.937007874015763687 ) ) ;
#48415=B_SPLINE_CURVE_WITH_KNOTS ( 'NONE', 3,
 ( #27424, #72473, #77536, #45935 ),
 .UNSPECIFIED., .F., .F.,
 ( 4, 4 ),
 ( 0.1331161126011571050, 0.1345277053022634894 ),
 .UNSPECIFIED. ) ;
#48416=CARTESIAN_POINT ( 'NONE',  ( 0.3335738234991732498, 1.199759523613724843, -2.750612009938800284 ) ) ;
#48429=VECTOR ( 'NONE', #60686, 39.37007874015748143 ) ;
#48438=CARTESIAN_POINT ( 'NONE',  ( -0.5314960629921371416, 2.755905511811024056, 3.184294706754628557 ) ) ;
#48450=DIRECTION ( 'NONE',  ( 1.000000000000000000, -0.000000000000000000, -0.000000000000000000 ) ) ;
#48465=CARTESIAN_POINT ( 'NONE',  ( 1.895394334970792016, 2.755905511811024056, -0.5314960629921260393 ) ) ;
#48473=CARTESIAN_POINT ( 'NONE',  ( -0.005475238697255037888, 1.062992125984248304, -1.631265707957251010 ) ) ;
#48486=CIRCLE ( 'NONE', #71332, 3.937007874015748143 ) ;
#48489=CARTESIAN_POINT ( 'NONE',  ( -1.650841896953458843, 1.144577896360981395, 0.2660319121884003879 ) ) ;
#48491=DIRECTION ( 'NONE',  ( -0.000000000000000000, -1.000000000000000000, -0.000000000000000000 ) ) ;
#48502=CARTESIAN_POINT ( 'NONE',  ( 3.898413161119330450, 2.697625129285034173, -0.5314960629921259283 ) ) ;
#48506=EDGE_CURVE ( 'NONE', #50475, #56091, #59792, .T. ) ;
#48514=ADVANCED_FACE ( 'NONE', ( #7320 ), #79293, .F. ) ;
#48515=CARTESIAN_POINT ( 'NONE',  ( 0.4422585667712756741, 1.709808357580390625, 3.912093821574601282 ) ) ;
#48529=CARTESIAN_POINT ( 'NONE',  ( -0.3635331417845649726, 1.231226750417221183, -2.723475981305045313 ) ) ;
#48538=CARTESIAN_POINT ( 'NONE',  ( 0.000000000000000000, 2.755905511811024056, 0.000000000000000000 ) ) ;
#48539=CARTESIAN_POINT ( 'NONE',  ( -3.250800425606660049, 2.742781087017835961, -0.5314960629921260393 ) ) ;
#48541=EDGE_CURVE ( 'NONE', #9951, #9892, #44786, .T. ) ;
#48542=FACE_BOUND ( 'NONE', #22741, .T. ) ;
#48551=AXIS2_PLACEMENT_3D ( 'NONE', #19230, #49976, #23901 ) ;
#48560=DIRECTION ( 'NONE',  ( 0.000000000000000000, 0.000000000000000000, 1.000000000000000000 ) ) ;
#48561=FACE_OUTER_BOUND ( 'NONE', #42025, .T. ) ;
#48568=CARTESIAN_POINT ( 'NONE',  ( 2.586150256253534785, 1.653403552777528596, -0.4602852883866567768 ) ) ;
#48571=CIRCLE ( 'NONE', #71407, 0.5118110236220471121 ) ;
#48593=ORIENTED_EDGE ( 'NONE', *, *, #7888, .T. ) ;
#48595=EDGE_CURVE ( 'NONE', #50169, #64186, #48844, .T. ) ;
#48604=B_SPLINE_CURVE_WITH_KNOTS ( 'NONE', 3,
 ( #70259, #58465, #6705, #32374, #45409, #63538, #76181, #7124, #82903, #58038, #77421, #63950, #44568, #19755, #20174, #828, #13869, #24810, #76589, #45824, #12614, #71523, #63127, #6287, #5465, #31962, #31127, #57623, #47494, #28563, #60137, #65216, #28147, #9214, #46669, #73186, #79105, #40366, #47078, #65643, #7555, #7973, #21424, #33636, #1248, #26897, #54219, #53803, #2488, #14711, #78265, #34887, #39528, #33226, #2067, #52556, #34471, #20596, #72769, #59299 ),
 .UNSPECIFIED., .F., .F.,
 ( 4, 2, 2, 2, 2, 2, 2, 2, 2, 2, 2, 2, 2, 2, 2, 2, 2, 2, 2, 2, 2, 2, 2, 2, 2, 2, 2, 2, 2, 4 ),
 ( 0.01323639539072392866, 0.01388181161316760608, 0.01452722783561128175, 0.01581806028049860535, 0.01710889272538592895, 0.01839972517027324908, 0.02098139006004787199, 0.02356305494982249837, 0.02485388739470980463, 0.02614471983959711088, 0.02743555228448441713, 0.02872638472937171991, 0.03130804961914634282, 0.03259888206403365601, 0.03388971450892096227, 0.03453513073136461886, 0.03518054695380826852, 0.03647137939869557477, 0.03776221184358288796, 0.03905304428847020115, 0.04034387673335750740, 0.04163470917824481365, 0.04421637406801944697, 0.04679803895779408723, 0.04937970384756872749, 0.05067053629245604762, 0.05196136873734337469, 0.05325220118223069482, 0.05389761740467436529, 0.05454303362711803577 ),
 .UNSPECIFIED. ) ;
#48611=CIRCLE ( 'NONE', #24393, 2.559055118110236560 ) ;
#48627=PLANE ( 'NONE',  #70581 ) ;
#48638=ORIENTED_EDGE ( 'NONE', *, *, #28964, .T. ) ;
#48641=CARTESIAN_POINT ( 'NONE',  ( 3.937007874015748143, 2.755905511811024056, 0.5314960629921260393 ) ) ;
#48665=DIRECTION ( 'NONE',  ( 0.000000000000000000, 0.000000000000000000, -1.000000000000000000 ) ) ;
#48666=EDGE_CURVE ( 'NONE', #64697, #51414, #27340, .T. ) ;
#48672=EDGE_CURVE ( 'NONE', #10674, #82069, #58261, .T. ) ;
#48706=B_SPLINE_CURVE_WITH_KNOTS ( 'NONE', 3,
 ( #4594, #12572, #37416, #82455, #63088, #43705, #76551, #23953, #25595, #25184, #31088, #24363, #51258, #75315, #17662, #68990, #24770, #62678, #38230, #11339, #36999, #82862, #63907, #50439, #69408, #6243, #56755, #5020, #76960, #36579, #19288, #30688, #82050, #50033, #76140, #18481, #44123, #71064, #27272, #13408, #19710, #21383, #77804, #39063, #53356, #70637, #59672, #65601, #20557 ),
 .UNSPECIFIED., .F., .F.,
 ( 4, 2, 2, 2, 2, 2, 2, 2, 2, 2, 2, 2, 2, 1, 2, 2, 2, 2, 2, 2, 2, 2, 2, 2, 4 ),
 ( 0.004857456657547474382, 0.007214810972081309864, 0.008393488129348227605, 0.009572165286615145346, 0.01192951960114899991, 0.01310819675841591939, 0.01428687391568283019, 0.01546555107294974273, 0.01664422823021665526, 0.01900158254475048034, 0.02135893685928430541, 0.02371629117381813048, 0.02489496833108504129, 0.02607364548835195209, 0.02725232264561886983, 0.02843099980288578063, 0.03078835411741961264, 0.03196703127468653038, 0.03314570843195344119, 0.03550306274648727667, 0.03668173990375418747, 0.03786041706102111215, 0.04021777137555496151, 0.04139644853282188619, 0.04257512569008879699 ),
 .UNSPECIFIED. ) ;
#48719=AXIS2_PLACEMENT_3D ( 'NONE', #78074, #39333, #65860 ) ;
#48749=CARTESIAN_POINT ( 'NONE',  ( 0.5314960629920993940, 2.716535433070866645, 2.543486866223394482 ) ) ;
#48756=LINE ( 'NONE', #1367, #35745 ) ;
#48765=EDGE_CURVE ( 'NONE', #63914, #39649, #80833, .T. ) ;
#48772=CARTESIAN_POINT ( 'NONE',  ( -3.210901149692899637, 2.729659893098101087, -0.5314960629921260393 ) ) ;
#48784=AXIS2_PLACEMENT_3D ( 'NONE', #19987, #14929, #51949 ) ;
#48798=CARTESIAN_POINT ( 'NONE',  ( 1.141392835773559211, 0.3937007874015748254, 1.141392835773562764 ) ) ;
#48817=ORIENTED_EDGE ( 'NONE', *, *, #37615, .F. ) ;
#48820=ORIENTED_EDGE ( 'NONE', *, *, #58440, .F. ) ;
#48826=CARTESIAN_POINT ( 'NONE',  ( 6.372542394380578105E-15, 1.062992125984252523, -1.629220936382730134 ) ) ;
#48844=CIRCLE ( 'NONE', #23311, 0.3149606299212597271 ) ;
#48872=CARTESIAN_POINT ( 'NONE',  ( 0.4678109194727930187, 1.617842475621884768, -1.019880138406202175 ) ) ;
#48899=AXIS2_PLACEMENT_3D ( 'NONE', #59888, #46422, #14051 ) ;
#48910=DIRECTION ( 'NONE',  ( 0.000000000000000000, 0.000000000000000000, 1.000000000000000000 ) ) ;
#48916=ORIENTED_EDGE ( 'NONE', *, *, #38141, .T. ) ;
#48932=CARTESIAN_POINT ( 'NONE',  ( 0.4711511276547932781, 1.601562584932245237, 3.908719782672964715 ) ) ;
#48944=AXIS2_PLACEMENT_3D ( 'NONE', #7200, #82563, #64023 ) ;
#48947=CARTESIAN_POINT ( 'NONE',  ( -0.1807872349014755242, 1.098494004316918460, -2.841285918040845626 ) ) ;
#48949=DIRECTION ( 'NONE',  ( 0.000000000000000000, 0.000000000000000000, 1.000000000000000000 ) ) ;
#48957=DIRECTION ( 'NONE',  ( 0.000000000000000000, 0.000000000000000000, -1.000000000000000000 ) ) ;
#48976=CARTESIAN_POINT ( 'NONE',  ( -2.118110236220477116, 0.000000000000000000, 0.4498537592782676509 ) ) ;
#48983=CARTESIAN_POINT ( 'NONE',  ( 2.594411373832371304, 1.668416680336019864, -0.4562095852119716355 ) ) ;
#49004=CARTESIAN_POINT ( 'NONE',  ( 0.4567729623170501685, 1.408376684009862378, 2.131114924183266091 ) ) ;
#49024=CARTESIAN_POINT ( 'NONE',  ( 0.000000000000000000, 0.03937007874015751446, 2.362204724409448620 ) ) ;
#49052=ORIENTED_EDGE ( 'NONE', *, *, #27675, .F. ) ;
#49058=FACE_OUTER_BOUND ( 'NONE', #20142, .T. ) ;
#49059=CARTESIAN_POINT ( 'NONE',  ( 0.5314960629921323676, 2.742788190551039396, -1.827151662668102361 ) ) ;
#49063=PRODUCT_DEFINITION_FORMATION_WITH_SPECIFIED_SOURCE ( 'ANY', '', #25763, .NOT_KNOWN. ) ;
#49097=CARTESIAN_POINT ( 'NONE',  ( -3.890406373195415490, 2.716724272663529227, 0.5314960629921260393 ) ) ;
#49100=ORIENTED_EDGE ( 'NONE', *, *, #59684, .T. ) ;
#49107=CARTESIAN_POINT ( 'NONE',  ( -0.3149606299212458493, 2.165354330708661568, -3.937007874015763242 ) ) ;
#49124=CONICAL_SURFACE ( 'NONE', #73312, 0.09842519685039351207, 1.029744258676651647 ) ;
#49134=EDGE_CURVE ( 'NONE', #34868, #26979, #12709, .T. ) ;
#49151=DIRECTION ( 'NONE',  ( -0.000000000000000000, -1.000000000000000000, -0.000000000000000000 ) ) ;
#49169=CARTESIAN_POINT ( 'NONE',  ( -0.2893911920035082685, 1.160213065395012899, 3.926441900275995600 ) ) ;
#49179=ADVANCED_FACE ( 'NONE', ( #78 ), #79816, .T. ) ;
#49190=VECTOR ( 'NONE', #81384, 39.37007874015748143 ) ;
#49191=CARTESIAN_POINT ( 'NONE',  ( -2.019766021329723937, 1.253539720428408888, 0.3811758253793102735 ) ) ;
#49220=FACE_OUTER_BOUND ( 'NONE', #21421, .T. ) ;
#49223=CARTESIAN_POINT ( 'NONE',  ( 1.141392835773559211, 0.2755905511811023723, 1.141392835773562764 ) ) ;
#49228=EDGE_CURVE ( 'NONE', #40163, #65284, #38080, .T. ) ;
#49244=CARTESIAN_POINT ( 'NONE',  ( 1.348312163386739426, 0.2755905511811023723, 0.7386866130305692613 ) ) ;
#49252=VECTOR ( 'NONE', #15456, 39.37007874015748143 ) ;
#49278=DIRECTION ( 'NONE',  ( 0.000000000000000000, -1.000000000000000000, 1.734723475976808327E-16 ) ) ;
#49285=CARTESIAN_POINT ( 'NONE',  ( -2.800975763476014180, 1.142877263639032748, -0.2639061591569959453 ) ) ;
#49288=CARTESIAN_POINT ( 'NONE',  ( 0.000000000000000000, 2.677165354330708791, 0.000000000000000000 ) ) ;
#49293=AXIS2_PLACEMENT_3D ( 'NONE', #25821, #52322, #78028 ) ;
#49303=CARTESIAN_POINT ( 'NONE',  ( 0.2887997841774525010, 1.160717306711469110, -1.939402670811599450 ) ) ;
#49307=DIRECTION ( 'NONE',  ( 0.000000000000000000, 0.000000000000000000, 1.000000000000000000 ) ) ;
#49320=DIRECTION ( 'NONE',  ( -0.000000000000000000, -1.000000000000000000, -0.000000000000000000 ) ) ;
#49321=DIRECTION ( 'NONE',  ( 0.000000000000000000, -0.000000000000000000, -1.000000000000000000 ) ) ;
#49322=CARTESIAN_POINT ( 'NONE',  ( -0.03443470937339728616, 0.2755905511811023723, -1.537015892239756099 ) ) ;
#49334=CARTESIAN_POINT ( 'NONE',  ( 2.130073781772665598, 0.01305114060239440966, 0.4563452811745986049 ) ) ;
#49345=VECTOR ( 'NONE', #1689, 39.37007874015748143 ) ;
#49349=CIRCLE ( 'NONE', #69487, 3.267716535433071279 ) ;
#49361=CARTESIAN_POINT ( 'NONE',  ( -0.4741766535082717060, 1.520234135998521863, -2.554840505098090020 ) ) ;
#49363=FACE_OUTER_BOUND ( 'NONE', #47291, .T. ) ;
#49366=VERTEX_POINT ( 'NONE', #82582 ) ;
#49367=ORIENTED_EDGE ( 'NONE', *, *, #20837, .F. ) ;
#49370=CARTESIAN_POINT ( 'NONE',  ( 0.5314960629921066104, 2.729664745829105232, 1.840814904541347774 ) ) ;
#49374=PRESENTATION_STYLE_ASSIGNMENT (( #11917 ) ) ;
#49389=B_SPLINE_CURVE_WITH_KNOTS ( 'NONE', 3,
 ( #53045, #33708, #64857, #32867 ),
 .UNSPECIFIED., .F., .F.,
 ( 4, 4 ),
 ( 0.1237084911784920305, 0.1251516581501740388 ),
 .UNSPECIFIED. ) ;
#49391=CARTESIAN_POINT ( 'NONE',  ( -3.912791665790199769, 1.724409448818897905, -0.4359958488159722534 ) ) ;
#49409=AXIS2_PLACEMENT_3D ( 'NONE', #73975, #28925, #42374 ) ;
#49427=EDGE_CURVE ( 'NONE', #13254, #55363, #35455, .T. ) ;
#49430=DIRECTION ( 'NONE',  ( 0.000000000000000000, 0.000000000000000000, 1.000000000000000000 ) ) ;
#49439=CARTESIAN_POINT ( 'NONE',  ( 3.912791665790199769, 1.724409448818897905, 0.4359958488159722534 ) ) ;
#49461=EDGE_CURVE ( 'NONE', #50709, #40260, #42174, .T. ) ;
#49467=ORIENTED_EDGE ( 'NONE', *, *, #52265, .F. ) ;
#49470=DIRECTION ( 'NONE',  ( 0.000000000000000000, -1.408710688920637755E-15, -1.000000000000000000 ) ) ;
#49471=VECTOR ( 'NONE', #17759, 39.37007874015748143 ) ;
#49477=CARTESIAN_POINT ( 'NONE',  ( 0.5314960629921322566, 2.755905511811024056, -1.813482582612291782 ) ) ;
#49485=VERTEX_POINT ( 'NONE', #6384 ) ;
#49495=CARTESIAN_POINT ( 'NONE',  ( 0.000000000000000000, 2.165354330708661568, 0.000000000000000000 ) ) ;
#49533=CARTESIAN_POINT ( 'NONE',  ( 0.5314960629921396951, 2.755905511811024056, -3.937007874015760578 ) ) ;
#49542=ORIENTED_EDGE ( 'NONE', *, *, #20457, .F. ) ;
#49558=ORIENTED_EDGE ( 'NONE', *, *, #82624, .T. ) ;
#49567=DIRECTION ( 'NONE',  ( 0.000000000000000000, 0.000000000000000000, -1.000000000000000000 ) ) ;
#49575=ORIENTED_EDGE ( 'NONE', *, *, #77389, .F. ) ;
#49578=VERTEX_POINT ( 'NONE', #30728 ) ;
#49607=CARTESIAN_POINT ( 'NONE',  ( 1.813482582612293559, 2.755905511811024056, 0.5314960629921260393 ) ) ;
#49642=VERTEX_POINT ( 'NONE', #12204 ) ;
#49655=CARTESIAN_POINT ( 'NONE',  ( -1.016821367227983552, 1.537401574803149984, -0.4744094488188975722 ) ) ;
#49657=ADVANCED_FACE ( 'NONE', ( #26059 ), #77845, .F. ) ;
#49692=CARTESIAN_POINT ( 'NONE',  ( 0.4744094488189011805, 1.553651517367183210, -1.016821367227981776 ) ) ;
#49695=CARTESIAN_POINT ( 'NONE',  ( -2.666390022512505453, 1.301092492065836659, -0.4123476441529835279 ) ) ;
#49698=CYLINDRICAL_SURFACE ( 'NONE', #35786, 0.4744094488188972947 ) ;
#49703=CARTESIAN_POINT ( 'NONE',  ( 0.000000000000000000, 2.755905511811024056, 0.000000000000000000 ) ) ;
#49719=CARTESIAN_POINT ( 'NONE',  ( -0.5314960629921294810, 2.559055118110236560, 0.9881811337016624952 ) ) ;
#49731=CARTESIAN_POINT ( 'NONE',  ( -3.937007874015748143, 2.559055118110236560, -0.5314960629921260393 ) ) ;
#49776=VERTEX_POINT ( 'NONE', #44985 ) ;
#49779=CARTESIAN_POINT ( 'NONE',  ( 1.141392835773559211, 0.3937007874015748254, 1.141392835773562764 ) ) ;
#49798=CARTESIAN_POINT ( 'NONE',  ( -3.911375737184146661, 1.694783778358343707, -0.4487029277117119963 ) ) ;
#49802=EDGE_CURVE ( 'NONE', #10785, #64866, #1818, .T. ) ;
#49811=AXIS2_PLACEMENT_3D ( 'NONE', #20500, #13774, #71849 ) ;
#49815=CARTESIAN_POINT ( 'NONE',  ( 2.575297182719591849, 1.629972608277045820, 0.4653577321740525186 ) ) ;
#49827=DIRECTION ( 'NONE',  ( 0.000000000000000000, -0.000000000000000000, 1.000000000000000000 ) ) ;
#49830=VECTOR ( 'NONE', #13517, 39.37007874015748143 ) ;
#49845=DIRECTION ( 'NONE',  ( 1.776356839400250465E-15, 0.000000000000000000, -1.000000000000000000 ) ) ;
#49868=AXIS2_PLACEMENT_3D ( 'NONE', #55871, #5370, #49567 ) ;
#49876=ORIENTED_EDGE ( 'NONE', *, *, #67320, .T. ) ;
#49883=CARTESIAN_POINT ( 'NONE',  ( -0.5314960629921148261, 2.742783305036532226, -3.197598447031737123 ) ) ;
#49890=AXIS2_PLACEMENT_3D ( 'NONE', #58817, #1174, #49278 ) ;
#49898=EDGE_CURVE ( 'NONE', #72873, #23049, #48604, .T. ) ;
#49901=ORIENTED_EDGE ( 'NONE', *, *, #41919, .T. ) ;
#49903=CARTESIAN_POINT ( 'NONE',  ( -0.4562955581495677371, 1.668131542012051494, 2.594245572444889625 ) ) ;
#49924=CARTESIAN_POINT ( 'NONE',  ( -3.900447471620230200, 2.687524476698323284, 0.5314960629921260393 ) ) ;
#49927=AXIS2_PLACEMENT_3D ( 'NONE', #59103, #65009, #32597 ) ;
#49940=CARTESIAN_POINT ( 'NONE',  ( 0.3334193678581618414, 1.199601195606732063, 2.750748997350709324 ) ) ;
#49953=ORIENTED_EDGE ( 'NONE', *, *, #24452, .T. ) ;
#49957=ADVANCED_FACE ( 'NONE', ( #1656 ), #20678, .T. ) ;
#49969=VERTEX_POINT ( 'NONE', #22250 ) ;
#49976=DIRECTION ( 'NONE',  ( 0.000000000000000000, -1.000000000000000000, 0.000000000000000000 ) ) ;
#49977=CARTESIAN_POINT ( 'NONE',  ( -0.4744094488188833059, 1.537401574803149984, -3.908320185825793658 ) ) ;
#49983=CARTESIAN_POINT ( 'NONE',  ( 3.910245801258434462, 1.413806224366693121, 0.4582898429536017004 ) ) ;
#49987=CARTESIAN_POINT ( 'NONE',  ( -0.5314960629921170465, 2.742779987576671186, -2.570293860457457225 ) ) ;
#49988=VERTEX_POINT ( 'NONE', #47908 ) ;
#49990=CIRCLE ( 'NONE', #16435, 0.1190944881889763746 ) ;
#49991=CARTESIAN_POINT ( 'NONE',  ( -1.033875059083676939, 1.724409448818897905, 0.4359958488159718093 ) ) ;
#50013=CARTESIAN_POINT ( 'NONE',  ( -2.159244633716660644, 1.469861850861823083, 0.4698711669589715201 ) ) ;
#50027=EDGE_CURVE ( 'NONE', #8695, #72978, #483, .T. ) ;
#50033=CARTESIAN_POINT ( 'NONE',  ( -3.926414575749307634, 1.160756069412853808, -0.2888700564287320360 ) ) ;
#50038=B_SPLINE_CURVE_WITH_KNOTS ( 'NONE', 3,
 ( #18732, #62524, #49883, #83122 ),
 .UNSPECIFIED., .F., .F.,
 ( 4, 4 ),
 ( 9.960895303349699888E-07, 0.001424104692945738371 ),
 .UNSPECIFIED. ) ;
#50042=CIRCLE ( 'NONE', #79654, 1.968503937007874072 ) ;
#50047=EDGE_CURVE ( 'NONE', #69251, #78176, #41604, .T. ) ;
#50050=CARTESIAN_POINT ( 'NONE',  ( 1.141392835773559211, 0.3937007874015748254, 0.8264322058523028147 ) ) ;
#50056=ORIENTED_EDGE ( 'NONE', *, *, #22073, .T. ) ;
#50071=VERTEX_POINT ( 'NONE', #4959 ) ;
#50100=CARTESIAN_POINT ( 'NONE',  ( -3.937007874015748143, 1.537401574803149984, 0.4744094488188970171 ) ) ;
#50103=CARTESIAN_POINT ( 'NONE',  ( -2.554854094587807101, 1.520093187801264900, 0.4741711390158121486 ) ) ;
#50120=DIRECTION ( 'NONE',  ( 0.000000000000000000, -1.000000000000000000, 0.000000000000000000 ) ) ;
#50125=CARTESIAN_POINT ( 'NONE',  ( 0.000000000000000000, 2.755905511811024056, 0.000000000000000000 ) ) ;
#50165=CARTESIAN_POINT ( 'NONE',  ( -0.3005662378122840872, 1.170051713876987920, -1.947704203106506604 ) ) ;
#50169=VERTEX_POINT ( 'NONE', #74433 ) ;
#50179=EDGE_CURVE ( 'NONE', #45807, #60543, #80349, .T. ) ;
#50185=ORIENTED_EDGE ( 'NONE', *, *, #42797, .T. ) ;
#50197=VECTOR ( 'NONE', #2019, 39.37007874015748143 ) ;
#50217=CARTESIAN_POINT ( 'NONE',  ( 0.6299212598425341092, 2.165354330708662012, -3.937007874015759690 ) ) ;
#50225=CARTESIAN_POINT ( 'NONE',  ( 2.594245572444920267, 1.668131542012050827, 0.4562955581495592994 ) ) ;
#50242=ORIENTED_EDGE ( 'NONE', *, *, #61206, .F. ) ;
#50246=CARTESIAN_POINT ( 'NONE',  ( -2.158884350236584204, 1.606100245667701598, -0.4697171261335985060 ) ) ;
#50255=DIRECTION ( 'NONE',  ( 0.000000000000000000, 1.000000000000000000, 0.000000000000000000 ) ) ;
#50256=CIRCLE ( 'NONE', #44886, 0.1771653543307085410 ) ;
#50285=ORIENTED_EDGE ( 'NONE', *, *, #19337, .T. ) ;
#50301=DIRECTION ( 'NONE',  ( 0.000000000000000000, 0.000000000000000000, -1.000000000000000000 ) ) ;
#50304=CARTESIAN_POINT ( 'NONE',  ( 2.158884350236621064, 1.606100245667702708, 0.4697171261335982284 ) ) ;
#50308=VERTEX_POINT ( 'NONE', #48321 ) ;
#50310=LINE ( 'NONE', #76418, #47902 ) ;
#50316=AXIS2_PLACEMENT_3D ( 'NONE', #19151, #41428, #48560 ) ;
#50328=VECTOR ( 'NONE', #59274, 39.37007874015748143 ) ;
#50348=CARTESIAN_POINT ( 'NONE',  ( 0.2406358745268415145, 1.128551111081926850, -1.544744577296102150 ) ) ;
#50355=EDGE_CURVE ( 'NONE', #54650, #60631, #22662, .T. ) ;
#50362=ORIENTED_EDGE ( 'NONE', *, *, #53188, .T. ) ;
#50363=EDGE_LOOP ( 'NONE', ( #6284, #3791, #59709, #25484, #17211, #60204, #70375, #48302, #38236, #52029 ) ) ;
#50364=EDGE_CURVE ( 'NONE', #78262, #50071, #15285, .T. ) ;
#50385=LINE ( 'NONE', #18825, #3923 ) ;
#50396=DIRECTION ( 'NONE',  ( -0.000000000000000000, 1.000000000000000000, -0.000000000000000000 ) ) ;
#50424=CARTESIAN_POINT ( 'NONE',  ( -0.3149606299212629468, -5.463695987328517809E-17, 1.076935383196056639 ) ) ;
#50428=CARTESIAN_POINT ( 'NONE',  ( -0.3149606299212459048, 2.559055118110236560, -3.937007874015763242 ) ) ;
#50436=AXIS2_PLACEMENT_3D ( 'NONE', #8126, #70845, #27469 ) ;
#50439=CARTESIAN_POINT ( 'NONE',  ( -3.937008591613926800, 1.062986170812217024, -0.01541001446542844891 ) ) ;
#50444=ORIENTED_EDGE ( 'NONE', *, *, #7531, .F. ) ;
#50454=DIRECTION ( 'NONE',  ( 8.673617379884035472E-16, 0.000000000000000000, -1.000000000000000000 ) ) ;
#50458=ORIENTED_EDGE ( 'NONE', *, *, #62746, .T. ) ;
#50460=ORIENTED_EDGE ( 'NONE', *, *, #72282, .T. ) ;
#50470=CARTESIAN_POINT ( 'NONE',  ( 0.4607143505782487214, 1.423150415408461544, -2.585258496787425919 ) ) ;
#50473=ORIENTED_EDGE ( 'NONE', *, *, #25974, .T. ) ;
#50475=VERTEX_POINT ( 'NONE', #30206 ) ;
#50477=DIRECTION ( 'NONE',  ( 0.000000000000000000, 0.000000000000000000, -1.000000000000000000 ) ) ;
#50488=EDGE_CURVE ( 'NONE', #34044, #49485, #39474, .T. ) ;
#50504=DIRECTION ( 'NONE',  ( -3.491481338843132961E-15, -0.000000000000000000, 1.000000000000000000 ) ) ;
#50506=DIRECTION ( 'NONE',  ( 0.000000000000000000, 0.000000000000000000, 1.000000000000000000 ) ) ;
#50509=CARTESIAN_POINT ( 'NONE',  ( -2.808613111760737802, 1.134406187872312843, -0.2508088161067581479 ) ) ;
#50526=CARTESIAN_POINT ( 'NONE',  ( 0.4725434569952585706, 1.494547573005087671, -2.165586928937583977 ) ) ;
#50531=AXIS2_PLACEMENT_3D ( 'NONE', #75913, #38420, #55702 ) ;
#50570=CARTESIAN_POINT ( 'NONE',  ( 0.000000000000000000, 2.165354330708661568, 0.000000000000000000 ) ) ;
#50571=CARTESIAN_POINT ( 'NONE',  ( 0.000000000000000000, 2.755905511811024056, 0.000000000000000000 ) ) ;
#50585=DIRECTION ( 'NONE',  ( 0.000000000000000000, 1.601283208593975810E-15, -1.000000000000000000 ) ) ;
#50590=ORIENTED_EDGE ( 'NONE', *, *, #76918, .F. ) ;
#50594=CIRCLE ( 'NONE', #37156, 0.2165354330708660069 ) ;
#50630=CARTESIAN_POINT ( 'NONE',  ( 1.028288428836420909, 1.383544431970676447, 0.4490413120122265789 ) ) ;
#50653=VECTOR ( 'NONE', #27347, 39.37007874015748143 ) ;
#50664=CARTESIAN_POINT ( 'NONE',  ( -0.2114499243052200550, 1.112441217203876676, 1.102030475220129535 ) ) ;
#50665=CARTESIAN_POINT ( 'NONE',  ( 3.264097702071373064, 2.755905511811024056, 0.5314960629921260393 ) ) ;
#50676=CARTESIAN_POINT ( 'NONE',  ( 1.141392835773559211, 0.3937007874015747699, 1.141392835773562764 ) ) ;
#50679=ADVANCED_FACE ( 'NONE', ( #37375 ), #43663, .F. ) ;
#50683=CARTESIAN_POINT ( 'NONE',  ( -0.5314960629921348101, 2.742784456114268909, 2.516666439024516144 ) ) ;
#50692=EDGE_CURVE ( 'NONE', #55882, #55851, #63678, .T. ) ;
#50695=ORIENTED_EDGE ( 'NONE', *, *, #60327, .T. ) ;
#50700=CARTESIAN_POINT ( 'NONE',  ( -0.3149606299212458493, 2.165354330708661568, -3.937007874015763242 ) ) ;
#50701=DIRECTION ( 'NONE',  ( 0.000000000000000000, -1.000000000000000000, -0.000000000000000000 ) ) ;
#50709=VERTEX_POINT ( 'NONE', #81598 ) ;
#50713=CARTESIAN_POINT ( 'NONE',  ( 0.000000000000000000, 2.755905511811024056, 0.000000000000000000 ) ) ;
#50715=TOROIDAL_SURFACE ( 'NONE', #33266, 3.858267716535433323, 0.07874015748031495954 ) ;
#50719=EDGE_LOOP ( 'NONE', ( #58118, #20506, #8178, #81664 ) ) ;
#50742=FACE_OUTER_BOUND ( 'NONE', #42784, .T. ) ;
#50760=CARTESIAN_POINT ( 'NONE',  ( 0.06791843738633827898, 1.067571514150120526, 2.869773448292317397 ) ) ;
#50774=VERTEX_POINT ( 'NONE', #42846 ) ;
#50786=VERTEX_POINT ( 'NONE', #49991 ) ;
#50788=ORIENTED_EDGE ( 'NONE', *, *, #30484, .T. ) ;
#50798=FACE_OUTER_BOUND ( 'NONE', #1345, .T. ) ;
#50804=ORIENTED_EDGE ( 'NONE', *, *, #62891, .F. ) ;
#50812=CARTESIAN_POINT ( 'NONE',  ( 1.813482582612293559, 2.755905511811024056, -0.5314960629921260393 ) ) ;
#50835=EDGE_CURVE ( 'NONE', #28101, #7205, #18042, .T. ) ;
#50842=DIRECTION ( 'NONE',  ( 0.000000000000000000, 0.000000000000000000, -1.000000000000000000 ) ) ;
#50866=CARTESIAN_POINT ( 'NONE',  ( -1.313877454013331780, 0.2929341459200028863, 0.8967544760595741460 ) ) ;
#50872=ORIENTED_EDGE ( 'NONE', *, *, #51075, .F. ) ;
#50913=B_SPLINE_CURVE_WITH_KNOTS ( 'NONE', 3,
 ( #25988, #70610, #62759, #11418, #64300, #32306, #51647, #81720, #57967, #38622, #29930, #12965, #30343, #42560, #45341, #42966, #334, #77351, #56424, #36256, #64717, #62333, #19683, #71037 ),
 .UNSPECIFIED., .F., .F.,
 ( 4, 2, 2, 2, 2, 2, 2, 2, 2, 2, 2, 4 ),
 ( 0.008892801244818756071, 0.009319797321957692601, 0.009746793399096627397, 0.01017378947623556393, 0.01060078555337450046, 0.01145477770765237005, 0.01230876986193024138, 0.01316276201620811097, 0.01401675417048598056, 0.01487074632476385189, 0.01529774240190278148, 0.01572473847904171107 ),
 .UNSPECIFIED. ) ;
#50917=CARTESIAN_POINT ( 'NONE',  ( -2.563288228875834296, 1.597527518877481123, -0.4706608522957235197 ) ) ;
#50934=CARTESIAN_POINT ( 'NONE',  ( 0.1685177960138025954, 1.093661989145994884, -1.109414537943555601 ) ) ;
#50936=B_SPLINE_CURVE_WITH_KNOTS ( 'NONE', 3,
 ( #48438, #3013, #16482, #60255 ),
 .UNSPECIFIED., .F., .F.,
 ( 4, 4 ),
 ( 0.2143416721067105124, 0.2157535705625736044 ),
 .UNSPECIFIED. ) ;
#50944=CARTESIAN_POINT ( 'NONE',  ( -0.07763836211493191364, 1.069131175596405026, -3.936271682215574330 ) ) ;
#50960=DIRECTION ( 'NONE',  ( 0.000000000000000000, 0.000000000000000000, 1.000000000000000000 ) ) ;
#50969=DIRECTION ( 'NONE',  ( 0.000000000000000000, 0.000000000000000000, -1.000000000000000000 ) ) ;
#50971=FACE_OUTER_BOUND ( 'NONE', #29805, .T. ) ;
#50984=ORIENTED_EDGE ( 'NONE', *, *, #65884, .F. ) ;
#50996=CARTESIAN_POINT ( 'NONE',  ( 3.908320185825791881, 1.537401574803149984, -0.4744094488188970171 ) ) ;
#51000=ORIENTED_EDGE ( 'NONE', *, *, #24627, .F. ) ;
#51026=CARTESIAN_POINT ( 'NONE',  ( -0.2639696576368211201, 1.142922413699642092, 1.923474121562456451 ) ) ;
#51031=DIRECTION ( 'NONE',  ( 0.000000000000000000, -1.000000000000000000, 0.000000000000000000 ) ) ;
#51045=LINE ( 'NONE', #43908, #78309 ) ;
#51075=EDGE_CURVE ( 'NONE', #66439, #53376, #63679, .T. ) ;
#51080=DIRECTION ( 'NONE',  ( -0.000000000000000000, -1.000000000000000000, -0.000000000000000000 ) ) ;
#51081=EDGE_CURVE ( 'NONE', #4880, #81379, #32836, .T. ) ;
#51098=ORIENTED_EDGE ( 'NONE', *, *, #27052, .F. ) ;
#51100=ORIENTED_EDGE ( 'NONE', *, *, #53209, .F. ) ;
#51114=ORIENTED_EDGE ( 'NONE', *, *, #48765, .F. ) ;
#51123=ORIENTED_EDGE ( 'NONE', *, *, #55596, .F. ) ;
#51124=ADVANCED_FACE ( 'NONE', ( #39997 ), #65259, .F. ) ;
#51138=EDGE_CURVE ( 'NONE', #16450, #35701, #80687, .T. ) ;
#51165=CARTESIAN_POINT ( 'NONE',  ( 0.3636368138136163997, 1.231320578257675713, 2.723393322692795770 ) ) ;
#51168=CIRCLE ( 'NONE', #61955, 0.09842519685039351207 ) ;
#51170=DIRECTION ( 'NONE',  ( -0.000000000000000000, -1.000000000000000000, -0.000000000000000000 ) ) ;
#51177=DIRECTION ( 'NONE',  ( 0.000000000000000000, 0.000000000000000000, -1.000000000000000000 ) ) ;
#51179=VERTEX_POINT ( 'NONE', #53845 ) ;
#51187=AXIS2_PLACEMENT_3D ( 'NONE', #19829, #45478, #80424 ) ;
#51204=DIRECTION ( 'NONE',  ( 1.000000000000000000, -0.000000000000000000, -0.000000000000000000 ) ) ;
#51210=EDGE_CURVE ( 'NONE', #44792, #22351, #36826, .T. ) ;
#51221=CARTESIAN_POINT ( 'NONE',  ( 2.077216372526538013, 1.325969025732677053, 0.4256800600601886586 ) ) ;
#51258=CARTESIAN_POINT ( 'NONE',  ( -3.921749386317083363, 1.212948189903745311, 0.3464575048171062432 ) ) ;
#51295=EDGE_LOOP ( 'NONE', ( #60954, #82186, #39919, #69363 ) ) ;
#51297=ORIENTED_EDGE ( 'NONE', *, *, #61511, .T. ) ;
#51302=EDGE_CURVE ( 'NONE', #11783, #74653, #70657, .T. ) ;
#51328=CARTESIAN_POINT ( 'NONE',  ( 2.362204724409448620, 1.724409448818897461, 8.247593713802677664E-15 ) ) ;
#51331=DIRECTION ( 'NONE',  ( -0.000000000000000000, 1.000000000000000000, -0.000000000000000000 ) ) ;
#51344=CARTESIAN_POINT ( 'NONE',  ( 0.3149606299212184268, 2.559055118110236560, 3.937007874015792552 ) ) ;
#51354=CARTESIAN_POINT ( 'NONE',  ( -0.2101277439827862470, 1.111780837440068392, -3.931420396975905174 ) ) ;
#51367=DIRECTION ( 'NONE',  ( 0.000000000000000000, 0.000000000000000000, -1.000000000000000000 ) ) ;
#51378=VERTEX_POINT ( 'NONE', #16406 ) ;
#51381=CARTESIAN_POINT ( 'NONE',  ( -0.03443470937339728616, 0.2755905511811023723, -1.537015892239756099 ) ) ;
#51390=EDGE_CURVE ( 'NONE', #66675, #42693, #36526, .T. ) ;
#51392=DIRECTION ( 'NONE',  ( 0.000000000000000000, -1.000000000000000000, 0.000000000000000000 ) ) ;
#51393=CARTESIAN_POINT ( 'NONE',  ( -0.4607143505782321236, 1.423150415408463987, -2.139150952031436237 ) ) ;
#51397=VERTEX_POINT ( 'NONE', #12144 ) ;
#51411=DIRECTION ( 'NONE',  ( 0.000000000000000000, -1.601283208593975810E-15, -1.000000000000000000 ) ) ;
#51413=CARTESIAN_POINT ( 'NONE',  ( 3.909774025758389726, 1.429695482061029477, -0.4622850232133952075 ) ) ;
#51414=VERTEX_POINT ( 'NONE', #24752 ) ;
#51415=VERTEX_POINT ( 'NONE', #63479 ) ;
#51419=CARTESIAN_POINT ( 'NONE',  ( 0.5314960629921325896, 2.729653106663536555, -1.868118594278512345 ) ) ;
#51453=CARTESIAN_POINT ( 'NONE',  ( 1.087350715983457228, 1.152082538880340179, 0.2771893343846333901 ) ) ;
#51492=DIRECTION ( 'NONE',  ( 0.000000000000000000, 0.000000000000000000, -1.000000000000000000 ) ) ;
#51501=CIRCLE ( 'NONE', #15271, 3.937007874015748143 ) ;
#51511=EDGE_LOOP ( 'NONE', ( #70472, #40769, #71820, #63747 ) ) ;
#51516=CYLINDRICAL_SURFACE ( 'NONE', #33030, 0.5118110236220472231 ) ;
#51527=EDGE_CURVE ( 'NONE', #64262, #53376, #52621, .T. ) ;
#51528=CARTESIAN_POINT ( 'NONE',  ( -1.115285832841460767, 1.079194095246727603, -0.1239054779398514883 ) ) ;
#51536=CARTESIAN_POINT ( 'NONE',  ( -0.03443470937339728616, 0.2755905511811023723, -1.753551325310622078 ) ) ;
#51550=ADVANCED_FACE ( 'NONE', ( #17642 ), #28782, .T. ) ;
#51564=VERTEX_POINT ( 'NONE', #82843 ) ;
#51577=AXIS2_PLACEMENT_3D ( 'NONE', #8868, #73689, #34546 ) ;
#51579=CARTESIAN_POINT ( 'NONE',  ( 0.3534909051124875967, 1.220709699003109217, -1.724520491472795847 ) ) ;
#51592=VERTEX_POINT ( 'NONE', #62239 ) ;
#51618=FACE_OUTER_BOUND ( 'NONE', #34278, .T. ) ;
#51626=EDGE_LOOP ( 'NONE', ( #53657, #68428, #71735, #53783, #38168, #47302 ) ) ;
#51633=CARTESIAN_POINT ( 'NONE',  ( 1.877095671717799341, 1.091897865355351271, 0.1662078246829481742 ) ) ;
#51643=VECTOR ( 'NONE', #10238, 39.37007874015748143 ) ;
#51647=CARTESIAN_POINT ( 'NONE',  ( -0.07506541128662616580, 1.068950050010701203, -1.458193486491603741 ) ) ;
#51655=B_SPLINE_CURVE_WITH_KNOTS ( 'NONE', 3,
 ( #71745, #72576, #1052, #1876, #14923, #15342, #27952, #26706 ),
 .UNSPECIFIED., .F., .F.,
 ( 4, 2, 2, 4 ),
 ( 0.05656618697110752519, 0.05899478853696744213, 0.06020908931989741447, 0.06142339010282737988 ),
 .UNSPECIFIED. ) ;
#51660=DIRECTION ( 'NONE',  ( 9.381338752702771457E-17, -0.6427876096865352551, 0.7660444431189814551 ) ) ;
#51680=CARTESIAN_POINT ( 'NONE',  ( -0.4744094488189005698, 1.553452312607695118, 1.016821367227982442 ) ) ;
#51696=ORIENTED_EDGE ( 'NONE', *, *, #40336, .T. ) ;
#51699=ORIENTED_EDGE ( 'NONE', *, *, #39798, .T. ) ;
#51718=CARTESIAN_POINT ( 'NONE',  ( 0.6299212598425341092, 2.165354330708662012, -3.937007874015759690 ) ) ;
#51722=EDGE_CURVE ( 'NONE', #52853, #34044, #71278, .T. ) ;
#51789=DIRECTION ( 'NONE',  ( 1.000000000000000000, -0.000000000000000000, -0.000000000000000000 ) ) ;
#51794=CARTESIAN_POINT ( 'NONE',  ( 0.5314960629921294810, 0.000000000000000000, -0.9881811337016621621 ) ) ;
#51798=ORIENTED_EDGE ( 'NONE', *, *, #28945, .F. ) ;
#51801=ORIENTED_EDGE ( 'NONE', *, *, #57736, .T. ) ;
#51805=CARTESIAN_POINT ( 'NONE',  ( 0.000000000000000000, 0.000000000000000000, 0.000000000000000000 ) ) ;
#51807=CARTESIAN_POINT ( 'NONE',  ( -3.937007874015748143, 1.724409448818897905, 0.6299212598425196763 ) ) ;
#51834=CARTESIAN_POINT ( 'NONE',  ( -0.5314960629921393620, 2.755905511811024056, 3.821484228344191880 ) ) ;
#51837=PLANE ( 'NONE',  #40204 ) ;
#51838=ORIENTED_EDGE ( 'NONE', *, *, #19393, .F. ) ;
#51843=CARTESIAN_POINT ( 'NONE',  ( 0.5314960629921324786, 2.716535433070866645, -1.854472803289050509 ) ) ;
#51856=DIRECTION ( 'NONE',  ( 0.000000000000000000, 0.000000000000000000, 1.000000000000000000 ) ) ;
#51862=CIRCLE ( 'NONE', #19603, 0.1771653543307085410 ) ;
#51863=TOROIDAL_SURFACE ( 'NONE', #42444, 3.858267716535433323, 0.07874015748031495954 ) ;
#51866=LINE ( 'NONE', #59033, #32141 ) ;
#51876=CARTESIAN_POINT ( 'NONE',  ( 1.057016155527769508, 1.247622337477865440, -0.3768861415345499677 ) ) ;
#51879=CIRCLE ( 'NONE', #53205, 0.3149606299212598381 ) ;
#51887=CARTESIAN_POINT ( 'NONE',  ( 0.6299212598425341092, 1.724409448818898127, -3.937007874015759690 ) ) ;
#51903=CARTESIAN_POINT ( 'NONE',  ( 0.000000000000000000, 2.755905511811024056, 0.000000000000000000 ) ) ;
#51913=DIRECTION ( 'NONE',  ( 0.8660254037844361541, 0.000000000000000000, 0.5000000000000043299 ) ) ;
#51917=AXIS2_PLACEMENT_3D ( 'NONE', #68218, #23573, #28659 ) ;
#51938=AXIS2_PLACEMENT_3D ( 'NONE', #69780, #25144, #23502 ) ;
#51940=CARTESIAN_POINT ( 'NONE',  ( -0.08520949344212035148, 1.070405622666591228, 2.867149795802078849 ) ) ;
#51941=DIRECTION ( 'NONE',  ( -0.000000000000000000, 1.000000000000000000, 0.000000000000000000 ) ) ;
#51949=DIRECTION ( 'NONE',  ( 0.000000000000000000, 0.000000000000000000, -1.000000000000000000 ) ) ;
#51951=LINE ( 'NONE', #635, #37112 ) ;
#51952=CARTESIAN_POINT ( 'NONE',  ( -0.03443470937339728616, 0.2755905511811023723, -1.656110380428732265 ) ) ;
#51971=EDGE_CURVE ( 'NONE', #79084, #63914, #55616, .T. ) ;
#51973=CIRCLE ( 'NONE', #22450, 1.929133858267716661 ) ;
#51975=VECTOR ( 'NONE', #64142, 39.37007874015749564 ) ;
#52002=CARTESIAN_POINT ( 'NONE',  ( 1.016821367227983552, 1.537401574803149984, 0.4744094488188975722 ) ) ;
#52014=ORIENTED_EDGE ( 'NONE', *, *, #61781, .F. ) ;
#52021=DIRECTION ( 'NONE',  ( 1.047444401652940007E-14, -0.000000000000000000, -1.000000000000000000 ) ) ;
#52029=ORIENTED_EDGE ( 'NONE', *, *, #40826, .F. ) ;
#52049=EDGE_LOOP ( 'NONE', ( #34698, #8263, #11717, #20171 ) ) ;
#52056=CARTESIAN_POINT ( 'NONE',  ( 1.939486441909066494, 1.160811571118570695, 0.2889173282905437290 ) ) ;
#52093=CIRCLE ( 'NONE', #64246, 0.5118110236220471121 ) ;
#52096=DIRECTION ( 'NONE',  ( 0.000000000000000000, 0.000000000000000000, -1.000000000000000000 ) ) ;
#52113=CARTESIAN_POINT ( 'NONE',  ( 0.2372349296589321144, 1.126275035012231918, -3.929877705396449539 ) ) ;
#52117=ORIENTED_EDGE ( 'NONE', *, *, #51302, .T. ) ;
#52130=EDGE_CURVE ( 'NONE', #38353, #81379, #30094, .T. ) ;
#52133=ORIENTED_EDGE ( 'NONE', *, *, #16548, .T. ) ;
#52145=CARTESIAN_POINT ( 'NONE',  ( 0.5314960629921349211, 2.716535433070866645, -2.543486866223387377 ) ) ;
#52154=B_SPLINE_CURVE_WITH_KNOTS ( 'NONE', 3,
 ( #83121, #30938, #36850, #10776 ),
 .UNSPECIFIED., .F., .F.,
 ( 4, 4 ),
 ( 0.2172790356422210356, 0.2186919052326019575 ),
 .UNSPECIFIED. ) ;
#52173=CARTESIAN_POINT ( 'NONE',  ( -0.03443470937339728616, 0.2755905511811023723, -1.656110380428732265 ) ) ;
#52190=EDGE_CURVE ( 'NONE', #58992, #28368, #6414, .T. ) ;
#52198=CARTESIAN_POINT ( 'NONE',  ( 0.4744094488189052328, 1.537401574803149984, -2.170146923806634653 ) ) ;
#52205=ORIENTED_EDGE ( 'NONE', *, *, #49228, .T. ) ;
#52221=ORIENTED_EDGE ( 'NONE', *, *, #17674, .T. ) ;
#52228=DIRECTION ( 'NONE',  ( 0.000000000000000000, 0.000000000000000000, -1.000000000000000000 ) ) ;
#52239=ORIENTED_EDGE ( 'NONE', *, *, #24452, .F. ) ;
#52255=CARTESIAN_POINT ( 'NONE',  ( -0.5314960629921197111, 2.755905511811024056, -1.813482582612295557 ) ) ;
#52265=EDGE_CURVE ( 'NONE', #30219, #29058, #20743, .T. ) ;
#52269=DIRECTION ( 'NONE',  ( 0.000000000000000000, -1.000000000000000000, 0.000000000000000000 ) ) ;
#52284=DIRECTION ( 'NONE',  ( 0.000000000000000000, -1.460819769243627131E-15, -1.000000000000000000 ) ) ;
#52295=CARTESIAN_POINT ( 'NONE',  ( 1.018615313942585976, 1.475001671837482542, -0.4705483627597061846 ) ) ;
#52298=CARTESIAN_POINT ( 'NONE',  ( 0.2098209183887521645, 1.111631239983235098, 3.931436657694179715 ) ) ;
#52304=LINE ( 'NONE', #52721, #78938 ) ;
#52322=DIRECTION ( 'NONE',  ( -0.000000000000000000, -1.000000000000000000, -0.000000000000000000 ) ) ;
#52332=CARTESIAN_POINT ( 'NONE',  ( 0.3568790343112974717, 1.224452473450301060, 1.063829662821178745 ) ) ;
#52352=ORIENTED_EDGE ( 'NONE', *, *, #67169, .F. ) ;
#52356=CARTESIAN_POINT ( 'NONE',  ( -0.06850640440391347896, 1.067651707476379830, 2.869699202025107532 ) ) ;
#52357=CARTESIAN_POINT ( 'NONE',  ( -0.4744094488188880798, 1.537401574803149984, -2.554262525012305218 ) ) ;
#52373=FACE_OUTER_BOUND ( 'NONE', #47707, .T. ) ;
#52374=CARTESIAN_POINT ( 'NONE',  ( 4.218763579739897660E-16, 0.000000000000000000, 3.444881889763779625 ) ) ;
#52417=LINE ( 'NONE', #13314, #69482 ) ;
#52428=DIRECTION ( 'NONE',  ( 0.000000000000000000, 1.000000000000000000, 0.000000000000000000 ) ) ;
#52429=ORIENTED_EDGE ( 'NONE', *, *, #64406, .F. ) ;
#52430=ORIENTED_EDGE ( 'NONE', *, *, #41383, .F. ) ;
#52432=CIRCLE ( 'NONE', #49927, 0.5118110236220472231 ) ;
#52442=EDGE_CURVE ( 'NONE', #74617, #24203, #32801, .T. ) ;
#52446=ORIENTED_EDGE ( 'NONE', *, *, #25189, .T. ) ;
#52456=B_SPLINE_CURVE_WITH_KNOTS ( 'NONE', 3,
 ( #39929, #65618, #73585, #59687, #3698, #35268, #48298, #9189 ),
 .UNSPECIFIED., .F., .F.,
 ( 4, 2, 2, 4 ),
 ( 0.000000000000000000, 0.002428728328773748467, 0.003643092493160610991, 0.004857456657547474382 ),
 .UNSPECIFIED. ) ;
#52475=CARTESIAN_POINT ( 'NONE',  ( 1.392101432702376629, 0.1377952755905511861, 0.9507481457704560768 ) ) ;
#52483=LINE ( 'NONE', #1585, #6206 ) ;
#52500=CARTESIAN_POINT ( 'NONE',  ( -1.019868997598491145, 1.617710314158373519, -0.4678352644680017214 ) ) ;
#52506=CARTESIAN_POINT ( 'NONE',  ( 0.000000000000000000, 2.755905511811024056, 0.000000000000000000 ) ) ;
#52508=VECTOR ( 'NONE', #4135, 39.37007874015748143 ) ;
#52525=CARTESIAN_POINT ( 'NONE',  ( 0.4724922890202770676, 1.580837543196284223, -2.558946168779563823 ) ) ;
#52534=DIRECTION ( 'NONE',  ( 0.000000000000000000, 0.000000000000000000, 1.000000000000000000 ) ) ;
#52556=CARTESIAN_POINT ( 'NONE',  ( 2.558801921129982837, 1.494646310179101878, 0.4725519687354816090 ) ) ;
#52586=CONICAL_SURFACE ( 'NONE', #28390, 1.244489337948955221, 0.7853981633974452814 ) ;
#52591=CARTESIAN_POINT ( 'NONE',  ( 3.224202737261815166, 2.716535433070866645, 0.5314960629921260393 ) ) ;
#52596=ADVANCED_FACE ( 'NONE', ( #79181 ), #79879, .T. ) ;
#52621=B_SPLINE_CURVE_WITH_KNOTS ( 'NONE', 3,
 ( #44105, #5407, #82030, #56331 ),
 .UNSPECIFIED., .F., .F.,
 ( 4, 4 ),
 ( 0.1331161126011577434, 0.1345277053022641001 ),
 .UNSPECIFIED. ) ;
#52628=CIRCLE ( 'NONE', #57970, 0.09842519685039351207 ) ;
#52632=LINE ( 'NONE', #20246, #6815 ) ;
#52633=CARTESIAN_POINT ( 'NONE',  ( 0.6299212598425100174, 1.724409448818897905, 0.9285414500055780840 ) ) ;
#52644=EDGE_LOOP ( 'NONE', ( #36520, #60758, #2896, #82886 ) ) ;
#52655=DIRECTION ( 'NONE',  ( 0.000000000000000000, 0.000000000000000000, 1.000000000000000000 ) ) ;
#52658=VERTEX_POINT ( 'NONE', #54721 ) ;
#52673=PLANE ( 'NONE',  #53372 ) ;
#52676=CARTESIAN_POINT ( 'NONE',  ( 3.918940769308645322, 1.247921457474008511, -0.3771434222490559485 ) ) ;
#52680=CARTESIAN_POINT ( 'NONE',  ( -1.854472803289052507, 2.716535433070866645, -0.5314960629921260393 ) ) ;
#52692=AXIS2_PLACEMENT_3D ( 'NONE', #3066, #16953, #49321 ) ;
#52701=DIRECTION ( 'NONE',  ( 0.000000000000000000, 0.000000000000000000, 1.000000000000000000 ) ) ;
#52715=CARTESIAN_POINT ( 'NONE',  ( 0.3858508372531669339, 1.260953067117916326, 3.918063942240381792 ) ) ;
#52721=CARTESIAN_POINT ( 'NONE',  ( 3.937007874015748143, 1.537401574803149984, 0.4744094488188975722 ) ) ;
#52727=B_SPLINE_CURVE_WITH_KNOTS ( 'NONE', 3,
 ( #59261, #60099, #39491, #45786 ),
 .UNSPECIFIED., .F., .F.,
 ( 4, 4 ),
 ( 2.857347768991906607E-07, 0.001436604392377180406 ),
 .UNSPECIFIED. ) ;
#52742=EDGE_CURVE ( 'NONE', #39419, #15857, #40860, .T. ) ;
#52746=AXIS2_PLACEMENT_3D ( 'NONE', #74608, #49320, #10630 ) ;
#52769=EDGE_CURVE ( 'NONE', #40470, #12202, #43535, .T. ) ;
#52777=CARTESIAN_POINT ( 'NONE',  ( -0.3234312996134343088, 1.189126250296157261, 2.759783988742167349 ) ) ;
#52780=EDGE_CURVE ( 'NONE', #70804, #29875, #47571, .T. ) ;
#52782=FACE_OUTER_BOUND ( 'NONE', #4711, .T. ) ;
#52790=DIRECTION ( 'NONE',  ( 0.000000000000000000, 0.000000000000000000, 1.000000000000000000 ) ) ;
#52820=CARTESIAN_POINT ( 'NONE',  ( 1.524059884292195765E-16, 0.04488074079120789317, 1.244489337948954555 ) ) ;
#52837=ADVANCED_FACE ( 'NONE', ( #3387 ), #34961, .F. ) ;
#52853=VERTEX_POINT ( 'NONE', #28640 ) ;
#52854=AXIS2_PLACEMENT_3D ( 'NONE', #5431, #11766, #44532 ) ;
#52859=CARTESIAN_POINT ( 'NONE',  ( 0.000000000000000000, 0.000000000000000000, 0.000000000000000000 ) ) ;
#52870=ORIENTED_EDGE ( 'NONE', *, *, #76757, .T. ) ;
#52880=CARTESIAN_POINT ( 'NONE',  ( 0.4417575354491365958, 1.710976477253062233, 2.103512204792471252 ) ) ;
#52887=VERTEX_POINT ( 'NONE', #48397 ) ;
#52892=CARTESIAN_POINT ( 'NONE',  ( 1.973869084197717116, 1.199841186584411190, 0.3336616047370207783 ) ) ;
#52914=CARTESIAN_POINT ( 'NONE',  ( -0.4744094488188934089, 1.537401574803149984, -1.016821367227985551 ) ) ;
#52916=DIRECTION ( 'NONE',  ( -0.000000000000000000, -1.000000000000000000, -0.000000000000000000 ) ) ;
#52923=DIRECTION ( 'NONE',  ( 0.000000000000000000, 0.000000000000000000, -1.000000000000000000 ) ) ;
#52939=LINE ( 'NONE', #46216, #8252 ) ;
#52951=ORIENTED_EDGE ( 'NONE', *, *, #70822, .T. ) ;
#52972=CARTESIAN_POINT ( 'NONE',  ( -1.424355216557543713, 1.172051041393591619, 0.3026866195246171176 ) ) ;
#52977=VECTOR ( 'NONE', #11356, 39.37007874015748143 ) ;
#52985=CARTESIAN_POINT ( 'NONE',  ( -2.565525098582201124, 1.606100245667705373, 0.4697171261335973402 ) ) ;
#53012=CARTESIAN_POINT ( 'NONE',  ( -0.5314960629921124946, 2.687524476698321507, -3.900447471620232864 ) ) ;
#53021=VECTOR ( 'NONE', #21122, 39.37007874015748143 ) ;
#53023=CARTESIAN_POINT ( 'NONE',  ( 6.265965269058076312E-17, 1.062992125984252745, -1.850393700787401619 ) ) ;
#53039=VERTEX_POINT ( 'NONE', #50866 ) ;
#53043=FACE_OUTER_BOUND ( 'NONE', #47806, .T. ) ;
#53045=CARTESIAN_POINT ( 'NONE',  ( -1.854472803289052507, 2.716535433070866645, 0.5314960629921260393 ) ) ;
#53056=EDGE_LOOP ( 'NONE', ( #1327, #58445 ) ) ;
#53064=EDGE_CURVE ( 'NONE', #51397, #10785, #18495, .T. ) ;
#53071=CARTESIAN_POINT ( 'NONE',  ( 0.000000000000000000, 2.559055118110236560, 0.000000000000000000 ) ) ;
#53072=ORIENTED_EDGE ( 'NONE', *, *, #26135, .T. ) ;
#53091=CARTESIAN_POINT ( 'NONE',  ( 3.931468625396333572, 1.111233271792932520, -0.2107404457489559235 ) ) ;
#53100=CIRCLE ( 'NONE', #15466, 0.5118110236220471121 ) ;
#53103=DIRECTION ( 'NONE',  ( 0.000000000000000000, 0.000000000000000000, -1.000000000000000000 ) ) ;
#53112=FACE_OUTER_BOUND ( 'NONE', #45286, .T. ) ;
#53121=CARTESIAN_POINT ( 'NONE',  ( -0.4670403427556097387, 1.622209144264169289, 2.152711368484138355 ) ) ;
#53130=CARTESIAN_POINT ( 'NONE',  ( 0.4622690493055590655, 1.429647347090970522, 3.909775897616574181 ) ) ;
#53153=CARTESIAN_POINT ( 'NONE',  ( 3.831929248781927200, 2.755905511811024056, -0.5314960629921259283 ) ) ;
#53159=B_SPLINE_CURVE_WITH_KNOTS ( 'NONE', 3,
 ( #43379, #29939, #63583, #75000, #30353, #69495, #5105, #56022, #75814, #69079, #11430, #5917, #11844, #57246, #63172, #81730, #56433, #24449, #25268, #50934, #24855, #44611, #17346, #42974, #68670, #18157 ),
 .UNSPECIFIED., .F., .F.,
 ( 4, 2, 2, 2, 2, 2, 2, 2, 2, 2, 2, 2, 4 ),
 ( 0.000000000000000000, 0.002383650122917511851, 0.003575475184376268861, 0.004767300245835024569, 0.007150950368752538588, 0.008342775430211293863, 0.009534600491670042199, 0.01072642555312879054, 0.01191825061458753714, 0.01430190073750502340, 0.01549372579896377000, 0.01668555086042251834, 0.01906920098334001501 ),
 .UNSPECIFIED. ) ;
#53164=CARTESIAN_POINT ( 'NONE',  ( 0.3466100433291510186, 1.213118387047130264, 1.067229880606827885 ) ) ;
#53181=ORIENTED_EDGE ( 'NONE', *, *, #23955, .T. ) ;
#53183=EDGE_LOOP ( 'NONE', ( #12595, #63521, #15551, #50473 ) ) ;
#53188=EDGE_CURVE ( 'NONE', #64046, #41865, #69830, .T. ) ;
#53190=DIRECTION ( 'NONE',  ( 0.000000000000000000, 1.000000000000000000, -0.000000000000000000 ) ) ;
#53198=CARTESIAN_POINT ( 'NONE',  ( -1.084166635437626258, 1.161135222542148071, -0.2893535460047377272 ) ) ;
#53205=AXIS2_PLACEMENT_3D ( 'NONE', #29603, #16583, #80153 ) ;
#53206=ORIENTED_EDGE ( 'NONE', *, *, #29099, .F. ) ;
#53209=EDGE_CURVE ( 'NONE', #30609, #51397, #63731, .T. ) ;
#53218=EDGE_CURVE ( 'NONE', #53039, #17115, #36594, .T. ) ;
#53235=DIRECTION ( 'NONE',  ( 0.000000000000000000, -1.000000000000000000, 0.000000000000000000 ) ) ;
#53241=EDGE_CURVE ( 'NONE', #13252, #59983, #24790, .T. ) ;
#53257=ADVANCED_FACE ( 'NONE', ( #43720 ), #8663, .F. ) ;
#53259=CARTESIAN_POINT ( 'NONE',  ( 0.4732185887570711236, 1.572090529166663364, 2.557182324916609240 ) ) ;
#53265=ADVANCED_FACE ( 'NONE', ( #74929, #68597 ), #31521, .F. ) ;
#53272=VERTEX_POINT ( 'NONE', #30702 ) ;
#53278=CARTESIAN_POINT ( 'NONE',  ( -3.900966923095589678, 2.559055118110236560, 0.5314960629921260393 ) ) ;
#53289=ORIENTED_EDGE ( 'NONE', *, *, #83098, .T. ) ;
#53290=LINE ( 'NONE', #48641, #59697 ) ;
#53306=ORIENTED_EDGE ( 'NONE', *, *, #81602, .T. ) ;
#53318=AXIS2_PLACEMENT_3D ( 'NONE', #32222, #57880, #19592 ) ;
#53323=EDGE_CURVE ( 'NONE', #58782, #12593, #37430, .T. ) ;
#53340=CARTESIAN_POINT ( 'NONE',  ( 0.4323985109340933719, 1.341647856265051564, -1.452992989815209190 ) ) ;
#53348=DIRECTION ( 'NONE',  ( 0.000000000000000000, 0.000000000000000000, 1.000000000000000000 ) ) ;
#53356=CARTESIAN_POINT ( 'NONE',  ( -3.909054398717938028, 1.460102366761165449, -0.4683312780462470237 ) ) ;
#53363=CARTESIAN_POINT ( 'NONE',  ( 0.4602855208775837870, 1.653389129435537175, -2.586148212265404922 ) ) ;
#53370=CARTESIAN_POINT ( 'NONE',  ( 3.937007874015748143, 2.165354330708661568, 0.3149606299212600047 ) ) ;
#53372=AXIS2_PLACEMENT_3D ( 'NONE', #58580, #14414, #53512 ) ;
#53376=VERTEX_POINT ( 'NONE', #81659 ) ;
#53393=VERTEX_POINT ( 'NONE', #42494 ) ;
#53405=DIRECTION ( 'NONE',  ( 1.000000000000000000, -1.734723475976808080E-16, 1.047444401652940007E-14 ) ) ;
#53424=ADVANCED_FACE ( 'NONE', ( #69005 ), #37014, .T. ) ;
#53437=CARTESIAN_POINT ( 'NONE',  ( 0.5314960629920854052, 2.746034003362845866, 3.861376881555345086 ) ) ;
#53455=CARTESIAN_POINT ( 'NONE',  ( -1.313877454013331780, 1.062992125984252079, 0.7983292792091805090 ) ) ;
#53462=EDGE_LOOP ( 'NONE', ( #43138, #73181, #7660, #48817 ) ) ;
#53494=ORIENTED_EDGE ( 'NONE', *, *, #54568, .F. ) ;
#53498=AXIS2_PLACEMENT_3D ( 'NONE', #42072, #74912, #23130 ) ;
#53512=DIRECTION ( 'NONE',  ( 0.000000000000000000, -0.000000000000000000, -1.000000000000000000 ) ) ;
#53515=CARTESIAN_POINT ( 'NONE',  ( 3.924581109467853324, 1.180375947577095408, 0.3127951191726855429 ) ) ;
#53538=DIRECTION ( 'NONE',  ( -0.000000000000000000, 1.000000000000000000, -1.408710688920637755E-15 ) ) ;
#53557=CARTESIAN_POINT ( 'NONE',  ( -3.937007874015748143, 2.755905511811024056, -0.5314960629921260393 ) ) ;
#53572=ORIENTED_EDGE ( 'NONE', *, *, #16744, .F. ) ;
#53574=CARTESIAN_POINT ( 'NONE',  ( 3.881246834694716874, 2.729333734409945755, -0.5314960629921260393 ) ) ;
#53583=CARTESIAN_POINT ( 'NONE',  ( 0.3763565203970011264, 1.248168874848284426, 1.057096006133714017 ) ) ;
#53604=B_SPLINE_CURVE_WITH_KNOTS ( 'NONE', 3,
 ( #57655, #13479, #17, #52591 ),
 .UNSPECIFIED., .F., .F.,
 ( 4, 4 ),
 ( 0.1795298335526531730, 0.1809577925700029677 ),
 .UNSPECIFIED. ) ;
#53607=CARTESIAN_POINT ( 'NONE',  ( 0.000000000000000000, 2.559055118110236560, 0.000000000000000000 ) ) ;
#53609=DIRECTION ( 'NONE',  ( 0.000000000000000000, 0.000000000000000000, -1.000000000000000000 ) ) ;
#53614=VERTEX_POINT ( 'NONE', #69422 ) ;
#53616=CARTESIAN_POINT ( 'NONE',  ( -1.116870163894023937, 1.075361400900961550, 0.1087570619416485251 ) ) ;
#53625=DIRECTION ( 'NONE',  ( -0.000000000000000000, -1.000000000000000000, -1.408710688920637755E-15 ) ) ;
#53657=ORIENTED_EDGE ( 'NONE', *, *, #78852, .F. ) ;
#53682=ORIENTED_EDGE ( 'NONE', *, *, #40727, .F. ) ;
#53701=ORIENTED_EDGE ( 'NONE', *, *, #83060, .T. ) ;
#53702=CARTESIAN_POINT ( 'NONE',  ( -1.481587895432891600, 1.357470117436001766, 0.4390532657067846012 ) ) ;
#53710=CARTESIAN_POINT ( 'NONE',  ( -0.4744094488188894121, 1.537401574803149984, -2.170146923806595574 ) ) ;
#53718=ORIENTED_EDGE ( 'NONE', *, *, #71221, .F. ) ;
#53723=EDGE_CURVE ( 'NONE', #19150, #79281, #6259, .T. ) ;
#53724=CARTESIAN_POINT ( 'NONE',  ( 1.850419646634101412, 1.063020117359137373, 0.01785754392580130370 ) ) ;
#53747=CARTESIAN_POINT ( 'NONE',  ( 0.000000000000000000, 2.559055118110236560, 0.000000000000000000 ) ) ;
#53753=CARTESIAN_POINT ( 'NONE',  ( 0.5314960629921396951, 2.559055118110236560, -3.937007874015760578 ) ) ;
#53771=B_SPLINE_CURVE_WITH_KNOTS ( 'NONE', 3,
 ( #67777, #16437, #12069, #76862, #36906, #11248, #62582, #12476, #31825, #37726, #76046, #6151, #18390, #83179, #51165, #49940, #17977, #37324, #56661, #5735, #41671, #35366, #54714, #4924, #30592, #69724, #50760, #31407, #57071, #18787 ),
 .UNSPECIFIED., .F., .F.,
 ( 4, 2, 2, 2, 2, 2, 2, 2, 2, 2, 2, 2, 2, 2, 4 ),
 ( 0.01323639539072356958, 0.01388240907739069462, 0.01452842276405781965, 0.01582045013739205239, 0.01711247751072628165, 0.01840450488406051438, 0.02098855963072899372, 0.02357261437739747306, 0.02486464175073171967, 0.02615666912406597669, 0.02744869649740022677, 0.02874072387073448032, 0.03132477861740298741, 0.03261680599073724096, 0.03390883336407149451 ),
 .UNSPECIFIED. ) ;
#53781=ORIENTED_EDGE ( 'NONE', *, *, #2120, .T. ) ;
#53783=ORIENTED_EDGE ( 'NONE', *, *, #1707, .F. ) ;
#53798=ORIENTED_EDGE ( 'NONE', *, *, #56208, .F. ) ;
#53803=CARTESIAN_POINT ( 'NONE',  ( 2.666390022512479696, 1.301092492065843320, 0.4123476441529870806 ) ) ;
#53809=CARTESIAN_POINT ( 'NONE',  ( 1.348312163386739426, 0.2755905511811023723, 0.7386866130305692613 ) ) ;
#53816=DIRECTION ( 'NONE',  ( 0.000000000000000000, -0.000000000000000000, 1.000000000000000000 ) ) ;
#53845=CARTESIAN_POINT ( 'NONE',  ( 3.184294706754630777, 2.755905511811024056, 0.5314960629921260393 ) ) ;
#53855=AXIS2_PLACEMENT_3D ( 'NONE', #12586, #36591, #30278 ) ;
#53864=DIRECTION ( 'NONE',  ( -1.000000000000000000, -0.000000000000000000, -0.000000000000000000 ) ) ;
#53870=CARTESIAN_POINT ( 'NONE',  ( -2.362204724409448620, 0.03937007874015751446, -2.474278114140802984E-14 ) ) ;
#53871=EDGE_LOOP ( 'NONE', ( #42909, #28577, #22318, #39403 ) ) ;
#53879=DIRECTION ( 'NONE',  ( 0.000000000000000000, -1.000000000000000000, 0.000000000000000000 ) ) ;
#53880=PLANE ( 'NONE',  #36810 ) ;
#53901=DIRECTION ( 'NONE',  ( -0.000000000000000000, 1.000000000000000000, -0.000000000000000000 ) ) ;
#53926=CARTESIAN_POINT ( 'NONE',  ( 0.9285414500055713116, 0.000000000000000000, -0.6299212598425196763 ) ) ;
#53930=CARTESIAN_POINT ( 'NONE',  ( -0.4677827689124922084, 0.03937007874015747977, 2.154527559055118946 ) ) ;
#53962=CARTESIAN_POINT ( 'NONE',  ( 0.2372001242736402615, 1.126255254315259968, 3.929879783441174279 ) ) ;
#53975=EDGE_CURVE ( 'NONE', #23435, #64696, #30408, .T. ) ;
#53978=DIRECTION ( 'NONE',  ( -0.000000000000000000, -1.000000000000000000, -0.000000000000000000 ) ) ;
#53980=CARTESIAN_POINT ( 'NONE',  ( 2.094141031014985721, 1.724409448818900570, -0.4359958488159719758 ) ) ;
#53988=EDGE_CURVE ( 'NONE', #30815, #51378, #52456, .T. ) ;
#53990=CARTESIAN_POINT ( 'NONE',  ( 3.884611959489589594, 2.725289161120230563, -0.5314960629921258173 ) ) ;
#54000=DIRECTION ( 'NONE',  ( 0.000000000000000000, 1.000000000000000000, 0.000000000000000000 ) ) ;
#54022=CARTESIAN_POINT ( 'NONE',  ( -0.03443470937339728616, 1.062992125984252079, -1.537015892239756099 ) ) ;
#54024=LINE ( 'NONE', #8600, #70109 ) ;
#54032=CARTESIAN_POINT ( 'NONE',  ( -1.053714247187549580, 1.260741004084709793, 0.3856939116699171222 ) ) ;
#54054=CARTESIAN_POINT ( 'NONE',  ( 0.000000000000000000, 0.03937007874015751446, -2.874015748031495843 ) ) ;
#54065=CARTESIAN_POINT ( 'NONE',  ( 0.000000000000000000, 0.04488074079120461107, 0.000000000000000000 ) ) ;
#54072=ORIENTED_EDGE ( 'NONE', *, *, #6391, .T. ) ;
#54097=DIRECTION ( 'NONE',  ( 0.000000000000000000, 0.000000000000000000, 1.000000000000000000 ) ) ;
#54099=EDGE_LOOP ( 'NONE', ( #71502, #8191 ) ) ;
#54110=EDGE_CURVE ( 'NONE', #1055, #29055, #22379, .T. ) ;
#54118=B_SPLINE_CURVE_WITH_KNOTS ( 'NONE', 3,
 ( #74592, #22409, #16936, #22816, #48473, #41747 ),
 .UNSPECIFIED., .F., .F.,
 ( 4, 2, 4 ),
 ( 0.001230262104865860332, 0.001674292070114364369, 0.002118322035362868189 ),
 .UNSPECIFIED. ) ;
#54119=ORIENTED_EDGE ( 'NONE', *, *, #35777, .T. ) ;
#54133=CARTESIAN_POINT ( 'NONE',  ( 0.5314960629921393620, 2.751923335154144556, -3.846978723397334488 ) ) ;
#54159=ADVANCED_FACE ( 'NONE', ( #60523 ), #46642, .F. ) ;
#54198=EDGE_LOOP ( 'NONE', ( #33600, #12729, #69821, #78981 ) ) ;
#54216=ORIENTED_EDGE ( 'NONE', *, *, #45360, .T. ) ;
#54219=CARTESIAN_POINT ( 'NONE',  ( 2.704643427489220375, 1.253539720428394677, 0.3811758253793009477 ) ) ;
#54233=DIRECTION ( 'NONE',  ( -1.000000000000000000, -0.000000000000000000, -0.000000000000000000 ) ) ;
#54249=AXIS2_PLACEMENT_3D ( 'NONE', #51718, #25636, #32796 ) ;
#54256=CARTESIAN_POINT ( 'NONE',  ( -3.937007874015748143, 1.537401574803149984, -0.4744094488188975722 ) ) ;
#54261=CARTESIAN_POINT ( 'NONE',  ( -1.947751274789666587, 1.170105060311635192, -0.3006284332565725692 ) ) ;
#54265=EDGE_CURVE ( 'NONE', #29875, #6933, #10045, .T. ) ;
#54289=CIRCLE ( 'NONE', #3243, 0.2165354330708660069 ) ;
#54305=AXIS2_PLACEMENT_3D ( 'NONE', #60212, #53879, #21909 ) ;
#54307=ORIENTED_EDGE ( 'NONE', *, *, #27431, .T. ) ;
#54326=ORIENTED_EDGE ( 'NONE', *, *, #5433, .T. ) ;
#54354=VECTOR ( 'NONE', #71757, 39.37007874015748143 ) ;
#54361=CARTESIAN_POINT ( 'NONE',  ( -0.1687104285705298135, 1.093727987196848161, -1.109387722385912101 ) ) ;
#54392=CARTESIAN_POINT ( 'NONE',  ( -1.614140194556460184, 1.133714490967797417, 0.2492166689920113365 ) ) ;
#54398=B_SPLINE_CURVE_WITH_KNOTS ( 'NONE', 3,
 ( #46056, #14103, #27541, #7783, #34280, #19559, #45218, #2297, #33451, #70919, #59111, #7354, #40588, #1468, #20819, #53198, #78911, #21232, #66270, #8609, #59941, #51528, #13268, #38918, #64599, #6934, #54872, #73838, #22060, #53616, #10689, #29206, #16593, #34700, #28371, #10273, #16178, #74250, #80578, #60363, #54032, #9852, #17012, #42238, #41825, #80985, #55275, #35941, #79744, #61610 ),
 .UNSPECIFIED., .F., .F.,
 ( 4, 2, 2, 2, 2, 2, 2, 2, 2, 2, 2, 2, 2, 2, 2, 2, 2, 2, 2, 2, 2, 2, 2, 2, 4 ),
 ( 0.004882041752397744960, 0.007267356590370914471, 0.008460014009357500961, 0.009652671428344087451, 0.01084532884733067221, 0.01203798626631725870, 0.01442330110429044902, 0.01561595852327704072, 0.01680861594226363415, 0.01919393078023681060, 0.02038658819922340576, 0.02157924561820999398, 0.02277190303719658568, 0.02396456045618317390, 0.02634987529415635729, 0.02754253271314294899, 0.02873519013212954415, 0.03112050497010273101, 0.03350581980807591786, 0.03469847722706250609, 0.03589113464604909431, 0.03827644948402229158, 0.03946910690300887981, 0.04066176432199546803, 0.04304707915996866530 ),
 .UNSPECIFIED. ) ;
#54401=EDGE_LOOP ( 'NONE', ( #35718, #80203, #69834, #5750 ) ) ;
#54406=CARTESIAN_POINT ( 'NONE',  ( 3.937007874015748143, 2.755905511811024056, 0.5314960629921260393 ) ) ;
#54416=CARTESIAN_POINT ( 'NONE',  ( 0.4359958488159310086, 1.724409448818897461, 3.912791665790203766 ) ) ;
#54431=LINE ( 'NONE', #9830, #7256 ) ;
#54435=ORIENTED_EDGE ( 'NONE', *, *, #33602, .T. ) ;
#54440=CARTESIAN_POINT ( 'NONE',  ( -1.313877454013331780, 0.2755905511811023723, 0.7983292792091805090 ) ) ;
#54442=DIRECTION ( 'NONE',  ( 0.000000000000000000, 0.000000000000000000, -1.000000000000000000 ) ) ;
#54477=CIRCLE ( 'NONE', #47746, 0.2165354330708660069 ) ;
#54487=CARTESIAN_POINT ( 'NONE',  ( 0.3813326747118215287, 1.253753238304358808, 2.019942904136674322 ) ) ;
#54515=DIRECTION ( 'NONE',  ( 0.000000000000000000, 1.000000000000000000, 0.000000000000000000 ) ) ;
#54517=EDGE_LOOP ( 'NONE', ( #29749, #15330, #66529, #50444 ) ) ;
#54533=ORIENTED_EDGE ( 'NONE', *, *, #80068, .T. ) ;
#54536=CARTESIAN_POINT ( 'NONE',  ( -1.680497585818729434, 1.332856214479095414, 0.4284113646842339640 ) ) ;
#54537=AXIS2_PLACEMENT_3D ( 'NONE', #54022, #22050, #46044 ) ;
#54542=LINE ( 'NONE', #29706, #71873 ) ;
#54563=DIRECTION ( 'NONE',  ( 0.000000000000000000, 0.000000000000000000, 1.000000000000000000 ) ) ;
#54568=EDGE_CURVE ( 'NONE', #82716, #80251, #47643, .T. ) ;
#54580=CONICAL_SURFACE ( 'NONE', #825, 1.250000000000000000, 0.1221730476396033355 ) ;
#54589=CARTESIAN_POINT ( 'NONE',  ( -3.861376881555339757, 2.746034003362845866, 0.5314960629921258173 ) ) ;
#54600=DIRECTION ( 'NONE',  ( -0.000000000000000000, -1.000000000000000000, -0.000000000000000000 ) ) ;
#54634=ORIENTED_EDGE ( 'NONE', *, *, #16141, .T. ) ;
#54650=VERTEX_POINT ( 'NONE', #74256 ) ;
#54652=CARTESIAN_POINT ( 'NONE',  ( 0.000000000000000000, 0.4177165354330708569, -1.178877988035069047 ) ) ;
#54653=ORIENTED_EDGE ( 'NONE', *, *, #22073, .F. ) ;
#54676=B_SPLINE_CURVE_WITH_KNOTS ( 'NONE', 3,
 ( #30390, #49334, #74622, #43010 ),
 .UNSPECIFIED., .F., .F.,
 ( 4, 4 ),
 ( 2.888536477588258382E-07, 0.001436607511248039464 ),
 .UNSPECIFIED. ) ;
#54679=CARTESIAN_POINT ( 'NONE',  ( 0.5314960629920851831, 2.702643891907236195, 3.896872718254352108 ) ) ;
#54691=AXIS2_PLACEMENT_3D ( 'NONE', #59783, #73684, #59367 ) ;
#54696=AXIS2_PLACEMENT_3D ( 'NONE', #53557, #71686, #28306 ) ;
#54700=AXIS2_PLACEMENT_3D ( 'NONE', #43953, #11993, #37647 ) ;
#54704=DIRECTION ( 'NONE',  ( -0.000000000000000000, -1.000000000000000000, -0.000000000000000000 ) ) ;
#54710=DIRECTION ( 'NONE',  ( 0.000000000000000000, 1.000000000000000000, -1.734723475976808327E-16 ) ) ;
#54714=CARTESIAN_POINT ( 'NONE',  ( 0.2096960158929673246, 1.111548270248051473, 2.829355687306212008 ) ) ;
#54718=EDGE_CURVE ( 'NONE', #70474, #17581, #77529, .T. ) ;
#54721=CARTESIAN_POINT ( 'NONE',  ( 0.5314960629921350321, 2.755905511811024056, -2.583694225513478937 ) ) ;
#54723=ADVANCED_FACE ( 'NONE', ( #29211, #41425 ), #68355, .T. ) ;
#54735=CARTESIAN_POINT ( 'NONE',  ( -0.4744094488188880798, 1.537401574803149984, -2.554262525012305218 ) ) ;
#54746=ORIENTED_EDGE ( 'NONE', *, *, #22, .T. ) ;
#54765=VECTOR ( 'NONE', #29542, 39.37007874015748143 ) ;
#54774=CARTESIAN_POINT ( 'NONE',  ( -0.03443470937339728616, 0.2755905511811023723, -1.537015892239756099 ) ) ;
#54781=CARTESIAN_POINT ( 'NONE',  ( -0.03443470937339728616, 0.2755905511811023723, -1.537015892239756099 ) ) ;
#54797=CARTESIAN_POINT ( 'NONE',  ( -3.937007874015748143, 2.755905511811024056, 0.5314960629921260393 ) ) ;
#54816=CARTESIAN_POINT ( 'NONE',  ( 2.152447471807405588, 1.622068519643040663, -0.4668652553835656027 ) ) ;
#54827=CARTESIAN_POINT ( 'NONE',  ( 3.900447471620230200, 2.687524476698323284, -0.5314960629921260393 ) ) ;
#54853=CARTESIAN_POINT ( 'NONE',  ( -0.4258029703577156933, 1.326239216270301391, -2.646999490626495977 ) ) ;
#54860=CARTESIAN_POINT ( 'NONE',  ( -1.016821367227983774, 1.553543944314659475, 0.4744094488188969616 ) ) ;
#54863=CARTESIAN_POINT ( 'NONE',  ( -0.4422825626179747727, 1.709752412933176258, 3.912091147757427390 ) ) ;
#54864=CARTESIAN_POINT ( 'NONE',  ( -0.03443470937339728616, 1.062992125984252079, -1.635441089090149402 ) ) ;
#54872=CARTESIAN_POINT ( 'NONE',  ( -1.122048159108791632, 1.062989961842522035, -0.01571064279740208569 ) ) ;
#54879=VECTOR ( 'NONE', #47678, 39.37007874015748143 ) ;
#54881=CARTESIAN_POINT ( 'NONE',  ( -3.909100906889131810, 1.617089521489746273, -0.4679440794864275222 ) ) ;
#54888=DIRECTION ( 'NONE',  ( 0.000000000000000000, 1.000000000000000000, -0.000000000000000000 ) ) ;
#54908=LINE ( 'NONE', #28410, #34015 ) ;
#54936=ORIENTED_EDGE ( 'NONE', *, *, #19337, .F. ) ;
#54954=ORIENTED_EDGE ( 'NONE', *, *, #65662, .F. ) ;
#54955=CARTESIAN_POINT ( 'NONE',  ( -2.154527559055114061, 0.03937007874015747977, -0.4677827689125148014 ) ) ;
#54958=DIRECTION ( 'NONE',  ( 0.000000000000000000, 1.000000000000000000, 0.000000000000000000 ) ) ;
#54969=ORIENTED_EDGE ( 'NONE', *, *, #57249, .T. ) ;
#54973=DIRECTION ( 'NONE',  ( -0.000000000000000000, -1.000000000000000000, -0.000000000000000000 ) ) ;
#54995=CARTESIAN_POINT ( 'NONE',  ( -2.543486866223389153, 2.716535433070866645, 0.5314960629921260393 ) ) ;
#55002=ORIENTED_EDGE ( 'NONE', *, *, #11630, .F. ) ;
#55020=ADVANCED_FACE ( 'NONE', ( #36309 ), #26119, .T. ) ;
#55027=ORIENTED_EDGE ( 'NONE', *, *, #15607, .F. ) ;
#55030=EDGE_CURVE ( 'NONE', #44550, #29599, #47271, .T. ) ;
#55044=ORIENTED_EDGE ( 'NONE', *, *, #7150, .T. ) ;
#55047=CARTESIAN_POINT ( 'NONE',  ( -0.3149606299212734384, 2.755905511811024056, 3.924389226575467404 ) ) ;
#55060=VERTEX_POINT ( 'NONE', #35908 ) ;
#55085=CARTESIAN_POINT ( 'NONE',  ( 0.5314960629920851831, 2.677165354330708791, 3.900966923095595451 ) ) ;
#55113=VERTEX_POINT ( 'NONE', #41790 ) ;
#55128=ORIENTED_EDGE ( 'NONE', *, *, #51138, .T. ) ;
#55134=FACE_OUTER_BOUND ( 'NONE', #51626, .T. ) ;
#55139=DIRECTION ( 'NONE',  ( -1.000000000000000000, -9.738798461624180871E-16, 0.000000000000000000 ) ) ;
#55175=DIRECTION ( 'NONE',  ( 3.491481338843132961E-15, 0.000000000000000000, -1.000000000000000000 ) ) ;
#55182=CARTESIAN_POINT ( 'NONE',  ( -0.4107360162338847265, 1.299495150281466227, -1.044197310779563237 ) ) ;
#55183=EDGE_CURVE ( 'NONE', #1571, #34573, #11341, .T. ) ;
#55189=ADVANCED_FACE ( 'NONE', ( #31222 ), #63630, .F. ) ;
#55219=DIRECTION ( 'NONE',  ( 0.000000000000000000, 1.000000000000000000, -0.000000000000000000 ) ) ;
#55229=DIRECTION ( 'NONE',  ( -0.000000000000000000, -1.000000000000000000, -0.000000000000000000 ) ) ;
#55231=CIRCLE ( 'NONE', #45791, 1.968503937007874072 ) ;
#55232=CARTESIAN_POINT ( 'NONE',  ( -0.06312602682716046687, 1.066946945958372028, 1.120379939242540868 ) ) ;
#55255=CARTESIAN_POINT ( 'NONE',  ( -0.2516608251556126663, 1.134091190147785699, -2.808839726227330580 ) ) ;
#55259=ORIENTED_EDGE ( 'NONE', *, *, #65662, .T. ) ;
#55275=CARTESIAN_POINT ( 'NONE',  ( -1.022479694362532499, 1.428910228063043686, 0.4621002115169275393 ) ) ;
#55283=CARTESIAN_POINT ( 'NONE',  ( -1.076935383196057527, 2.165354330708661568, -0.3149606299212600047 ) ) ;
#55290=ADVANCED_FACE ( 'NONE', ( #69942 ), #44659, .T. ) ;
#55291=CARTESIAN_POINT ( 'NONE',  ( 2.611754389584936220, 1.697151583350149595, -0.4469586986359051495 ) ) ;
#55299=CARTESIAN_POINT ( 'NONE',  ( 0.4497697399585466882, 1.386499259343020762, -1.566055164954403889 ) ) ;
#55306=CARTESIAN_POINT ( 'NONE',  ( -1.313877454013331780, 1.062992125984252079, 0.8967544760595740350 ) ) ;
#55313=CARTESIAN_POINT ( 'NONE',  ( 0.4732412630952341770, 1.503056026428866598, 2.167282348326871055 ) ) ;
#55316=EDGE_CURVE ( 'NONE', #23166, #32357, #15398, .T. ) ;
#55318=EDGE_LOOP ( 'NONE', ( #45737, #17583, #54746, #40277, #47258, #46872, #23995, #6084 ) ) ;
#55322=CARTESIAN_POINT ( 'NONE',  ( -2.094141031014932874, 1.724409448818898127, -0.4359958488159723644 ) ) ;
#55345=EDGE_CURVE ( 'NONE', #78599, #38787, #4728, .T. ) ;
#55363=VERTEX_POINT ( 'NONE', #24086 ) ;
#55364=CARTESIAN_POINT ( 'NONE',  ( -1.559171609364246924, 0.4110443821404751730, 0.5949441279213820710 ) ) ;
#55380=DIRECTION ( 'NONE',  ( 0.000000000000000000, -0.000000000000000000, -1.000000000000000000 ) ) ;
#55396=VECTOR ( 'NONE', #3895, 39.37007874015748143 ) ;
#55412=ORIENTED_EDGE ( 'NONE', *, *, #35732, .F. ) ;
#55438=ORIENTED_EDGE ( 'NONE', *, *, #6944, .T. ) ;
#55439=CONICAL_SURFACE ( 'NONE', #70222, 2.637795275590551380, 0.7853981633974500554 ) ;
#55461=CARTESIAN_POINT ( 'NONE',  ( 0.4744094488188941861, 1.553443221530653728, 1.016821367227985329 ) ) ;
#55466=ORIENTED_EDGE ( 'NONE', *, *, #68728, .F. ) ;
#55468=CARTESIAN_POINT ( 'NONE',  ( -0.03443470937339727228, 1.062992125984252079, -1.438590695389362573 ) ) ;
#55471=DIRECTION ( 'NONE',  ( 1.000000000000000000, 1.408710688920637755E-15, 0.000000000000000000 ) ) ;
#55488=AXIS2_PLACEMENT_3D ( 'NONE', #54065, #53235, #59560 ) ;
#55497=CARTESIAN_POINT ( 'NONE',  ( -2.167277156196906418, 1.503024749832831741, 0.4732391302016646928 ) ) ;
#55502=AXIS2_PLACEMENT_3D ( 'NONE', #65281, #25281, #19396 ) ;
#55515=CYLINDRICAL_SURFACE ( 'NONE', #17239, 0.1771653543307085410 ) ;
#55542=CIRCLE ( 'NONE', #38121, 3.405511811023621771 ) ;
#55549=DIRECTION ( 'NONE',  ( -0.000000000000000000, -1.000000000000000000, -0.000000000000000000 ) ) ;
#55552=VERTEX_POINT ( 'NONE', #17794 ) ;
#55555=EDGE_LOOP ( 'NONE', ( #31943, #18613, #52446, #36955 ) ) ;
#55583=FACE_OUTER_BOUND ( 'NONE', #2696, .T. ) ;
#55587=CARTESIAN_POINT ( 'NONE',  ( -3.264097702071373064, 2.755905511811024056, 0.5314960629921260393 ) ) ;
#55590=CARTESIAN_POINT ( 'NONE',  ( -2.867114984585481974, 1.070443199938759138, 0.08545185031214221072 ) ) ;
#55596=EDGE_CURVE ( 'NONE', #79730, #32076, #26381, .T. ) ;
#55605=VECTOR ( 'NONE', #34547, 39.37007874015748143 ) ;
#55608=CARTESIAN_POINT ( 'NONE',  ( 0.4606671848300903926, 1.422950954677614011, -2.139052088108191807 ) ) ;
#55616=CIRCLE ( 'NONE', #48899, 3.937007874015748143 ) ;
#55626=CARTESIAN_POINT ( 'NONE',  ( -1.607431655553806182, 1.132464663736809873, 0.2471720702981345663 ) ) ;
#55634=EDGE_LOOP ( 'NONE', ( #51098, #79495, #62818, #66027 ) ) ;
#55662=VECTOR ( 'NONE', #76417, 39.37007874015748143 ) ;
#55665=CARTESIAN_POINT ( 'NONE',  ( -0.3006999498584465025, 1.170162153792019710, -2.776607427673829509 ) ) ;
#55678=CARTESIAN_POINT ( 'NONE',  ( 0.4623158380715545746, 0.02617651024168223331, -2.142213561789874543 ) ) ;
#55702=DIRECTION ( 'NONE',  ( 0.000000000000000000, 0.000000000000000000, 1.000000000000000000 ) ) ;
#55723=CARTESIAN_POINT ( 'NONE',  ( 0.4124503923812352646, 1.301275207309030346, 2.058161246854230519 ) ) ;
#55727=EDGE_CURVE ( 'NONE', #51415, #52887, #74585, .T. ) ;
#55742=LINE ( 'NONE', #75543, #31265 ) ;
#55749=ADVANCED_FACE ( 'NONE', ( #68025 ), #42326, .F. ) ;
#55773=ORIENTED_EDGE ( 'NONE', *, *, #23955, .F. ) ;
#55774=FACE_OUTER_BOUND ( 'NONE', #9604, .T. ) ;
#55777=LINE ( 'NONE', #42738, #41135 ) ;
#55779=CARTESIAN_POINT ( 'NONE',  ( 0.5314960629921396951, 2.559055118110236560, -3.937007874015760578 ) ) ;
#55792=CARTESIAN_POINT ( 'NONE',  ( 1.455672919077434579E-16, 0.4374015748031496176, 1.178877988035069047 ) ) ;
#55801=CIRCLE ( 'NONE', #12798, 3.307086614173228689 ) ;
#55811=EDGE_CURVE ( 'NONE', #78599, #43641, #54542, .T. ) ;
#55823=ORIENTED_EDGE ( 'NONE', *, *, #35062, .F. ) ;
#55831=CARTESIAN_POINT ( 'NONE',  ( 1.141392835773559211, 0.3937007874015748254, 1.141392835773562764 ) ) ;
#55849=ORIENTED_EDGE ( 'NONE', *, *, #48124, .F. ) ;
#55851=VERTEX_POINT ( 'NONE', #73090 ) ;
#55863=ORIENTED_EDGE ( 'NONE', *, *, #70014, .F. ) ;
#55865=VERTEX_POINT ( 'NONE', #80667 ) ;
#55868=DIRECTION ( 'NONE',  ( 0.000000000000000000, 0.000000000000000000, 1.000000000000000000 ) ) ;
#55871=CARTESIAN_POINT ( 'NONE',  ( -2.362204724409448620, 1.929133858267716661, -2.474278114140802984E-14 ) ) ;
#55880=CARTESIAN_POINT ( 'NONE',  ( 3.909792448225465566, 1.429026188080324333, 0.4621293626231841034 ) ) ;
#55882=VERTEX_POINT ( 'NONE', #47399 ) ;
#55887=CARTESIAN_POINT ( 'NONE',  ( 0.000000000000000000, 2.755905511811024056, 0.000000000000000000 ) ) ;
#55898=CIRCLE ( 'NONE', #18305, 1.122047244094488194 ) ;
#55941=CARTESIAN_POINT ( 'NONE',  ( 0.000000000000000000, 2.165354330708661568, 0.000000000000000000 ) ) ;
#55944=CARTESIAN_POINT ( 'NONE',  ( -3.937007874015748143, 2.165354330708661568, -0.3149606299212600047 ) ) ;
#55951=VERTEX_POINT ( 'NONE', #16687 ) ;
#55954=ORIENTED_EDGE ( 'NONE', *, *, #73105, .T. ) ;
#55965=FACE_OUTER_BOUND ( 'NONE', #6520, .T. ) ;
#55968=ORIENTED_EDGE ( 'NONE', *, *, #14716, .F. ) ;
#55971=ORIENTED_EDGE ( 'NONE', *, *, #62649, .T. ) ;
#55973=AXIS2_PLACEMENT_3D ( 'NONE', #1776, #66168, #8508 ) ;
#56003=PLANE ( 'NONE',  #42622 ) ;
#56006=CARTESIAN_POINT ( 'NONE',  ( -2.822823420596379140, 1.118719813955001863, -0.2236424093447015315 ) ) ;
#56009=DIRECTION ( 'NONE',  ( -1.000000000000000000, -0.000000000000000000, -0.000000000000000000 ) ) ;
#56014=CIRCLE ( 'NONE', #17125, 0.5118110236220472231 ) ;
#56022=CARTESIAN_POINT ( 'NONE',  ( 0.4257251611738756547, 1.325776663396805555, -1.038227845120437642 ) ) ;
#56044=DIRECTION ( 'NONE',  ( 0.000000000000000000, 0.000000000000000000, -1.000000000000000000 ) ) ;
#56045=DIRECTION ( 'NONE',  ( 0.000000000000000000, 0.000000000000000000, -1.000000000000000000 ) ) ;
#56051=ORIENTED_EDGE ( 'NONE', *, *, #51081, .T. ) ;
#56060=AXIS2_PLACEMENT_3D ( 'NONE', #18598, #23663, #75035 ) ;
#56070=ORIENTED_EDGE ( 'NONE', *, *, #4271, .T. ) ;
#56077=ADVANCED_FACE ( 'NONE', ( #40679, #66364 ), #8702, .T. ) ;
#56087=CARTESIAN_POINT ( 'NONE',  ( 1.150409065943327258, 0.2755905511811023723, 0.8265612839971842041 ) ) ;
#56090=ORIENTED_EDGE ( 'NONE', *, *, #18680, .F. ) ;
#56091=VERTEX_POINT ( 'NONE', #67199 ) ;
#56094=DIRECTION ( 'NONE',  ( 0.000000000000000000, 0.000000000000000000, -1.000000000000000000 ) ) ;
#56095=CARTESIAN_POINT ( 'NONE',  ( 3.937007874015748143, 1.724409448818898127, 0.6299212598425202314 ) ) ;
#56113=DIRECTION ( 'NONE',  ( -0.000000000000000000, -1.000000000000000000, -0.000000000000000000 ) ) ;
#56120=CARTESIAN_POINT ( 'NONE',  ( -3.937007874015748143, 1.537401574803149984, -2.901595197523589142E-16 ) ) ;
#56128=CARTESIAN_POINT ( 'NONE',  ( 1.122050806839039794, 1.062983699574960195, -0.01543924256646982823 ) ) ;
#56135=LINE ( 'NONE', #10303, #15165 ) ;
#56142=CARTESIAN_POINT ( 'NONE',  ( 0.2512006810191718675, 1.134651008203187761, 1.916017364051557426 ) ) ;
#56148=ORIENTED_EDGE ( 'NONE', *, *, #77992, .F. ) ;
#56152=CARTESIAN_POINT ( 'NONE',  ( 0.000000000000000000, 2.755905511811024056, 0.000000000000000000 ) ) ;
#56161=CARTESIAN_POINT ( 'NONE',  ( -0.5314960629921197111, 2.755905511811024056, -1.813482582612295557 ) ) ;
#56207=ORIENTED_EDGE ( 'NONE', *, *, #41448, .F. ) ;
#56208=EDGE_CURVE ( 'NONE', #23435, #32357, #69259, .T. ) ;
#56217=CARTESIAN_POINT ( 'NONE',  ( 3.900966923095589678, 2.559055118110236560, 0.5314960629921260393 ) ) ;
#56234=ADVANCED_FACE ( 'NONE', ( #49058 ), #81487, .F. ) ;
#56246=ORIENTED_EDGE ( 'NONE', *, *, #83089, .T. ) ;
#56258=CARTESIAN_POINT ( 'NONE',  ( 0.2733222648309123204, 1.149615049381084608, -1.456396182690151031 ) ) ;
#56273=ORIENTED_EDGE ( 'NONE', *, *, #82019, .F. ) ;
#56282=ADVANCED_FACE ( 'NONE', ( #4452 ), #76399, .F. ) ;
#56288=ORIENTED_EDGE ( 'NONE', *, *, #41957, .T. ) ;
#56296=CARTESIAN_POINT ( 'NONE',  ( -0.4614843117558885544, 1.648562443335530370, -3.909868781823469419 ) ) ;
#56298=CARTESIAN_POINT ( 'NONE',  ( -1.736178228450298011, 1.299212598425196985, 0.4102808022082834460 ) ) ;
#56304=ORIENTED_EDGE ( 'NONE', *, *, #69071, .F. ) ;
#56309=DIRECTION ( 'NONE',  ( 0.000000000000000000, -1.000000000000000000, 1.408710688920637755E-15 ) ) ;
#56331=CARTESIAN_POINT ( 'NONE',  ( 0.5314960629920989499, 2.755905511811024056, 2.583694225513486042 ) ) ;
#56351=AXIS2_PLACEMENT_3D ( 'NONE', #59834, #66580, #21539 ) ;
#56352=EDGE_CURVE ( 'NONE', #9951, #10674, #52154, .T. ) ;
#56357=EDGE_CURVE ( 'NONE', #55363, #13254, #16847, .T. ) ;
#56386=VERTEX_POINT ( 'NONE', #74757 ) ;
#56394=EDGE_CURVE ( 'NONE', #51414, #64697, #61156, .T. ) ;
#56421=CARTESIAN_POINT ( 'NONE',  ( -0.03443470937339728616, 1.062992125984252079, -1.537015892239756099 ) ) ;
#56424=CARTESIAN_POINT ( 'NONE',  ( -0.07518215644454619151, 1.068889330503016932, -1.616455086487287529 ) ) ;
#56433=CARTESIAN_POINT ( 'NONE',  ( 0.2770644220722718876, 1.151992524107844806, -1.087382630950603613 ) ) ;
#56436=DIRECTION ( 'NONE',  ( 0.000000000000000000, 0.000000000000000000, -1.000000000000000000 ) ) ;
#56441=DIRECTION ( 'NONE',  ( 0.000000000000000000, 0.000000000000000000, 1.000000000000000000 ) ) ;
#56456=CARTESIAN_POINT ( 'NONE',  ( 0.000000000000000000, 0.4177165354330708569, 0.000000000000000000 ) ) ;
#56467=STYLED_ITEM ( 'NONE', ( #49374 ), #33697 ) ;
#56470=CARTESIAN_POINT ( 'NONE',  ( 0.000000000000000000, 0.000000000000000000, -3.444881889763779625 ) ) ;
#56479=CARTESIAN_POINT ( 'NONE',  ( -0.1807970329289189937, 1.098498331261037686, -1.883127487649877141 ) ) ;
#56480=EDGE_LOOP ( 'NONE', ( #45527, #62004, #13446, #27818 ) ) ;
#56496=CARTESIAN_POINT ( 'NONE',  ( 0.000000000000000000, 2.755905511811024056, 0.000000000000000000 ) ) ;
#56499=ORIENTED_EDGE ( 'NONE', *, *, #34592, .T. ) ;
#56503=CYLINDRICAL_SURFACE ( 'NONE', #9516, 0.1771653543307085410 ) ;
#56504=CARTESIAN_POINT ( 'NONE',  ( 5.818687728935708833E-24, 1.062992125984252745, -3.937007874015748143 ) ) ;
#56523=CARTESIAN_POINT ( 'NONE',  ( -0.4476898780827052726, 1.379730629998461522, 2.113977306180467863 ) ) ;
#56534=AXIS2_PLACEMENT_3D ( 'NONE', #53809, #35301, #61795 ) ;
#56539=CARTESIAN_POINT ( 'NONE',  ( 1.116858202696501046, 1.075390326517888351, -0.1088746120232600839 ) ) ;
#56542=CARTESIAN_POINT ( 'NONE',  ( 0.4744094488188839720, 1.537401574803149984, 3.908320185825793658 ) ) ;
#56556=ORIENTED_EDGE ( 'NONE', *, *, #7406, .F. ) ;
#56568=CARTESIAN_POINT ( 'NONE',  ( -0.3767879474345934843, 1.247505695433910100, 1.057050330549203832 ) ) ;
#56569=CARTESIAN_POINT ( 'NONE',  ( 1.141392835773559211, 0.3937007874015748254, 1.141392835773562764 ) ) ;
#56586=FACE_OUTER_BOUND ( 'NONE', #76572, .T. ) ;
#56591=AXIS2_PLACEMENT_3D ( 'NONE', #77386, #70645, #44949 ) ;
#56597=EDGE_LOOP ( 'NONE', ( #36598, #60939, #21651, #64195, #21684, #78230, #65847, #37152, #19659, #60968, #2469, #81593, #12610, #13360 ) ) ;
#56599=ORIENTED_EDGE ( 'NONE', *, *, #52769, .T. ) ;
#56604=CARTESIAN_POINT ( 'NONE',  ( -0.4744094488188832504, 1.537401574803149984, -3.937007874015763687 ) ) ;
#56615=CARTESIAN_POINT ( 'NONE',  ( 2.118110236220470899, 0.000000000000000000, 0.4498537592782972383 ) ) ;
#56618=CARTESIAN_POINT ( 'NONE',  ( 2.170146923806595574, 1.546132656481028933, 0.4744094488188977388 ) ) ;
#56649=ORIENTED_EDGE ( 'NONE', *, *, #55727, .T. ) ;
#56661=CARTESIAN_POINT ( 'NONE',  ( 0.2885979965725480323, 1.160566086728936908, 2.785141739107498182 ) ) ;
#56673=CARTESIAN_POINT ( 'NONE',  ( 0.000000000000000000, 1.929133858267716661, -2.362204724409448620 ) ) ;
#56675=ORIENTED_EDGE ( 'NONE', *, *, #63509, .T. ) ;
#56687=EDGE_CURVE ( 'NONE', #35211, #41007, #53100, .T. ) ;
#56700=DIRECTION ( 'NONE',  ( 0.000000000000000000, 0.000000000000000000, -1.000000000000000000 ) ) ;
#56711=EDGE_LOOP ( 'NONE', ( #25615, #50242, #78786, #1330 ) ) ;
#56713=CIRCLE ( 'NONE', #2967, 3.937007874015748143 ) ;
#56719=CARTESIAN_POINT ( 'NONE',  ( -0.3576100502496167843, 1.224098650525152543, 3.920795739734008301 ) ) ;
#56737=CARTESIAN_POINT ( 'NONE',  ( -2.170146923806674621, 1.528780496884627915, 0.4744094488188969616 ) ) ;
#56755=CARTESIAN_POINT ( 'NONE',  ( -3.936002401691375052, 1.071382210147229452, -0.09277206283147471089 ) ) ;
#56760=ORIENTED_EDGE ( 'NONE', *, *, #31624, .F. ) ;
#56761=CARTESIAN_POINT ( 'NONE',  ( 0.000000000000000000, 0.000000000000000000, 1.122047244094488194 ) ) ;
#56763=CIRCLE ( 'NONE', #20509, 2.559055118110236560 ) ;
#56776=ORIENTED_EDGE ( 'NONE', *, *, #51390, .F. ) ;
#56790=ORIENTED_EDGE ( 'NONE', *, *, #36043, .T. ) ;
#56792=ORIENTED_EDGE ( 'NONE', *, *, #7741, .T. ) ;
#56794=CARTESIAN_POINT ( 'NONE',  ( 1.141392835773559211, 0.000000000000000000, 1.141392835773562764 ) ) ;
#56817=EDGE_CURVE ( 'NONE', #69342, #14187, #11425, .T. ) ;
#56827=CARTESIAN_POINT ( 'NONE',  ( -2.869680830158521712, 1.067671560069319403, 0.06860298820098456596 ) ) ;
#56839=FACE_OUTER_BOUND ( 'NONE', #72175, .T. ) ;
#56841=ADVANCED_FACE ( 'NONE', ( #37665 ), #35639, .T. ) ;
#56848=CARTESIAN_POINT ( 'NONE',  ( -1.559171609364246924, 0.3937007874015747699, 0.4177787735906735578 ) ) ;
#56851=EDGE_CURVE ( 'NONE', #71433, #27584, #27573, .T. ) ;
#56863=CARTESIAN_POINT ( 'NONE',  ( -0.03443470937339728616, 0.2755905511811023723, -1.537015892239756099 ) ) ;
#56881=DIRECTION ( 'NONE',  ( -3.491481338843133355E-15, -0.000000000000000000, 1.000000000000000000 ) ) ;
#56906=CARTESIAN_POINT ( 'NONE',  ( -2.094141031014932874, 1.724409448818898127, -0.4359958488159723644 ) ) ;
#56914=DIRECTION ( 'NONE',  ( -0.8660254037844433705, 0.000000000000000000, 0.4999999999999920064 ) ) ;
#56922=VECTOR ( 'NONE', #30256, 39.37007874015748143 ) ;
#56933=FACE_OUTER_BOUND ( 'NONE', #56597, .T. ) ;
#56976=CARTESIAN_POINT ( 'NONE',  ( -0.5314960629921169355, 2.755905511811024056, -2.583694225513482490 ) ) ;
#56977=VECTOR ( 'NONE', #71000, 39.37007874015748143 ) ;
#56994=CARTESIAN_POINT ( 'NONE',  ( -0.5314960629921346991, 2.755905511811024056, 2.503252890251014939 ) ) ;
#57004=ORIENTED_EDGE ( 'NONE', *, *, #6973, .T. ) ;
#57006=VERTEX_POINT ( 'NONE', #58258 ) ;
#57012=CARTESIAN_POINT ( 'NONE',  ( -3.937007874015748143, 2.559055118110236560, -0.3149606299212599492 ) ) ;
#57026=CARTESIAN_POINT ( 'NONE',  ( 2.169549097624094092, 1.554815631980116741, 0.4741686481756398064 ) ) ;
#57032=FACE_OUTER_BOUND ( 'NONE', #32040, .T. ) ;
#57038=AXIS2_PLACEMENT_3D ( 'NONE', #68454, #5296, #11208 ) ;
#57050=AXIS2_PLACEMENT_3D ( 'NONE', #15093, #2042, #15930 ) ;
#57071=CARTESIAN_POINT ( 'NONE',  ( 0.01711686753222834215, 1.062992125984252967, 2.874015748031495843 ) ) ;
#57075=CARTESIAN_POINT ( 'NONE',  ( -1.519422763189357539, 0.1377952755905511861, 0.7302211324797360792 ) ) ;
#57084=EDGE_LOOP ( 'NONE', ( #42413, #16867, #51000, #66025 ) ) ;
#57094=EDGE_CURVE ( 'NONE', #19150, #55865, #21025, .T. ) ;
#57106=CARTESIAN_POINT ( 'NONE',  ( 2.530077726415320249, 2.729661064330337616, -0.5314960629921260393 ) ) ;
#57108=CIRCLE ( 'NONE', #23486, 0.2165354330708659791 ) ;
#57110=CARTESIAN_POINT ( 'NONE',  ( 3.250800423740332512, 2.742781085175769018, 0.5314960629921260393 ) ) ;
#57144=CARTESIAN_POINT ( 'NONE',  ( -2.153151837758440212, 1.453715418023200145, 0.4672341690643352363 ) ) ;
#57160=CONICAL_SURFACE ( 'NONE', #67957, 3.228346456692913424, 0.7853981633974500554 ) ;
#57163=DIRECTION ( 'NONE',  ( -0.000000000000000000, 1.000000000000000000, -0.000000000000000000 ) ) ;
#57175=DIRECTION ( 'NONE',  ( 0.000000000000000000, 0.000000000000000000, -1.000000000000000000 ) ) ;
#57178=DIRECTION ( 'NONE',  ( 0.000000000000000000, 1.000000000000000000, 0.000000000000000000 ) ) ;
#57184=ORIENTED_EDGE ( 'NONE', *, *, #24269, .T. ) ;
#57201=CIRCLE ( 'NONE', #37092, 2.598425196850393970 ) ;
#57238=EDGE_CURVE ( 'NONE', #66126, #74865, #38909, .T. ) ;
#57246=CARTESIAN_POINT ( 'NONE',  ( 0.3245613508421869020, 1.191052126719460036, -1.074140734518187701 ) ) ;
#57249=EDGE_CURVE ( 'NONE', #49969, #66560, #62153, .T. ) ;
#57250=CARTESIAN_POINT ( 'NONE',  ( 0.1181161979004412693, 1.077624259009876573, -1.863928217990339364 ) ) ;
#57252=CONICAL_SURFACE ( 'NONE', #21004, 0.1978346456692914035, 0.8726646259971700959 ) ;
#57258=EDGE_CURVE ( 'NONE', #45100, #38768, #80568, .T. ) ;
#57272=CARTESIAN_POINT ( 'NONE',  ( 0.6299212598425235621, 2.165354330708662012, -0.9285414500055688691 ) ) ;
#57273=DIRECTION ( 'NONE',  ( 0.000000000000000000, -1.000000000000000000, 0.000000000000000000 ) ) ;
#57278=CIRCLE ( 'NONE', #41218, 0.1771653543307085410 ) ;
#57298=ORIENTED_EDGE ( 'NONE', *, *, #68594, .T. ) ;
#57311=CARTESIAN_POINT ( 'NONE',  ( -2.362204724409448620, 1.724409448818897461, -2.474278114140802984E-14 ) ) ;
#57313=DIRECTION ( 'NONE',  ( 0.000000000000000000, 1.000000000000000000, 0.000000000000000000 ) ) ;
#57314=EDGE_CURVE ( 'NONE', #24482, #25219, #60232, .T. ) ;
#57317=EDGE_LOOP ( 'NONE', ( #2048, #26810, #43215, #34866, #29075, #21377 ) ) ;
#57319=AXIS2_PLACEMENT_3D ( 'NONE', #13174, #32935, #51856 ) ;
#57344=CARTESIAN_POINT ( 'NONE',  ( -0.2239781325220785713, 1.118900601684390761, 1.901750336123934737 ) ) ;
#57349=DIRECTION ( 'NONE',  ( -0.000000000000000000, -1.000000000000000000, -0.000000000000000000 ) ) ;
#57358=CARTESIAN_POINT ( 'NONE',  ( 1.038214557251247117, 1.325842827038092420, 0.4257573143050834008 ) ) ;
#57361=PLANE ( 'NONE',  #41427 ) ;
#57380=VECTOR ( 'NONE', #2523, 39.37007874015748143 ) ;
#57389=EDGE_CURVE ( 'NONE', #9709, #45259, #38316, .T. ) ;
#57393=CARTESIAN_POINT ( 'NONE',  ( -1.854472803289052507, 2.716535433070866645, -0.5314960629921260393 ) ) ;
#57395=EDGE_CURVE ( 'NONE', #69205, #37133, #57108, .T. ) ;
#57420=EDGE_LOOP ( 'NONE', ( #45703, #70679, #74868, #1535 ) ) ;
#57422=VERTEX_POINT ( 'NONE', #15759 ) ;
#57440=CARTESIAN_POINT ( 'NONE',  ( 0.4102808022082901629, 1.299212598425196985, -1.736178228450289573 ) ) ;
#57446=CARTESIAN_POINT ( 'NONE',  ( -1.868118647894634776, 2.729653158204613739, -0.5314960629921260393 ) ) ;
#57447=DIRECTION ( 'NONE',  ( 0.000000000000000000, 0.000000000000000000, -1.000000000000000000 ) ) ;
#57483=ADVANCED_FACE ( 'NONE', ( #48542, #22051 ), #66260, .T. ) ;
#57486=CARTESIAN_POINT ( 'NONE',  ( 0.3961676841499099377, 1.274902735363087736, -1.382762819646744523 ) ) ;
#57498=AXIS2_PLACEMENT_3D ( 'NONE', #53455, #8032, #72829 ) ;
#57500=VERTEX_POINT ( 'NONE', #80154 ) ;
#57528=CARTESIAN_POINT ( 'NONE',  ( 3.237502114873379799, 2.729657712569140582, 0.5314960629921260393 ) ) ;
#57534=DIRECTION ( 'NONE',  ( 0.000000000000000000, -1.000000000000000000, -0.000000000000000000 ) ) ;
#57542=CARTESIAN_POINT ( 'NONE',  ( 1.923693779251858693, 1.143166703770561732, 0.2643333500026358585 ) ) ;
#57575=EDGE_CURVE ( 'NONE', #37133, #17817, #67906, .T. ) ;
#57581=DIRECTION ( 'NONE',  ( -1.953992523340275511E-14, -1.460819769243627131E-15, -1.000000000000000000 ) ) ;
#57602=EDGE_LOOP ( 'NONE', ( #5266, #56288, #21918, #7104 ) ) ;
#57615=CARTESIAN_POINT ( 'NONE',  ( 0.3811282389481255306, 1.253478596003493095, -2.704694874393154702 ) ) ;
#57623=CARTESIAN_POINT ( 'NONE',  ( 2.873110008490984857, 1.063968899401425583, -0.03484477857462457695 ) ) ;
#57655=CARTESIAN_POINT ( 'NONE',  ( 3.184294706754630777, 2.755905511811024056, 0.5314960629921260393 ) ) ;
#57678=CARTESIAN_POINT ( 'NONE',  ( -0.4705807874741004815, 1.475249678874074322, -3.908783329518705330 ) ) ;
#57683=DIRECTION ( 'NONE',  ( 1.000000000000000000, -0.000000000000000000, -0.000000000000000000 ) ) ;
#57691=DIRECTION ( 'NONE',  ( 0.000000000000000000, 1.000000000000000000, 0.000000000000000000 ) ) ;
#57715=DIRECTION ( 'NONE',  ( 1.000000000000000000, -0.000000000000000000, -0.000000000000000000 ) ) ;
#57732=CARTESIAN_POINT ( 'NONE',  ( -1.313877454013331780, 0.2755905511811023723, 0.7983292792091805090 ) ) ;
#57735=ORIENTED_EDGE ( 'NONE', *, *, #50179, .T. ) ;
#57736=EDGE_CURVE ( 'NONE', #36842, #58460, #9427, .T. ) ;
#57737=ORIENTED_EDGE ( 'NONE', *, *, #57803, .F. ) ;
#57762=CARTESIAN_POINT ( 'NONE',  ( -0.4744094488189047332, 1.528796061338912882, 2.170146923806633765 ) ) ;
#57767=CARTESIAN_POINT ( 'NONE',  ( -0.4417590601942997797, 1.710972922415816555, 2.103514684735031892 ) ) ;
#57774=CARTESIAN_POINT ( 'NONE',  ( 1.063938142021821021, 1.224083459767688176, 0.3565564186812866243 ) ) ;
#57801=DIRECTION ( 'NONE',  ( 0.000000000000000000, 0.000000000000000000, -1.000000000000000000 ) ) ;
#57803=EDGE_CURVE ( 'NONE', #35701, #21301, #43650, .T. ) ;
#57832=DIRECTION ( 'NONE',  ( -0.000000000000000000, -1.000000000000000000, -0.000000000000000000 ) ) ;
#57837=CARTESIAN_POINT ( 'NONE',  ( -0.3813326747118357951, 1.253753238304356810, 2.704466544682207374 ) ) ;
#57838=CARTESIAN_POINT ( 'NONE',  ( -2.154527559055114061, 0.03937007874015747977, -0.4677827689125148014 ) ) ;
#57850=DIRECTION ( 'NONE',  ( 0.000000000000000000, -1.000000000000000000, 0.000000000000000000 ) ) ;
#57857=CARTESIAN_POINT ( 'NONE',  ( 0.4677827689124922084, 0.03937007874015747977, -2.154527559055118946 ) ) ;
#57880=DIRECTION ( 'NONE',  ( 0.000000000000000000, -1.000000000000000000, -0.000000000000000000 ) ) ;
#57884=VERTEX_POINT ( 'NONE', #62418 ) ;
#57885=EDGE_CURVE ( 'NONE', #24806, #72153, #65197, .T. ) ;
#57900=CARTESIAN_POINT ( 'NONE',  ( 0.4670403427555926967, 1.622209144264177283, 2.571698080334799297 ) ) ;
#57914=EDGE_LOOP ( 'NONE', ( #18418, #73624, #46751 ) ) ;
#57915=ORIENTED_EDGE ( 'NONE', *, *, #66595, .F. ) ;
#57939=CARTESIAN_POINT ( 'NONE',  ( -0.005429349025308751603, 1.062992125984252745, -1.442783214386379020 ) ) ;
#57946=ORIENTED_EDGE ( 'NONE', *, *, #19828, .F. ) ;
#57953=CARTESIAN_POINT ( 'NONE',  ( -2.170146923806675954, 1.554943921348594049, 0.4744094488188970171 ) ) ;
#57961=EDGE_CURVE ( 'NONE', #9709, #77311, #70562, .T. ) ;
#57967=CARTESIAN_POINT ( 'NONE',  ( -0.08704787641669393949, 1.071034085402255309, -1.469981051961803287 ) ) ;
#57970=AXIS2_PLACEMENT_3D ( 'NONE', #59516, #14095, #39747 ) ;
#57979=DIRECTION ( 'NONE',  ( 0.000000000000000000, 0.000000000000000000, -1.000000000000000000 ) ) ;
#57981=CARTESIAN_POINT ( 'NONE',  ( -1.033875059083676717, 1.724409448818897905, -0.4359958488159722534 ) ) ;
#58003=ORIENTED_EDGE ( 'NONE', *, *, #5997, .F. ) ;
#58004=DIRECTION ( 'NONE',  ( -8.881784197001252323E-16, 0.000000000000000000, 1.000000000000000000 ) ) ;
#58016=ORIENTED_EDGE ( 'NONE', *, *, #25337, .F. ) ;
#58028=AXIS2_PLACEMENT_3D ( 'NONE', #56456, #70756, #51367 ) ;
#58038=CARTESIAN_POINT ( 'NONE',  ( 2.610350574616482788, 1.379859446982311777, -0.4477348144951681652 ) ) ;
#58066=DIRECTION ( 'NONE',  ( 0.000000000000000000, -1.000000000000000000, 0.000000000000000000 ) ) ;
#58068=B_SPLINE_CURVE_WITH_KNOTS ( 'NONE', 3,
 ( #65802, #46829, #20760, #46410 ),
 .UNSPECIFIED., .F., .F.,
 ( 4, 4 ),
 ( 0.1177794994733336598, 0.1192034014685218191 ),
 .UNSPECIFIED. ) ;
#58070=CARTESIAN_POINT ( 'NONE',  ( 0.000000000000000000, 0.000000000000000000, 0.000000000000000000 ) ) ;
#58086=AXIS2_PLACEMENT_3D ( 'NONE', #14371, #39174, #45479 ) ;
#58106=CARTESIAN_POINT ( 'NONE',  ( 0.4741708390789288186, 1.554782515222133954, -2.169554433241255520 ) ) ;
#58107=DIRECTION ( 'NONE',  ( 0.000000000000000000, -1.000000000000000000, 0.000000000000000000 ) ) ;
#58111=CARTESIAN_POINT ( 'NONE',  ( -0.03443470937339725840, 0.2755905511811023723, -1.320480459168889897 ) ) ;
#58118=ORIENTED_EDGE ( 'NONE', *, *, #12124, .F. ) ;
#58122=FACE_OUTER_BOUND ( 'NONE', #21845, .T. ) ;
#58133=CARTESIAN_POINT ( 'NONE',  ( -0.4314295484911011003, 1.339559522712173267, -2.086640540083727124 ) ) ;
#58142=CIRCLE ( 'NONE', #21878, 0.5118110236220472231 ) ;
#58153=CARTESIAN_POINT ( 'NONE',  ( -0.5314960629921325896, 2.755905511811024056, 1.895394334970790018 ) ) ;
#58154=VERTEX_POINT ( 'NONE', #64669 ) ;
#58155=EDGE_CURVE ( 'NONE', #12714, #82375, #26361, .T. ) ;
#58156=ORIENTED_EDGE ( 'NONE', *, *, #36314, .T. ) ;
#58166=CARTESIAN_POINT ( 'NONE',  ( 0.000000000000000000, 2.559055118110236560, 0.000000000000000000 ) ) ;
#58180=DIRECTION ( 'NONE',  ( 0.000000000000000000, 0.000000000000000000, -1.000000000000000000 ) ) ;
#58187=AXIS2_PLACEMENT_3D ( 'NONE', #39791, #41042, #34736 ) ;
#58196=DIRECTION ( 'NONE',  ( 0.000000000000000000, -0.000000000000000000, 1.000000000000000000 ) ) ;
#58210=EDGE_CURVE ( 'NONE', #66560, #29487, #59776, .T. ) ;
#58221=DIRECTION ( 'NONE',  ( -0.000000000000000000, -1.000000000000000000, -0.000000000000000000 ) ) ;
#58238=B_SPLINE_CURVE_WITH_KNOTS ( 'NONE', 3,
 ( #18292, #43937, #6058, #82674, #32145, #17478, #11151, #49439 ),
 .UNSPECIFIED., .F., .F.,
 ( 4, 2, 2, 4 ),
 ( 0.000000000000000000, 0.002428646466414857708, 0.003642969699622285694, 0.004857292932829714548 ),
 .UNSPECIFIED. ) ;
#58244=AXIS2_PLACEMENT_3D ( 'NONE', #39480, #33172, #78215 ) ;
#58252=EDGE_LOOP ( 'NONE', ( #38512, #37526, #13546, #41406, #68943 ) ) ;
#58258=CARTESIAN_POINT ( 'NONE',  ( 3.821484228344193657, 2.755905511811024056, 0.5314960629921260393 ) ) ;
#58261=CIRCLE ( 'NONE', #12558, 3.307086614173228689 ) ;
#58270=FACE_OUTER_BOUND ( 'NONE', #26466, .T. ) ;
#58276=CARTESIAN_POINT ( 'NONE',  ( -0.03443470937339728616, 1.062992125984252079, -1.537015892239756099 ) ) ;
#58291=ADVANCED_FACE ( 'NONE', ( #14176 ), #11483, .T. ) ;
#58303=AXIS2_PLACEMENT_3D ( 'NONE', #11600, #24619, #75984 ) ;
#58316=EDGE_CURVE ( 'NONE', #25219, #41276, #55801, .T. ) ;
#58336=EDGE_LOOP ( 'NONE', ( #53072, #5349, #21402, #13957 ) ) ;
#58353=ORIENTED_EDGE ( 'NONE', *, *, #61206, .T. ) ;
#58367=VECTOR ( 'NONE', #12855, 39.37007874015748143 ) ;
#58380=CARTESIAN_POINT ( 'NONE',  ( 0.000000000000000000, 0.000000000000000000, 0.000000000000000000 ) ) ;
#58407=CARTESIAN_POINT ( 'NONE',  ( 0.3149606299212183158, 2.165354330708661568, 3.937007874015792552 ) ) ;
#58413=DIRECTION ( 'NONE',  ( 0.000000000000000000, 0.000000000000000000, 1.000000000000000000 ) ) ;
#58428=ORIENTED_EDGE ( 'NONE', *, *, #72187, .T. ) ;
#58434=PLANE ( 'NONE',  #37811 ) ;
#58437=CARTESIAN_POINT ( 'NONE',  ( 0.1077553908667773369, 1.075127789244234577, -3.935562805465960601 ) ) ;
#58438=DIRECTION ( 'NONE',  ( -0.000000000000000000, 1.000000000000000000, -0.000000000000000000 ) ) ;
#58440=EDGE_CURVE ( 'NONE', #45259, #65182, #22554, .T. ) ;
#58442=VERTEX_POINT ( 'NONE', #53278 ) ;
#58443=AXIS2_PLACEMENT_3D ( 'NONE', #27949, #42230, #28779 ) ;
#58445=ORIENTED_EDGE ( 'NONE', *, *, #61841, .F. ) ;
#58451=EDGE_CURVE ( 'NONE', #65535, #5038, #62548, .T. ) ;
#58460=VERTEX_POINT ( 'NONE', #60435 ) ;
#58465=CARTESIAN_POINT ( 'NONE',  ( 2.554262525012262586, 1.528804020127598529, -0.4744094488188971281 ) ) ;
#58494=CARTESIAN_POINT ( 'NONE',  ( -2.575297182719626043, 1.629972608277043822, -0.4653577321740525741 ) ) ;
#58535=CARTESIAN_POINT ( 'NONE',  ( -0.4744094488188833059, 1.537401574803149984, -3.908320185825793658 ) ) ;
#58548=ORIENTED_EDGE ( 'NONE', *, *, #59446, .F. ) ;
#58552=DIRECTION ( 'NONE',  ( -1.000000000000000000, -0.000000000000000000, -0.000000000000000000 ) ) ;
#58554=DIRECTION ( 'NONE',  ( 0.000000000000000000, 0.000000000000000000, -1.000000000000000000 ) ) ;
#58580=CARTESIAN_POINT ( 'NONE',  ( -0.6299212598425059095, 1.724409448818897905, -3.937007874015764131 ) ) ;
#58582=LINE ( 'NONE', #39647, #38867 ) ;
#58593=CARTESIAN_POINT ( 'NONE',  ( 1.348312163386739426, 0.000000000000000000, 0.7386866130305692613 ) ) ;
#58606=CIRCLE ( 'NONE', #65365, 2.204724409448819422 ) ;
#58618=CARTESIAN_POINT ( 'NONE',  ( 1.063819296904228162, 1.224016087139557341, -0.3574819075361487797 ) ) ;
#58622=CARTESIAN_POINT ( 'NONE',  ( 0.2895750033033090975, 1.160328408095293806, 3.926430088202063295 ) ) ;
#58657=CARTESIAN_POINT ( 'NONE',  ( 0.4490604499032361252, 1.383603895493148883, 1.028280011760609458 ) ) ;
#58662=CIRCLE ( 'NONE', #69423, 0.09842519685039365085 ) ;
#58674=CARTESIAN_POINT ( 'NONE',  ( 0.3149606299212736049, 2.559055118110236560, -3.924389226575467404 ) ) ;
#58690=ORIENTED_EDGE ( 'NONE', *, *, #35732, .T. ) ;
#58694=DIRECTION ( 'NONE',  ( 0.000000000000000000, -0.000000000000000000, 1.000000000000000000 ) ) ;
#58695=DIRECTION ( 'NONE',  ( -1.000000000000000000, -0.000000000000000000, -0.000000000000000000 ) ) ;
#58701=DIRECTION ( 'NONE',  ( 1.000000000000000000, -0.000000000000000000, -0.000000000000000000 ) ) ;
#58706=EDGE_CURVE ( 'NONE', #78262, #21338, #61258, .T. ) ;
#58717=AXIS2_PLACEMENT_3D ( 'NONE', #9443, #35948, #81403 ) ;
#58720=AXIS2_PLACEMENT_3D ( 'NONE', #56569, #6475, #57801 ) ;
#58731=PRODUCT_DEFINITION_SHAPE ( 'NONE', 'NONE',  #25919 ) ;
#58761=ORIENTED_EDGE ( 'NONE', *, *, #55316, .F. ) ;
#58771=ADVANCED_FACE ( 'NONE', ( #80648 ), #48627, .F. ) ;
#58775=EDGE_CURVE ( 'NONE', #30834, #38086, #67246, .T. ) ;
#58779=ORIENTED_EDGE ( 'NONE', *, *, #28811, .F. ) ;
#58781=AXIS2_PLACEMENT_3D ( 'NONE', #58070, #436, #33670 ) ;
#58782=VERTEX_POINT ( 'NONE', #81882 ) ;
#58784=AXIS2_PLACEMENT_3D ( 'NONE', #65309, #33318, #491 ) ;
#58791=CARTESIAN_POINT ( 'NONE',  ( 1.348312163386739426, 0.000000000000000000, 0.5221511799597032821 ) ) ;
#58792=DIRECTION ( 'NONE',  ( 1.047444401652940007E-14, -0.000000000000000000, -1.000000000000000000 ) ) ;
#58801=ORIENTED_EDGE ( 'NONE', *, *, #70218, .T. ) ;
#58808=CARTESIAN_POINT ( 'NONE',  ( -2.158445410120303443, 1.605872332714554096, 0.4695140184743379907 ) ) ;
#58809=EDGE_CURVE ( 'NONE', #11181, #52658, #45027, .T. ) ;
#58817=CARTESIAN_POINT ( 'NONE',  ( 3.937007874015748143, 2.559055118110236560, 0.3149606299212599492 ) ) ;
#58857=FACE_OUTER_BOUND ( 'NONE', #67286, .T. ) ;
#58860=EDGE_CURVE ( 'NONE', #59294, #70804, #82287, .T. ) ;
#58866=CARTESIAN_POINT ( 'NONE',  ( 0.4585086550082259071, 1.414613662877127531, -3.910220139313873133 ) ) ;
#58872=ORIENTED_EDGE ( 'NONE', *, *, #52742, .F. ) ;
#58886=ORIENTED_EDGE ( 'NONE', *, *, #46015, .F. ) ;
#58901=CARTESIAN_POINT ( 'NONE',  ( 0.4744094488188839720, 1.537401574803149984, 3.908320185825793658 ) ) ;
#58919=LINE ( 'NONE', #63978, #81020 ) ;
#58937=DIRECTION ( 'NONE',  ( 1.047444401652940007E-14, -0.000000000000000000, -1.000000000000000000 ) ) ;
#58948=DIRECTION ( 'NONE',  ( -0.000000000000000000, -1.000000000000000000, -0.000000000000000000 ) ) ;
#58992=VERTEX_POINT ( 'NONE', #75563 ) ;
#59007=CARTESIAN_POINT ( 'NONE',  ( 3.910225209392130363, 1.414458570209803812, -0.4584652947720309069 ) ) ;
#59012=DIRECTION ( 'NONE',  ( 0.000000000000000000, 0.000000000000000000, 1.000000000000000000 ) ) ;
#59014=DIRECTION ( 'NONE',  ( -1.000000000000000000, -0.000000000000000000, -0.000000000000000000 ) ) ;
#59033=CARTESIAN_POINT ( 'NONE',  ( -3.937007874015748143, 2.165354330708662012, -0.6299212598425202314 ) ) ;
#59059=CARTESIAN_POINT ( 'NONE',  ( 0.000000000000000000, 2.755905511811024056, 0.000000000000000000 ) ) ;
#59078=DIRECTION ( 'NONE',  ( -0.000000000000000000, -1.000000000000000000, -0.000000000000000000 ) ) ;
#59096=ORIENTED_EDGE ( 'NONE', *, *, #25809, .T. ) ;
#59099=CARTESIAN_POINT ( 'NONE',  ( 1.348312163386739426, 0.2755905511811023723, 0.7386866130305692613 ) ) ;
#59102=CARTESIAN_POINT ( 'NONE',  ( -0.4257672537616706832, 1.326168777627700246, 2.647052616966094618 ) ) ;
#59103=CARTESIAN_POINT ( 'NONE',  ( -2.362204724409448620, 1.724409448818897905, -2.474278114140802984E-14 ) ) ;
#59111=CARTESIAN_POINT ( 'NONE',  ( -1.047434348705044815, 1.285715225710756249, -0.4024367083785531651 ) ) ;
#59113=CARTESIAN_POINT ( 'NONE',  ( -3.937007874015748143, 2.559055118110236560, -0.3149606299212599492 ) ) ;
#59114=CARTESIAN_POINT ( 'NONE',  ( 0.000000000000000000, 0.07874015748031502893, 3.858267716535433323 ) ) ;
#59116=ADVANCED_FACE ( 'NONE', ( #56586 ), #75971, .F. ) ;
#59120=CARTESIAN_POINT ( 'NONE',  ( -0.5314960629921194890, 2.742776589625216754, -1.881759000869286158 ) ) ;
#59135=B_SPLINE_CURVE_WITH_KNOTS ( 'NONE', 3,
 ( #65167, #46199, #71473, #13821 ),
 .UNSPECIFIED., .F., .F.,
 ( 4, 4 ),
 ( 0.09524935589747281217, 0.09667867193306639573 ),
 .UNSPECIFIED. ) ;
#59145=B_SPLINE_CURVE_WITH_KNOTS ( 'NONE', 3,
 ( #20844, #72195, #14550, #33884 ),
 .UNSPECIFIED., .F., .F.,
 ( 4, 4 ),
 ( 0.1307222445546318834, 0.1321409493595271933 ),
 .UNSPECIFIED. ) ;
#59165=CARTESIAN_POINT ( 'NONE',  ( 0.4102808022082901629, 1.299212598425196985, -1.736178228450289573 ) ) ;
#59176=ORIENTED_EDGE ( 'NONE', *, *, #8974, .T. ) ;
#59179=AXIS2_PLACEMENT_3D ( 'NONE', #22392, #72908, #16089 ) ;
#59192=ORIENTED_EDGE ( 'NONE', *, *, #48124, .T. ) ;
#59194=ORIENTED_EDGE ( 'NONE', *, *, #79456, .F. ) ;
#59202=DIRECTION ( 'NONE',  ( -1.000000000000000000, -0.000000000000000000, -0.000000000000000000 ) ) ;
#59240=CARTESIAN_POINT ( 'NONE',  ( -0.4359958488159683676, 1.724409448818897905, -1.033875059083678272 ) ) ;
#59242=DIRECTION ( 'NONE',  ( -0.000000000000000000, 0.000000000000000000, -1.000000000000000000 ) ) ;
#59259=FACE_OUTER_BOUND ( 'NONE', #50719, .T. ) ;
#59261=CARTESIAN_POINT ( 'NONE',  ( 0.4677827689124922084, 0.03937007874015747977, 2.154527559055118946 ) ) ;
#59265=CARTESIAN_POINT ( 'NONE',  ( 0.4732023222440338017, 1.572318554836809046, -2.557221887108173775 ) ) ;
#59270=DIRECTION ( 'NONE',  ( -2.664535259100375697E-15, 9.738798461624180871E-16, 1.000000000000000000 ) ) ;
#59274=DIRECTION ( 'NONE',  ( -0.000000000000000000, -1.000000000000000000, -0.000000000000000000 ) ) ;
#59278=ORIENTED_EDGE ( 'NONE', *, *, #890, .T. ) ;
#59290=B_SPLINE_CURVE_WITH_KNOTS ( 'NONE', 3,
 ( #29241, #22516, #15805, #74285, #23748, #81847, #80611, #4801, #75116, #17048, #11133, #67968, #73455, #56142, #9887, #74703, #10311, #42689, #54487, #55723, #80198, #36790, #48177, #49004, #41456, #73873, #3574, #3987, #55313, #35976, #81022, #24159 ),
 .UNSPECIFIED., .F., .F.,
 ( 4, 2, 2, 2, 2, 2, 2, 2, 2, 2, 2, 2, 2, 2, 2, 4 ),
 ( 0.03390883336407266024, 0.03455365212229282584, 0.03519847088051299144, 0.03648810839695332264, 0.03777774591339366078, 0.03906738342983399198, 0.04035702094627433012, 0.04164665846271466132, 0.04422593349559533066, 0.04680520852847600000, 0.04938448356135666933, 0.05067412107779700747, 0.05196375859423733867, 0.05325339611067767681, 0.05389821486889784241, 0.05454303362711801495 ),
 .UNSPECIFIED. ) ;
#59294=VERTEX_POINT ( 'NONE', #58674 ) ;
#59299=CARTESIAN_POINT ( 'NONE',  ( 2.554262525012302110, 1.537401574803149984, 0.4744094488188975722 ) ) ;
#59312=CARTESIAN_POINT ( 'NONE',  ( -2.620894764083836925, 1.710972922415817665, 0.4417590601942920636 ) ) ;
#59338=CARTESIAN_POINT ( 'NONE',  ( -0.5314960629921122726, 2.682389230697236115, -3.900966923095591010 ) ) ;
#59361=CARTESIAN_POINT ( 'NONE',  ( 1.348312163386739426, 1.062992125984252079, 0.7386866130305692613 ) ) ;
#59362=EDGE_LOOP ( 'NONE', ( #70224, #20472, #44981, #18223 ) ) ;
#59367=DIRECTION ( 'NONE',  ( 0.000000000000000000, 0.000000000000000000, -1.000000000000000000 ) ) ;
#59369=LINE ( 'NONE', #79177, #24291 ) ;
#59381=ORIENTED_EDGE ( 'NONE', *, *, #59829, .T. ) ;
#59409=EDGE_CURVE ( 'NONE', #40881, #66560, #80965, .T. ) ;
#59411=CARTESIAN_POINT ( 'NONE',  ( 1.348312163386739426, 1.062992125984252079, 0.6402614161801758463 ) ) ;
#59413=CARTESIAN_POINT ( 'NONE',  ( -0.5314960629921395840, 2.725419031863056674, 3.884512598959603658 ) ) ;
#59416=CARTESIAN_POINT ( 'NONE',  ( 3.929894648360968024, 1.125820779260225502, -0.2379601796926557877 ) ) ;
#59433=AXIS2_PLACEMENT_3D ( 'NONE', #48082, #22832, #48910 ) ;
#59438=ADVANCED_FACE ( 'NONE', ( #74650 ), #3652, .F. ) ;
#59446=EDGE_CURVE ( 'NONE', #42501, #34982, #37219, .T. ) ;
#59448=DIRECTION ( 'NONE',  ( -0.000000000000000000, -1.000000000000000000, -0.000000000000000000 ) ) ;
#59453=B_SPLINE_CURVE_WITH_KNOTS ( 'NONE', 3,
 ( #30134, #43163, #36867, #69686 ),
 .UNSPECIFIED., .F., .F.,
 ( 4, 4 ),
 ( 0.08702371034448116993, 0.08847090869701865201 ),
 .UNSPECIFIED. ) ;
#59456=CARTESIAN_POINT ( 'NONE',  ( 1.109416077537178191, 1.093657130816544143, -0.1685245874982175818 ) ) ;
#59481=AXIS2_PLACEMENT_3D ( 'NONE', #74769, #61712, #80678 ) ;
#59483=CARTESIAN_POINT ( 'NONE',  ( 0.4153800209585299386, 1.308165027668613645, -1.396905599340544368 ) ) ;
#59492=CARTESIAN_POINT ( 'NONE',  ( 0.1239713036211918251, 1.079207359476603845, 1.115280228140321350 ) ) ;
#59497=ADVANCED_FACE ( 'NONE', ( #49363 ), #43930, .F. ) ;
#59515=CARTESIAN_POINT ( 'NONE',  ( 0.4177787735907000366, 1.299212598425196985, -1.559171609364239375 ) ) ;
#59516=CARTESIAN_POINT ( 'NONE',  ( 1.348312163386739426, 0.2929341459200028863, 0.7386866130305692613 ) ) ;
#59524=CARTESIAN_POINT ( 'NONE',  ( 0.6299212598425337761, 1.724409448818898127, -3.886287458032460229 ) ) ;
#59527=DIRECTION ( 'NONE',  ( -1.000000000000000000, 0.000000000000000000, 0.000000000000000000 ) ) ;
#59560=DIRECTION ( 'NONE',  ( 0.000000000000000000, 0.000000000000000000, -1.000000000000000000 ) ) ;
#59580=CARTESIAN_POINT ( 'NONE',  ( 0.2850944291156183308, 1.158178041707070172, -1.676740862593898207 ) ) ;
#59631=CARTESIAN_POINT ( 'NONE',  ( 2.058019426306444633, 1.301092492065848649, -0.4123476441529899117 ) ) ;
#59638=DIRECTION ( 'NONE',  ( 1.049727191138618079E-16, -0.5150380749100549327, 0.8571673007021117785 ) ) ;
#59644=AXIS2_PLACEMENT_3D ( 'NONE', #67244, #73138, #52923 ) ;
#59655=CARTESIAN_POINT ( 'NONE',  ( 0.4468661194710661366, 1.378074791477804206, -1.523351412176985775 ) ) ;
#59665=ORIENTED_EDGE ( 'NONE', *, *, #10585, .F. ) ;
#59672=CARTESIAN_POINT ( 'NONE',  ( -3.908412016409563261, 1.506477424558240630, -0.4736547731912041925 ) ) ;
#59678=CARTESIAN_POINT ( 'NONE',  ( -3.846978723397335376, 2.751923335154144556, -0.5314960629921260393 ) ) ;
#59684=EDGE_CURVE ( 'NONE', #42693, #49366, #61590, .T. ) ;
#59687=CARTESIAN_POINT ( 'NONE',  ( -3.909107915504009600, 1.617412091359350823, 0.4678854304693115806 ) ) ;
#59688=CARTESIAN_POINT ( 'NONE',  ( 3.841955293929017135, 2.753420937170568461, 0.5314960629921260393 ) ) ;
#59692=VERTEX_POINT ( 'NONE', #48123 ) ;
#59697=VECTOR ( 'NONE', #22151, 39.37007874015748143 ) ;
#59709=ORIENTED_EDGE ( 'NONE', *, *, #67626, .F. ) ;
#59712=CARTESIAN_POINT ( 'NONE',  ( -1.397575190283976365, 1.210854158823307269, 0.3443910704722475402 ) ) ;
#59717=AXIS2_PLACEMENT_3D ( 'NONE', #43839, #36715, #30402 ) ;
#59753=CARTESIAN_POINT ( 'NONE',  ( -2.114058874202352278, 1.379859446982304894, -0.4477348144951664444 ) ) ;
#59763=AXIS2_PLACEMENT_3D ( 'NONE', #19569, #45228, #6942 ) ;
#59772=DIRECTION ( 'NONE',  ( 0.000000000000000000, 0.000000000000000000, -1.000000000000000000 ) ) ;
#59776=CIRCLE ( 'NONE', #8726, 3.937007874015748143 ) ;
#59783=CARTESIAN_POINT ( 'NONE',  ( -1.313877454013331780, 0.2929341459200028863, 0.7983292792091805090 ) ) ;
#59785=DIRECTION ( 'NONE',  ( -0.000000000000000000, 1.000000000000000000, -0.000000000000000000 ) ) ;
#59790=DIRECTION ( 'NONE',  ( 0.000000000000000000, 0.000000000000000000, -1.000000000000000000 ) ) ;
#59792=B_SPLINE_CURVE_WITH_KNOTS ( 'NONE', 3,
 ( #66656, #14896, #27925, #66237, #59492, #15311, #26677, #27089, #40974, #78460, #27507, #20785, #33416, #53164, #52332, #53583, #64985, #39722, #34245, #65414, #58657, #21200, #20368, #46020, #7751, #40556 ),
 .UNSPECIFIED., .F., .F.,
 ( 4, 2, 2, 2, 2, 2, 2, 2, 2, 2, 2, 2, 4 ),
 ( 0.000000000000000000, 0.002383993240623330772, 0.003575989860934996808, 0.004767986481246663279, 0.007151979721869992750, 0.008343976342181655750, 0.009535972962493319618, 0.01072796958280498696, 0.01191996620311664215, 0.01430395944373995254, 0.01549595606405161120, 0.01668795268436326987, 0.01907194592498655597 ),
 .UNSPECIFIED. ) ;
#59809=DIRECTION ( 'NONE',  ( -3.491481338843132961E-15, -0.000000000000000000, 1.000000000000000000 ) ) ;
#59812=ORIENTED_EDGE ( 'NONE', *, *, #36661, .F. ) ;
#59815=EDGE_LOOP ( 'NONE', ( #31927, #13414, #12184, #4519 ) ) ;
#59828=LINE ( 'NONE', #2182, #61209 ) ;
#59829=EDGE_CURVE ( 'NONE', #13254, #29189, #47704, .T. ) ;
#59834=CARTESIAN_POINT ( 'NONE',  ( 0.000000000000000000, 1.724409448818897905, 0.000000000000000000 ) ) ;
#59842=AXIS2_PLACEMENT_3D ( 'NONE', #52859, #46548, #72246 ) ;
#59852=CARTESIAN_POINT ( 'NONE',  ( -0.4705509983644061700, 1.475022898150550654, -1.018614094479749932 ) ) ;
#59878=CARTESIAN_POINT ( 'NONE',  ( -1.313877454013331780, 0.2755905511811023723, 0.9174237673981568975 ) ) ;
#59888=CARTESIAN_POINT ( 'NONE',  ( 0.000000000000000000, 1.724409448818897461, 0.000000000000000000 ) ) ;
#59891=EDGE_CURVE ( 'NONE', #6920, #2295, #51973, .T. ) ;
#59895=ORIENTED_EDGE ( 'NONE', *, *, #57575, .T. ) ;
#59902=EDGE_CURVE ( 'NONE', #34982, #53393, #29942, .T. ) ;
#59931=AXIS2_PLACEMENT_3D ( 'NONE', #47736, #16194, #28386 ) ;
#59933=CARTESIAN_POINT ( 'NONE',  ( 0.5314960629920920665, 2.729657717072965450, 3.237502119437994264 ) ) ;
#59941=CARTESIAN_POINT ( 'NONE',  ( -1.111574668186677162, 1.088302645458066875, -0.1536776283199748350 ) ) ;
#59948=VECTOR ( 'NONE', #38812, 39.37007874015748143 ) ;
#59951=CARTESIAN_POINT ( 'NONE',  ( -2.362204724409448620, 1.724409448818897461, -2.474278114140802984E-14 ) ) ;
#59970=ADVANCED_FACE ( 'NONE', ( #70371 ), #60113, .F. ) ;
#59977=LINE ( 'NONE', #15380, #9847 ) ;
#59983=VERTEX_POINT ( 'NONE', #56087 ) ;
#59988=AXIS2_PLACEMENT_3D ( 'NONE', #79439, #41121, #65567 ) ;
#59992=AXIS2_PLACEMENT_3D ( 'NONE', #51805, #82984, #50969 ) ;
#59993=AXIS2_PLACEMENT_3D ( 'NONE', #56673, #44854, #51177 ) ;
#60037=CARTESIAN_POINT ( 'NONE',  ( 1.827151616986590010, 2.742788234388597868, -0.5314960629921260393 ) ) ;
#60050=( NAMED_UNIT ( * ) PLANE_ANGLE_UNIT ( ) SI_UNIT ( $, .RADIAN. ) );
#60058=AXIS2_PLACEMENT_3D ( 'NONE', #61881, #67803, #47592 ) ;
#60078=CARTESIAN_POINT ( 'NONE',  ( 0.1273213304869930951, 0.000000000000000000, -1.680969278250197707 ) ) ;
#60079=EDGE_CURVE ( 'NONE', #24482, #31528, #49349, .T. ) ;
#60087=DIRECTION ( 'NONE',  ( 1.000000000000000000, -0.000000000000000000, -0.000000000000000000 ) ) ;
#60099=CARTESIAN_POINT ( 'NONE',  ( 0.4623158380715545746, 0.02617651024168222984, 2.142213561789874543 ) ) ;
#60102=CARTESIAN_POINT ( 'NONE',  ( -3.873860110281697189, 2.736617272820978553, -0.5314960629921261503 ) ) ;
#60113=CONICAL_SURFACE ( 'NONE', #30491, 0.1771653543307085410, 1.029744258676653645 ) ;
#60114=CARTESIAN_POINT ( 'NONE',  ( 3.856579543051780856, 2.748002881374839390, 0.5314960629921259283 ) ) ;
#60116=ORIENTED_EDGE ( 'NONE', *, *, #17653, .F. ) ;
#60132=EDGE_LOOP ( 'NONE', ( #74707, #35471, #70082, #23148, #72750, #35812 ) ) ;
#60137=CARTESIAN_POINT ( 'NONE',  ( 2.873826567705914936, 1.063196196511239977, 0.01636564761923926109 ) ) ;
#60150=CARTESIAN_POINT ( 'NONE',  ( 1.403614904275686858E-14, 1.537401574803149984, -3.937007874015761910 ) ) ;
#60173=ADVANCED_FACE ( 'NONE', ( #25748 ), #11906, .F. ) ;
#60174=AXIS2_PLACEMENT_3D ( 'NONE', #17690, #69019, #23568 ) ;
#60176=CARTESIAN_POINT ( 'NONE',  ( -2.170146923806555606, 1.528804020127598751, -0.4744094488188977388 ) ) ;
#60203=B_SPLINE_CURVE_WITH_KNOTS ( 'NONE', 3,
 ( #4962, #57106, #37763, #82801 ),
 .UNSPECIFIED., .F., .F.,
 ( 4, 4 ),
 ( 0.07469576999304877729, 0.07612553241189870534 ),
 .UNSPECIFIED. ) ;
#60204=ORIENTED_EDGE ( 'NONE', *, *, #75249, .F. ) ;
#60212=CARTESIAN_POINT ( 'NONE',  ( -2.362204724409448620, 0.000000000000000000, -2.474278114140802984E-14 ) ) ;
#60213=CARTESIAN_POINT ( 'NONE',  ( 6.267877318470707138E-17, 0.03937007874015751446, 2.874015748031495843 ) ) ;
#60217=VERTEX_POINT ( 'NONE', #56906 ) ;
#60232=B_SPLINE_CURVE_WITH_KNOTS ( 'NONE', 3,
 ( #40579, #59933, #60354, #16585 ),
 .UNSPECIFIED., .F., .F.,
 ( 4, 4 ),
 ( 0.1818586053348001663, 0.1832800580269407509 ),
 .UNSPECIFIED. ) ;
#60237=ORIENTED_EDGE ( 'NONE', *, *, #45798, .T. ) ;
#60240=ORIENTED_EDGE ( 'NONE', *, *, #34333, .F. ) ;
#60255=CARTESIAN_POINT ( 'NONE',  ( -0.5314960629921372526, 2.716535433070866645, 3.224202737261813834 ) ) ;
#60262=CARTESIAN_POINT ( 'NONE',  ( 0.000000000000000000, 2.755905511811024056, 0.000000000000000000 ) ) ;
#60268=CARTESIAN_POINT ( 'NONE',  ( -0.9285414500055709786, 2.165354330708662012, -0.6299212598425202314 ) ) ;
#60275=CARTESIAN_POINT ( 'NONE',  ( -0.4736394362785769641, 1.506176172253612000, -1.017181694652558699 ) ) ;
#60304=ADVANCED_FACE ( 'NONE', ( #18625 ), #32072, .T. ) ;
#60327=EDGE_CURVE ( 'NONE', #15966, #51592, #56014, .T. ) ;
#60330=DIRECTION ( 'NONE',  ( -0.000000000000000000, -1.000000000000000000, 0.000000000000000000 ) ) ;
#60347=EDGE_CURVE ( 'NONE', #36478, #63415, #23825, .T. ) ;
#60353=DIRECTION ( 'NONE',  ( -3.491481338843132961E-15, -0.000000000000000000, 1.000000000000000000 ) ) ;
#60354=CARTESIAN_POINT ( 'NONE',  ( 0.5314960629920919555, 2.742781089625999424, 3.250800428249180030 ) ) ;
#60361=EDGE_LOOP ( 'NONE', ( #50804, #2304, #80328, #68884, #67375, #6596, #64065, #71103, #73493, #68430, #213, #58779, #14276, #77943 ) ) ;
#60363=CARTESIAN_POINT ( 'NONE',  ( -1.057068326459881691, 1.248267542859002655, 0.3764357908784603524 ) ) ;
#60377=CARTESIAN_POINT ( 'NONE',  ( 2.630268417803912406, 1.724409448818900570, -0.4359958488159719758 ) ) ;
#60388=AXIS2_PLACEMENT_3D ( 'NONE', #12106, #81585, #56700 ) ;
#60402=VERTEX_POINT ( 'NONE', #45523 ) ;
#60417=DIRECTION ( 'NONE',  ( 0.000000000000000000, 0.000000000000000000, -1.000000000000000000 ) ) ;
#60435=CARTESIAN_POINT ( 'NONE',  ( 3.900966923095589678, 2.559055118110236560, -0.5314960629921260393 ) ) ;
#60447=ORIENTED_EDGE ( 'NONE', *, *, #3802, .F. ) ;
#60448=CARTESIAN_POINT ( 'NONE',  ( -1.526728978123871538, 1.379587654853634326, 0.4473998187889915434 ) ) ;
#60452=CARTESIAN_POINT ( 'NONE',  ( 1.017199299814982805, 1.569430237215018176, -0.4736019971540504914 ) ) ;
#60463=EDGE_LOOP ( 'NONE', ( #72241, #1962, #19986, #44389 ) ) ;
#60468=CARTESIAN_POINT ( 'NONE',  ( 2.113943251734093032, 1.379671404989100569, -0.4476723508032725563 ) ) ;
#60498=DIRECTION ( 'NONE',  ( 0.000000000000000000, 0.000000000000000000, -1.000000000000000000 ) ) ;
#60501=ORIENTED_EDGE ( 'NONE', *, *, #56208, .T. ) ;
#60504=EDGE_CURVE ( 'NONE', #13567, #23658, #78800, .T. ) ;
#60523=FACE_OUTER_BOUND ( 'NONE', #17701, .T. ) ;
#60525=CARTESIAN_POINT ( 'NONE',  ( 3.892840969167625786, 2.712230453466949687, 0.5314960629921260393 ) ) ;
#60527=EDGE_LOOP ( 'NONE', ( #4854, #62683, #34466, #55954, #27163, #523 ) ) ;
#60543=VERTEX_POINT ( 'NONE', #34168 ) ;
#60548=CARTESIAN_POINT ( 'NONE',  ( -1.510944988927603871, 1.132458528238634798, 0.2471620315916907840 ) ) ;
#60552=ADVANCED_FACE ( 'NONE', ( #32488 ), #52673, .F. ) ;
#60560=EDGE_LOOP ( 'NONE', ( #58801, #79914, #76983, #23913 ) ) ;
#60583=CONICAL_SURFACE ( 'NONE', #64598, 0.1190944881889763746, 0.8726646259971648778 ) ;
#60590=CARTESIAN_POINT ( 'NONE',  ( 0.5314960629920854052, 2.712196231959916659, 3.892860353355080072 ) ) ;
#60600=CIRCLE ( 'NONE', #51187, 0.1978346456692914035 ) ;
#60621=CARTESIAN_POINT ( 'NONE',  ( 0.6299212598424790421, 2.755905511811024056, 3.886287458032468667 ) ) ;
#60624=CARTESIAN_POINT ( 'NONE',  ( 0.4177787735907000366, 0.3937007874015748254, -1.559171609364239375 ) ) ;
#60631=VERTEX_POINT ( 'NONE', #2184 ) ;
#60639=VECTOR ( 'NONE', #43972, 39.37007874015748143 ) ;
#60643=CARTESIAN_POINT ( 'NONE',  ( 0.1807970329289269873, 1.098498331261034133, -2.841281961169017656 ) ) ;
#60646=ORIENTED_EDGE ( 'NONE', *, *, #45034, .T. ) ;
#60649=ORIENTED_EDGE ( 'NONE', *, *, #48765, .T. ) ;
#60684=CARTESIAN_POINT ( 'NONE',  ( 2.362204724409448620, 0.03937007874015751446, 8.247593713802677664E-15 ) ) ;
#60686=DIRECTION ( 'NONE',  ( -1.000000000000000000, -0.000000000000000000, -0.000000000000000000 ) ) ;
#60715=CARTESIAN_POINT ( 'NONE',  ( -1.733288081962263139, 1.252173825773542637, 0.3800872639956032750 ) ) ;
#60717=LINE ( 'NONE', #36690, #55396 ) ;
#60719=CARTESIAN_POINT ( 'NONE',  ( 2.170146923806634653, 1.537401574803149984, -0.4744094488188970171 ) ) ;
#60728=CARTESIAN_POINT ( 'NONE',  ( 3.900966923095589678, 2.677165354330708791, -0.5314960629921260393 ) ) ;
#60737=EDGE_CURVE ( 'NONE', #61368, #49776, #20861, .T. ) ;
#60739=CARTESIAN_POINT ( 'NONE',  ( 0.4477876756950379122, 1.694898206223995007, 3.911462694204230317 ) ) ;
#60752=CARTESIAN_POINT ( 'NONE',  ( -0.1341320108093635721, 1.082050302230251448, -2.856397811438244005 ) ) ;
#60754=AXIS2_PLACEMENT_3D ( 'NONE', #11033, #53978, #79690 ) ;
#60758=ORIENTED_EDGE ( 'NONE', *, *, #36242, .T. ) ;
#60763=CARTESIAN_POINT ( 'NONE',  ( 1.348312163386739426, 0.2929341459200028863, 0.7386866130305692613 ) ) ;
#60764=DIRECTION ( 'NONE',  ( 0.000000000000000000, -1.000000000000000000, 0.000000000000000000 ) ) ;
#60775=CARTESIAN_POINT ( 'NONE',  ( -0.5314960629921294810, 2.755905511811024056, 0.9881811337016621621 ) ) ;
#60779=DIRECTION ( 'NONE',  ( -0.000000000000000000, -1.000000000000000000, 0.000000000000000000 ) ) ;
#60780=FACE_OUTER_BOUND ( 'NONE', #55555, .T. ) ;
#60812=VERTEX_POINT ( 'NONE', #52255 ) ;
#60826=CARTESIAN_POINT ( 'NONE',  ( -1.559171609364246924, 0.3937007874015747699, 0.2199441279213821265 ) ) ;
#60855=VERTEX_POINT ( 'NONE', #20290 ) ;
#60858=CARTESIAN_POINT ( 'NONE',  ( -1.563876174483072035, 1.386417634015433942, 0.4497423439146382429 ) ) ;
#60863=DIRECTION ( 'NONE',  ( -0.000000000000000000, -1.000000000000000000, 0.000000000000000000 ) ) ;
#60872=CARTESIAN_POINT ( 'NONE',  ( 0.5314960629921394730, 2.712230453466948799, -3.892840969167623566 ) ) ;
#60873=EDGE_LOOP ( 'NONE', ( #6918, #57946, #56556, #2403, #14936, #82202, #78175, #23384, #63840, #7849 ) ) ;
#60880=EDGE_CURVE ( 'NONE', #20906, #75749, #50936, .T. ) ;
#60909=DIRECTION ( 'NONE',  ( 0.000000000000000000, 1.000000000000000000, 0.000000000000000000 ) ) ;
#60911=ORIENTED_EDGE ( 'NONE', *, *, #11099, .T. ) ;
#60939=ORIENTED_EDGE ( 'NONE', *, *, #68146, .T. ) ;
#60954=ORIENTED_EDGE ( 'NONE', *, *, #80559, .F. ) ;
#60968=ORIENTED_EDGE ( 'NONE', *, *, #63295, .F. ) ;
#61000=CARTESIAN_POINT ( 'NONE',  ( -1.923693779251843150, 1.143166703770554626, -0.2643333500026249783 ) ) ;
#61026=ORIENTED_EDGE ( 'NONE', *, *, #28821, .F. ) ;
#61031=CARTESIAN_POINT ( 'NONE',  ( 0.3118275472110223490, 1.179820887159493292, -1.417058425483740836 ) ) ;
#61037=DIRECTION ( 'NONE',  ( 0.000000000000000000, -1.000000000000000000, 0.000000000000000000 ) ) ;
#61038=CARTESIAN_POINT ( 'NONE',  ( 0.4744094488189011805, 1.537401574803149984, -1.016821367227981998 ) ) ;
#61043=AXIS2_PLACEMENT_3D ( 'NONE', #60624, #67783, #2974 ) ;
#61051=CARTESIAN_POINT ( 'NONE',  ( 0.03160120395398562099, 1.064035752752396258, -1.466227782781327926 ) ) ;
#61056=CARTESIAN_POINT ( 'NONE',  ( 0.08519462842576361328, 1.070400731138066552, -2.867154304459277991 ) ) ;
#61059=ORIENTED_EDGE ( 'NONE', *, *, #6668, .F. ) ;
#61089=CARTESIAN_POINT ( 'NONE',  ( 0.5314960629921373636, 2.742781085175769462, -3.250800423740331624 ) ) ;
#61096=CARTESIAN_POINT ( 'NONE',  ( -0.2391728406892293379, 1.126541202442033152, -1.096574649324438155 ) ) ;
#61128=DIRECTION ( 'NONE',  ( -3.491481338843132961E-15, -0.000000000000000000, 1.000000000000000000 ) ) ;
#61135=ORIENTED_EDGE ( 'NONE', *, *, #12124, .T. ) ;
#61156=CIRCLE ( 'NONE', #40981, 0.1978346456692914035 ) ;
#61165=CARTESIAN_POINT ( 'NONE',  ( -0.4725434569952416397, 1.494547573005089447, -2.558822519881354118 ) ) ;
#61170=ORIENTED_EDGE ( 'NONE', *, *, #13485, .T. ) ;
#61177=DIRECTION ( 'NONE',  ( -0.000000000000000000, 1.000000000000000000, -0.000000000000000000 ) ) ;
#61206=EDGE_CURVE ( 'NONE', #5989, #26718, #70927, .T. ) ;
#61209=VECTOR ( 'NONE', #16480, 39.37007874015748143 ) ;
#61223=LINE ( 'NONE', #10314, #429 ) ;
#61225=B_SPLINE_CURVE_WITH_KNOTS ( 'NONE', 3,
 ( #47814, #28878, #60452, #28049, #1559, #73929, #2804, #79838 ),
 .UNSPECIFIED., .F., .F.,
 ( 4, 2, 2, 4 ),
 ( 0.03812540793793221805, 0.03934516121038392905, 0.04056491448283564699, 0.04300442102773906899 ),
 .UNSPECIFIED. ) ;
#61238=B_SPLINE_CURVE_WITH_KNOTS ( 'NONE', 3,
 ( #22941, #35577, #48196, #28427 ),
 .UNSPECIFIED., .F., .F.,
 ( 4, 4 ),
 ( 0.09384283614957933395, 0.09527263441391617405 ),
 .UNSPECIFIED. ) ;
#61258=LINE ( 'NONE', #66345, #47752 ) ;
#61271=CARTESIAN_POINT ( 'NONE',  ( 0.000000000000000000, 1.724409448818897905, 0.000000000000000000 ) ) ;
#61272=CONICAL_SURFACE ( 'NONE', #77441, 0.1771653543307085410, 1.029744258676653645 ) ;
#61276=LINE ( 'NONE', #3629, #18208 ) ;
#61291=DIRECTION ( 'NONE',  ( 0.000000000000000000, 0.000000000000000000, -1.000000000000000000 ) ) ;
#61293=LINE ( 'NONE', #62539, #72132 ) ;
#61320=DIRECTION ( 'NONE',  ( 0.000000000000000000, 1.000000000000000000, 0.000000000000000000 ) ) ;
#61321=CYLINDRICAL_SURFACE ( 'NONE', #12600, 0.2165354330708660069 ) ;
#61326=CIRCLE ( 'NONE', #77499, 0.1771653543307085410 ) ;
#61336=ADVANCED_FACE ( 'NONE', ( #62379 ), #44243, .F. ) ;
#61346=CARTESIAN_POINT ( 'NONE',  ( -2.503252890251015828, 2.755905511811024056, -0.5314960629921260393 ) ) ;
#61363=EDGE_CURVE ( 'NONE', #55851, #7036, #21902, .T. ) ;
#61368=VERTEX_POINT ( 'NONE', #35895 ) ;
#61370=VECTOR ( 'NONE', #10140, 39.37007874015748143 ) ;
#61371=AXIS2_PLACEMENT_3D ( 'NONE', #77396, #58438, #19730 ) ;
#61380=CARTESIAN_POINT ( 'NONE',  ( -0.5314960629921395840, 2.755905511811024056, 3.900966923095588346 ) ) ;
#61385=VERTEX_POINT ( 'NONE', #37944 ) ;
#61408=LINE ( 'NONE', #15572, #57380 ) ;
#61422=LINE ( 'NONE', #8843, #21923 ) ;
#61424=AXIS2_PLACEMENT_3D ( 'NONE', #78426, #39688, #15277 ) ;
#61425=EDGE_CURVE ( 'NONE', #39595, #41210, #15794, .T. ) ;
#61434=VECTOR ( 'NONE', #36954, 39.37007874015748143 ) ;
#61444=ORIENTED_EDGE ( 'NONE', *, *, #25507, .T. ) ;
#61452=DIRECTION ( 'NONE',  ( 0.000000000000000000, 0.000000000000000000, 1.000000000000000000 ) ) ;
#61454=B_SPLINE_CURVE_WITH_KNOTS ( 'NONE', 3,
 ( #67084, #80556, #49361, #16156, #61165, #16574, #68731, #17405, #61998, #29185, #10668, #54853, #23277, #15748, #48529, #29592, #74229, #55665, #79725, #55255, #9416, #48947, #35086, #60752, #28769, #80141, #22463, #48121, #30417, #25330 ),
 .UNSPECIFIED., .F., .F.,
 ( 4, 2, 2, 2, 2, 2, 2, 2, 2, 2, 2, 2, 2, 2, 4 ),
 ( 0.005313729678161549161, 0.005969797177608808514, 0.006625864677056067867, 0.007937999675950588307, 0.009250134674845107013, 0.01056226967373962572, 0.01318653967152868742, 0.01581080966931774912, 0.01712294466821228170, 0.01843507966710681428, 0.02105934966489587251, 0.02237148466379040163, 0.02368361966268493074, 0.02499575466157945985, 0.02630788966047398897 ),
 .UNSPECIFIED. ) ;
#61457=ORIENTED_EDGE ( 'NONE', *, *, #22925, .F. ) ;
#61471=CARTESIAN_POINT ( 'NONE',  ( 0.4359958488159859646, 1.724409448818897905, -3.937007874015760578 ) ) ;
#61478=ORIENTED_EDGE ( 'NONE', *, *, #53988, .T. ) ;
#61498=CONICAL_SURFACE ( 'NONE', #38646, 0.1978346456692914035, 0.8726646259971685415 ) ;
#61504=ADVANCED_FACE ( 'NONE', ( #50971 ), #61498, .F. ) ;
#61511=EDGE_CURVE ( 'NONE', #5038, #65535, #27908, .T. ) ;
#61516=CARTESIAN_POINT ( 'NONE',  ( -0.4319747415000730895, 1.340679305999893600, -1.035581624764630115 ) ) ;
#61531=EDGE_CURVE ( 'NONE', #46748, #21089, #76668, .T. ) ;
#61533=DIRECTION ( 'NONE',  ( 0.000000000000000000, 0.000000000000000000, -1.000000000000000000 ) ) ;
#61559=ORIENTED_EDGE ( 'NONE', *, *, #15443, .T. ) ;
#61565=CARTESIAN_POINT ( 'NONE',  ( 0.000000000000000000, 0.000000000000000000, 0.000000000000000000 ) ) ;
#61574=CARTESIAN_POINT ( 'NONE',  ( 0.4744094488188839720, 1.537401574803149984, 3.908320185825793658 ) ) ;
#61588=LINE ( 'NONE', #68330, #78594 ) ;
#61590=LINE ( 'NONE', #9011, #65476 ) ;
#61593=ORIENTED_EDGE ( 'NONE', *, *, #47818, .F. ) ;
#61597=CARTESIAN_POINT ( 'NONE',  ( 0.5314960629921070545, 2.755905511811024056, 1.813482582612299110 ) ) ;
#61610=CARTESIAN_POINT ( 'NONE',  ( -1.016821367227983997, 1.537401574803149984, 0.4744094488188970171 ) ) ;
#61649=DIRECTION ( 'NONE',  ( 1.049727191138617093E-16, -0.5150380749100561539, 0.8571673007021108903 ) ) ;
#61651=ORIENTED_EDGE ( 'NONE', *, *, #24144, .F. ) ;
#61693=ORIENTED_EDGE ( 'NONE', *, *, #78869, .F. ) ;
#61695=ORIENTED_EDGE ( 'NONE', *, *, #53188, .F. ) ;
#61712=DIRECTION ( 'NONE',  ( -0.000000000000000000, -1.000000000000000000, -0.000000000000000000 ) ) ;
#61714=CARTESIAN_POINT ( 'NONE',  ( 2.167227123902291108, 1.572090529166659367, 0.4732185887570802829 ) ) ;
#61716=DIRECTION ( 'NONE',  ( 0.000000000000000000, 1.000000000000000000, 0.000000000000000000 ) ) ;
#61720=CARTESIAN_POINT ( 'NONE',  ( 1.141392835773559211, 0.000000000000000000, 0.8264322058523028147 ) ) ;
#61769=ORIENTED_EDGE ( 'NONE', *, *, #36314, .F. ) ;
#61781=EDGE_CURVE ( 'NONE', #73035, #27965, #74972, .T. ) ;
#61784=ORIENTED_EDGE ( 'NONE', *, *, #33853, .F. ) ;
#61786=ORIENTED_EDGE ( 'NONE', *, *, #33602, .F. ) ;
#61795=DIRECTION ( 'NONE',  ( 0.000000000000000000, 0.000000000000000000, -1.000000000000000000 ) ) ;
#61796=DIRECTION ( 'NONE',  ( 1.047444401652940007E-14, 0.000000000000000000, -1.000000000000000000 ) ) ;
#61802=PLANE ( 'NONE',  #45247 ) ;
#61803=ORIENTED_EDGE ( 'NONE', *, *, #48095, .F. ) ;
#61809=CARTESIAN_POINT ( 'NONE',  ( -0.2101607493002635163, 1.111797321395157967, 3.931418615208038148 ) ) ;
#61830=CARTESIAN_POINT ( 'NONE',  ( -1.877461585981332171, 1.092324130688954176, 0.1650676745532031753 ) ) ;
#61841=EDGE_CURVE ( 'NONE', #62412, #50709, #11771, .T. ) ;
#61848=DIRECTION ( 'NONE',  ( 0.8660254037844362651, 0.000000000000000000, 0.5000000000000041078 ) ) ;
#61854=CARTESIAN_POINT ( 'NONE',  ( -1.313877454013331780, 0.2755905511811023723, 0.7983292792091805090 ) ) ;
#61855=VERTEX_POINT ( 'NONE', #47586 ) ;
#61860=DIRECTION ( 'NONE',  ( 0.000000000000000000, -0.000000000000000000, -1.000000000000000000 ) ) ;
#61881=CARTESIAN_POINT ( 'NONE',  ( -1.313877454013331780, 1.062992125984252079, 0.7983292792091805090 ) ) ;
#61915=CARTESIAN_POINT ( 'NONE',  ( -3.937007874015748143, 2.755905511811024056, 0.5314960629921260393 ) ) ;
#61923=CARTESIAN_POINT ( 'NONE',  ( -2.847313777101077026, 1.091897865355362152, 0.1662078246829769568 ) ) ;
#61926=FACE_OUTER_BOUND ( 'NONE', #73904, .T. ) ;
#61946=CARTESIAN_POINT ( 'NONE',  ( -0.5314960629921171575, 2.729661165926052124, -2.530077622625179767 ) ) ;
#61955=AXIS2_PLACEMENT_3D ( 'NONE', #78166, #13350, #71846 ) ;
#61958=CARTESIAN_POINT ( 'NONE',  ( -1.704584837829988819, 1.183873793530418661, 0.3164211518737862217 ) ) ;
#61961=CARTESIAN_POINT ( 'NONE',  ( 2.170146923806633765, 1.554943921348592273, -0.4744094488188969616 ) ) ;
#61964=EDGE_CURVE ( 'NONE', #41007, #32917, #68999, .T. ) ;
#61973=EDGE_CURVE ( 'NONE', #68390, #7361, #81702, .T. ) ;
#61975=AXIS2_PLACEMENT_3D ( 'NONE', #18082, #31517, #82466 ) ;
#61976=CARTESIAN_POINT ( 'NONE',  ( -0.1540510737581029521, 1.087609530016003356, 1.111807356369383104 ) ) ;
#61998=CARTESIAN_POINT ( 'NONE',  ( -0.4567115769095945188, 1.408171547189569939, -2.593413219429640204 ) ) ;
#62004=ORIENTED_EDGE ( 'NONE', *, *, #78455, .T. ) ;
#62008=LINE ( 'NONE', #67504, #14252 ) ;
#62024=ADVANCED_FACE ( 'NONE', ( #55134 ), #30294, .F. ) ;
#62049=DIRECTION ( 'NONE',  ( 1.049727191138616477E-16, -0.5150380749100564870, 0.8571673007021107793 ) ) ;
#62056=DIRECTION ( 'NONE',  ( 0.000000000000000000, 0.000000000000000000, -1.000000000000000000 ) ) ;
#62074=CYLINDRICAL_SURFACE ( 'NONE', #64071, 0.1771653543307085410 ) ;
#62101=ORIENTED_EDGE ( 'NONE', *, *, #10568, .T. ) ;
#62103=ORIENTED_EDGE ( 'NONE', *, *, #80969, .T. ) ;
#62104=DIRECTION ( 'NONE',  ( 0.000000000000000000, -1.000000000000000000, 0.000000000000000000 ) ) ;
#62122=DIRECTION ( 'NONE',  ( 0.8660254037844361541, 0.000000000000000000, 0.5000000000000043299 ) ) ;
#62137=VECTOR ( 'NONE', #15710, 39.37007874015748143 ) ;
#62149=CARTESIAN_POINT ( 'NONE',  ( -3.842312626974349943, 2.753838553078471918, 0.5314960629921259283 ) ) ;
#62153=B_SPLINE_CURVE_WITH_KNOTS ( 'NONE', 3,
 ( #41814, #35096, #67097, #74241, #73829, #47711, #54863, #29196 ),
 .UNSPECIFIED., .F., .F.,
 ( 4, 2, 2, 4 ),
 ( 0.03770802486988160396, 0.04014025118898163075, 0.04135636434853164067, 0.04257247750808165060 ),
 .UNSPECIFIED. ) ;
#62169=LINE ( 'NONE', #31829, #25111 ) ;
#62179=ORIENTED_EDGE ( 'NONE', *, *, #63459, .T. ) ;
#62209=CARTESIAN_POINT ( 'NONE',  ( 3.923644508792730523, 1.190792352294606449, 0.3242919053828030584 ) ) ;
#62232=CONICAL_SURFACE ( 'NONE', #55488, 1.244489337948955221, 0.7853981633974452814 ) ;
#62239=CARTESIAN_POINT ( 'NONE',  ( 2.094141031014959520, 1.724409448818898127, 0.4359958488159723644 ) ) ;
#62286=DIRECTION ( 'NONE',  ( 0.000000000000000000, 0.000000000000000000, -1.000000000000000000 ) ) ;
#62290=DIRECTION ( 'NONE',  ( -0.8660254037844432595, 0.000000000000000000, 0.4999999999999918954 ) ) ;
#62294=ORIENTED_EDGE ( 'NONE', *, *, #33188, .T. ) ;
#62323=CARTESIAN_POINT ( 'NONE',  ( 0.4744094488189113945, 1.537401574803149984, -3.937007874015760578 ) ) ;
#62327=DIRECTION ( 'NONE',  ( -0.000000000000000000, -1.000000000000000000, -0.000000000000000000 ) ) ;
#62330=CARTESIAN_POINT ( 'NONE',  ( -2.777177547361640908, 1.169463170161808785, -0.3010181502270431464 ) ) ;
#62333=CARTESIAN_POINT ( 'NONE',  ( -0.04537753515110386909, 1.065137975676527349, -1.631395471344458503 ) ) ;
#62345=CIRCLE ( 'NONE', #74504, 2.598425196850393970 ) ;
#62348=FACE_OUTER_BOUND ( 'NONE', #19012, .T. ) ;
#62356=AXIS2_PLACEMENT_3D ( 'NONE', #3481, #16121, #28735 ) ;
#62364=LINE ( 'NONE', #23238, #24515 ) ;
#62379=FACE_OUTER_BOUND ( 'NONE', #22873, .T. ) ;
#62391=DIRECTION ( 'NONE',  ( -0.000000000000000000, -1.000000000000000000, -0.000000000000000000 ) ) ;
#62410=ORIENTED_EDGE ( 'NONE', *, *, #43225, .T. ) ;
#62411=ADVANCED_FACE ( 'NONE', ( #43732 ), #42510, .F. ) ;
#62412=VERTEX_POINT ( 'NONE', #48826 ) ;
#62415=DIRECTION ( 'NONE',  ( -1.000000000000000000, 0.000000000000000000, -0.000000000000000000 ) ) ;
#62416=FACE_OUTER_BOUND ( 'NONE', #43626, .T. ) ;
#62418=CARTESIAN_POINT ( 'NONE',  ( 3.886287458032462006, 2.165354330708662012, 0.6299212598425202314 ) ) ;
#62419=( LENGTH_UNIT ( ) NAMED_UNIT ( * ) SI_UNIT ( $, .METRE. ) );
#62441=B_SPLINE_CURVE_WITH_KNOTS ( 'NONE', 3,
 ( #32522, #57767, #6852, #19907, #27463, #53121, #72505, #45134, #71253, #7275, #39679, #7706 ),
 .UNSPECIFIED., .F., .F.,
 ( 4, 2, 2, 2, 2, 4 ),
 ( 0.007992874908875454570, 0.009303755029337567456, 0.01061463514979968034, 0.01192551527026179323, 0.01258095533049286008, 0.01323639539072392693 ),
 .UNSPECIFIED. ) ;
#62444=DIRECTION ( 'NONE',  ( 0.000000000000000000, 0.000000000000000000, -1.000000000000000000 ) ) ;
#62452=CARTESIAN_POINT ( 'NONE',  ( 2.571961977011526290, 1.622068519643039330, 0.4668652553835664909 ) ) ;
#62486=CARTESIAN_POINT ( 'NONE',  ( -0.5314960629921194890, 2.716535433070866645, -1.854472803289054283 ) ) ;
#62524=CARTESIAN_POINT ( 'NONE',  ( -0.5314960629921148261, 2.729659931386287042, -3.210901110887978582 ) ) ;
#62539=CARTESIAN_POINT ( 'NONE',  ( 0.4744094488189113945, 1.537401574803149984, -3.937007874015760578 ) ) ;
#62543=CARTESIAN_POINT ( 'NONE',  ( 3.937007874015748143, 1.537401574803149984, -0.4744094488188970171 ) ) ;
#62548=CIRCLE ( 'NONE', #725, 0.1771653543307085410 ) ;
#62552=EDGE_CURVE ( 'NONE', #17178, #36023, #33267, .T. ) ;
#62570=VERTEX_POINT ( 'NONE', #5047 ) ;
#62577=CARTESIAN_POINT ( 'NONE',  ( 3.937007874015748143, 2.165354330708661568, 0.3149606299212600047 ) ) ;
#62582=CARTESIAN_POINT ( 'NONE',  ( 0.4671901501889602626, 1.453473631083803674, 2.571356120034363091 ) ) ;
#62596=ORIENTED_EDGE ( 'NONE', *, *, #42203, .T. ) ;
#62617=DIRECTION ( 'NONE',  ( 0.000000000000000000, 1.000000000000000000, 0.000000000000000000 ) ) ;
#62623=DIRECTION ( 'NONE',  ( 0.000000000000000000, 0.000000000000000000, 1.000000000000000000 ) ) ;
#62627=CARTESIAN_POINT ( 'NONE',  ( 3.908697805448793972, 1.475019653495670546, 0.4713285578992283953 ) ) ;
#62629=ORIENTED_EDGE ( 'NONE', *, *, #733, .F. ) ;
#62632=ORIENTED_EDGE ( 'NONE', *, *, #39907, .F. ) ;
#62638=CARTESIAN_POINT ( 'NONE',  ( -0.4109299095364690735, 1.299823618673216830, 3.915510462780284140 ) ) ;
#62649=EDGE_CURVE ( 'NONE', #55865, #49969, #63116, .T. ) ;
#62656=CARTESIAN_POINT ( 'NONE',  ( -3.224202737261815166, 2.716535433070866645, -0.5314960629921260393 ) ) ;
#62660=CARTESIAN_POINT ( 'NONE',  ( -1.901586028222560953, 1.118719813955022069, 0.2236424093447385852 ) ) ;
#62678=CARTESIAN_POINT ( 'NONE',  ( -3.929911103084700486, 1.125660643012857731, 0.2377022791102254007 ) ) ;
#62683=ORIENTED_EDGE ( 'NONE', *, *, #21285, .T. ) ;
#62692=DIRECTION ( 'NONE',  ( 0.000000000000000000, 1.000000000000000000, 0.000000000000000000 ) ) ;
#62693=AXIS2_PLACEMENT_3D ( 'NONE', #27132, #58701, #47313 ) ;
#62699=ORIENTED_EDGE ( 'NONE', *, *, #25507, .F. ) ;
#62709=CARTESIAN_POINT ( 'NONE',  ( -1.559171609364246924, 0.3937007874015747699, 0.4177787735906735578 ) ) ;
#62713=CARTESIAN_POINT ( 'NONE',  ( 0.4744094488189065095, 1.537401574803149984, -2.554262525012259477 ) ) ;
#62716=VERTEX_POINT ( 'NONE', #70246 ) ;
#62720=CIRCLE ( 'NONE', #6225, 1.198416298106748767 ) ;
#62746=EDGE_CURVE ( 'NONE', #55552, #20068, #65537, .T. ) ;
#62755=CARTESIAN_POINT ( 'NONE',  ( -2.571257611060566717, 1.453715418023197703, -0.4672341690643354584 ) ) ;
#62758=AXIS2_PLACEMENT_3D ( 'NONE', #1207, #39489, #52096 ) ;
#62759=CARTESIAN_POINT ( 'NONE',  ( -0.04553727834043951039, 1.065153152349019416, -1.442679039838661303 ) ) ;
#62763=VECTOR ( 'NONE', #16158, 39.37007874015748143 ) ;
#62764=AXIS2_PLACEMENT_3D ( 'NONE', #31312, #50255, #49845 ) ;
#62774=CARTESIAN_POINT ( 'NONE',  ( 2.362204724409448620, 1.929133858267716661, 0.5118110236220555498 ) ) ;
#62779=CARTESIAN_POINT ( 'NONE',  ( -1.033875059083676717, 1.724409448818897905, -0.4359958488159722534 ) ) ;
#62800=ORIENTED_EDGE ( 'NONE', *, *, #35790, .F. ) ;
#62805=FACE_OUTER_BOUND ( 'NONE', #7243, .T. ) ;
#62816=VECTOR ( 'NONE', #20207, 39.37007874015748143 ) ;
#62817=DIRECTION ( 'NONE',  ( 0.000000000000000000, 0.000000000000000000, -1.000000000000000000 ) ) ;
#62818=ORIENTED_EDGE ( 'NONE', *, *, #9419, .F. ) ;
#62833=DIRECTION ( 'NONE',  ( 0.000000000000000000, 0.000000000000000000, 1.000000000000000000 ) ) ;
#62836=ORIENTED_EDGE ( 'NONE', *, *, #77984, .F. ) ;
#62840=DIRECTION ( 'NONE',  ( -0.000000000000000000, -1.000000000000000000, -0.000000000000000000 ) ) ;
#62857=DIRECTION ( 'NONE',  ( -1.000000000000000000, 0.000000000000000000, -0.000000000000000000 ) ) ;
#62861=CARTESIAN_POINT ( 'NONE',  ( 0.5314960629920847390, 2.755905511811024056, 3.937007874015794773 ) ) ;
#62891=EDGE_CURVE ( 'NONE', #58154, #9606, #80092, .T. ) ;
#62903=CARTESIAN_POINT ( 'NONE',  ( 3.937007874015748143, 1.724409448818897905, -0.4359958488159719758 ) ) ;
#62911=B_SPLINE_CURVE_WITH_KNOTS ( 'NONE', 3,
 ( #12943, #73098, #28472, #34381, #54133, #15031, #80265, #8710, #8295, #47824, #15874, #40687, #60872, #35210, #72683, #79848 ),
 .UNSPECIFIED., .F., .F.,
 ( 4, 2, 2, 2, 2, 2, 2, 4 ),
 ( 0.000000000000000000, 0.0003923911760484576224, 0.0007847823520969152448, 0.001177173528145373030, 0.001569564704193830490, 0.001961955880242287949, 0.002354347056290746060, 0.003139129408387677025 ),
 .UNSPECIFIED. ) ;
#62933=VERTEX_POINT ( 'NONE', #3468 ) ;
#62942=CARTESIAN_POINT ( 'NONE',  ( 0.000000000000000000, 0.07874015748031502893, -3.937007874015748143 ) ) ;
#62949=ORIENTED_EDGE ( 'NONE', *, *, #25177, .F. ) ;
#62954=CARTESIAN_POINT ( 'NONE',  ( 2.152711368484104604, 1.622209144264168845, 0.4670403427556030218 ) ) ;
#62958=ORIENTED_EDGE ( 'NONE', *, *, #67735, .T. ) ;
#62996=CARTESIAN_POINT ( 'NONE',  ( 0.2772244525506746826, 1.152387065982276360, -1.451133023321481419 ) ) ;
#63000=LINE ( 'NONE', #57075, #3827 ) ;
#63011=ORIENTED_EDGE ( 'NONE', *, *, #77836, .F. ) ;
#63016=EDGE_CURVE ( 'NONE', #47922, #7036, #2447, .T. ) ;
#63023=EDGE_LOOP ( 'NONE', ( #62596, #28212 ) ) ;
#63043=ORIENTED_EDGE ( 'NONE', *, *, #44641, .T. ) ;
#63070=DIRECTION ( 'NONE',  ( 0.000000000000000000, 0.000000000000000000, 1.000000000000000000 ) ) ;
#63088=CARTESIAN_POINT ( 'NONE',  ( -3.910221821200592363, 1.414556597369199586, 0.4584944303835873369 ) ) ;
#63093=CYLINDRICAL_SURFACE ( 'NONE', #52854, 0.5118110236220471121 ) ;
#63094=EDGE_LOOP ( 'NONE', ( #12317, #6164 ) ) ;
#63095=FACE_OUTER_BOUND ( 'NONE', #14706, .T. ) ;
#63103=CARTESIAN_POINT ( 'NONE',  ( 0.000000000000000000, 2.755905511811024056, 0.000000000000000000 ) ) ;
#63110=ORIENTED_EDGE ( 'NONE', *, *, #34659, .T. ) ;
#63116=LINE ( 'NONE', #48410, #7735 ) ;
#63120=CARTESIAN_POINT ( 'NONE',  ( 0.3635064842674253227, 1.231191414405742535, -2.723505603036860734 ) ) ;
#63125=ORIENTED_EDGE ( 'NONE', *, *, #22, .F. ) ;
#63127=CARTESIAN_POINT ( 'NONE',  ( 2.829146054566470614, 1.111778211650228609, -0.2101609992702737073 ) ) ;
#63155=CARTESIAN_POINT ( 'NONE',  ( -0.5314960629921396951, 2.559055118110236560, 3.900966923095587457 ) ) ;
#63157=B_SPLINE_CURVE_WITH_KNOTS ( 'NONE', 3,
 ( #52914, #72714, #39895, #29638, #7916, #4380, #33577, #59240 ),
 .UNSPECIFIED., .F., .F.,
 ( 4, 2, 2, 4 ),
 ( 0.03812540793793221111, 0.03934516121038392211, 0.04056491448283564005, 0.04300442102773906206 ),
 .UNSPECIFIED. ) ;
#63159=CARTESIAN_POINT ( 'NONE',  ( -2.565164815102350282, 1.469861850861822195, -0.4698711669589719642 ) ) ;
#63172=CARTESIAN_POINT ( 'NONE',  ( 0.3132322334736995506, 1.180770478131392354, -1.077509718351006063 ) ) ;
#63180=CARTESIAN_POINT ( 'NONE',  ( -0.06215494498385511213, 1.066821167736317966, -3.936548014160229148 ) ) ;
#63199=EDGE_CURVE ( 'NONE', #4444, #8202, #46930, .T. ) ;
#63201=VERTEX_POINT ( 'NONE', #42170 ) ;
#63204=VECTOR ( 'NONE', #59014, 39.37007874015748143 ) ;
#63222=ORIENTED_EDGE ( 'NONE', *, *, #70277, .T. ) ;
#63232=DIRECTION ( 'NONE',  ( -1.000000000000000000, -0.000000000000000000, -0.000000000000000000 ) ) ;
#63238=ORIENTED_EDGE ( 'NONE', *, *, #22805, .T. ) ;
#63242=CARTESIAN_POINT ( 'NONE',  ( 0.5314960629921325896, 2.742776584231126247, -1.881758995267129642 ) ) ;
#63245=( NAMED_UNIT ( * ) SI_UNIT ( $, .STERADIAN. ) SOLID_ANGLE_UNIT ( ) );
#63265=LINE ( 'NONE', #68767, #77420 ) ;
#63275=CARTESIAN_POINT ( 'NONE',  ( 1.074111983884923571, 1.191141316951608076, 0.3246562585368536480 ) ) ;
#63291=VECTOR ( 'NONE', #26029, 39.37007874015748143 ) ;
#63295=EDGE_CURVE ( 'NONE', #6920, #3121, #76020, .T. ) ;
#63343=DIRECTION ( 'NONE',  ( 0.000000000000000000, 0.000000000000000000, -1.000000000000000000 ) ) ;
#63351=VECTOR ( 'NONE', #69058, 39.37007874015748143 ) ;
#63352=ORIENTED_EDGE ( 'NONE', *, *, #7798, .F. ) ;
#63414=VERTEX_POINT ( 'NONE', #49719 ) ;
#63415=VERTEX_POINT ( 'NONE', #62779 ) ;
#63425=ADVANCED_FACE ( 'NONE', ( #31184 ), #26590, .T. ) ;
#63426=EDGE_CURVE ( 'NONE', #33327, #55113, #5518, .T. ) ;
#63429=EDGE_LOOP ( 'NONE', ( #71318, #28855, #67176, #58690 ) ) ;
#63441=CARTESIAN_POINT ( 'NONE',  ( 1.392101432702376629, 0.000000000000000000, 0.9507481457704560768 ) ) ;
#63449=CARTESIAN_POINT ( 'NONE',  ( -0.5314960629921171575, 2.716535433070866645, -2.543486866223390930 ) ) ;
#63453=CIRCLE ( 'NONE', #67496, 3.937007874015748143 ) ;
#63458=CARTESIAN_POINT ( 'NONE',  ( 4.821444091131311894E-16, 0.07874015748031502893, 3.937007874015748143 ) ) ;
#63459=EDGE_CURVE ( 'NONE', #7122, #23435, #29786, .T. ) ;
#63467=ADVANCED_FACE ( 'NONE', ( #13095 ), #33331, .F. ) ;
#63478=B_SPLINE_CURVE_WITH_KNOTS ( 'NONE', 3,
 ( #39764, #33458, #59120, #1477 ),
 .UNSPECIFIED., .F., .F.,
 ( 4, 4 ),
 ( 0.1211256351025462169, 0.1225682571257921682 ),
 .UNSPECIFIED. ) ;
#63479=CARTESIAN_POINT ( 'NONE',  ( -3.924389226575468737, 2.559055118110236560, -0.3149606299212599492 ) ) ;
#63487=DIRECTION ( 'NONE',  ( 0.000000000000000000, 0.000000000000000000, -1.000000000000000000 ) ) ;
#63502=CIRCLE ( 'NONE', #35343, 3.937007874015748143 ) ;
#63504=EDGE_LOOP ( 'NONE', ( #64467, #20387 ) ) ;
#63505=CARTESIAN_POINT ( 'NONE',  ( -3.886287458032462006, 2.755905511811024056, 0.6299212598425196763 ) ) ;
#63507=VECTOR ( 'NONE', #35186, 39.37007874015748143 ) ;
#63509=EDGE_CURVE ( 'NONE', #5361, #50786, #32018, .T. ) ;
#63515=CARTESIAN_POINT ( 'NONE',  ( 0.4744094488189113945, 1.537401574803149984, -3.937007874015760578 ) ) ;
#63521=ORIENTED_EDGE ( 'NONE', *, *, #25905, .T. ) ;
#63531=CARTESIAN_POINT ( 'NONE',  ( 0.4044922606986875446, 1.289103360985770941, -2.676033440910250860 ) ) ;
#63538=CARTESIAN_POINT ( 'NONE',  ( 2.565212732165838450, 1.469708627452554595, -0.4698506773045480478 ) ) ;
#63554=EDGE_CURVE ( 'NONE', #21629, #9606, #68297, .T. ) ;
#63570=CARTESIAN_POINT ( 'NONE',  ( -2.558801921130022805, 1.494646310179101656, -0.4725519687354814979 ) ) ;
#63583=CARTESIAN_POINT ( 'NONE',  ( 0.4712520375767828007, 1.474486464701640021, -1.018310922256620676 ) ) ;
#63587=DIRECTION ( 'NONE',  ( -3.491481338843133355E-15, -0.000000000000000000, 1.000000000000000000 ) ) ;
#63597=DIRECTION ( 'NONE',  ( -0.000000000000000000, -1.000000000000000000, -0.000000000000000000 ) ) ;
#63605=DIRECTION ( 'NONE',  ( -0.8660254037844433705, 0.000000000000000000, 0.4999999999999920064 ) ) ;
#63619=CARTESIAN_POINT ( 'NONE',  ( -1.559171609364246924, 1.128537896298103416, 0.2406134192599649890 ) ) ;
#63630=CYLINDRICAL_SURFACE ( 'NONE', #12675, 0.2165354330708660624 ) ;
#63634=ORIENTED_EDGE ( 'NONE', *, *, #18368, .T. ) ;
#63662=CIRCLE ( 'NONE', #59644, 2.165354330708661568 ) ;
#63673=CARTESIAN_POINT ( 'NONE',  ( 0.000000000000000000, 1.724409448818897461, 0.000000000000000000 ) ) ;
#63678=CIRCLE ( 'NONE', #81195, 3.228346456692913424 ) ;
#63679=LINE ( 'NONE', #62861, #78550 ) ;
#63731=CIRCLE ( 'NONE', #27461, 0.3149606299212598381 ) ;
#63747=ORIENTED_EDGE ( 'NONE', *, *, #5614, .F. ) ;
#63748=FACE_OUTER_BOUND ( 'NONE', #65105, .T. ) ;
#63752=FACE_OUTER_BOUND ( 'NONE', #80434, .T. ) ;
#63760=ORIENTED_EDGE ( 'NONE', *, *, #22925, .T. ) ;
#63761=CARTESIAN_POINT ( 'NONE',  ( 0.000000000000000000, 1.724409448818897905, 2.362204724409448620 ) ) ;
#63769=ORIENTED_EDGE ( 'NONE', *, *, #72539, .F. ) ;
#63778=CONICAL_SURFACE ( 'NONE', #7310, 0.09842519685039351207, 1.029744258676652091 ) ;
#63790=AXIS2_PLACEMENT_3D ( 'NONE', #63103, #62692, #5034 ) ;
#63798=ORIENTED_EDGE ( 'NONE', *, *, #30238, .T. ) ;
#63812=DIRECTION ( 'NONE',  ( 0.000000000000000000, -1.000000000000000000, 0.000000000000000000 ) ) ;
#63824=ORIENTED_EDGE ( 'NONE', *, *, #41919, .F. ) ;
#63827=EDGE_CURVE ( 'NONE', #11296, #29599, #52093, .T. ) ;
#63840=ORIENTED_EDGE ( 'NONE', *, *, #33956, .F. ) ;
#63853=CARTESIAN_POINT ( 'NONE',  ( 3.264097702071373064, 2.755905511811024056, 0.5314960629921260393 ) ) ;
#63859=CARTESIAN_POINT ( 'NONE',  ( 0.4177787735907000366, 0.000000000000000000, -1.559171609364239375 ) ) ;
#63867=CARTESIAN_POINT ( 'NONE',  ( -0.4736532623569962297, 1.506389555808205660, 3.908412207303153973 ) ) ;
#63889=CARTESIAN_POINT ( 'NONE',  ( -3.937007874015748143, 1.724409448818897905, -0.4359958488159722534 ) ) ;
#63907=CARTESIAN_POINT ( 'NONE',  ( -3.937006426163500716, 1.063004141356476140, 0.03136679951920979398 ) ) ;
#63912=CARTESIAN_POINT ( 'NONE',  ( -0.4702989522381291199, 1.601790779910749807, 1.018730689361767583 ) ) ;
#63914=VERTEX_POINT ( 'NONE', #459 ) ;
#63915=CARTESIAN_POINT ( 'NONE',  ( 0.4177787735906991484, 1.312623414240987163, -1.404325600637324367 ) ) ;
#63922=EDGE_CURVE ( 'NONE', #45375, #3191, #66922, .T. ) ;
#63949=AXIS2_PLACEMENT_3D ( 'NONE', #66709, #9042, #6437 ) ;
#63950=CARTESIAN_POINT ( 'NONE',  ( 2.647193076292333025, 1.325969025732682605, -0.4256800600601902684 ) ) ;
#63978=CARTESIAN_POINT ( 'NONE',  ( -2.362204724409448620, 1.929133858267716661, 0.5118110236220224651 ) ) ;
#63981=DIRECTION ( 'NONE',  ( 0.000000000000000000, 1.000000000000000000, 0.000000000000000000 ) ) ;
#63998=CARTESIAN_POINT ( 'NONE',  ( 0.4426497960380878505, 1.366130357955170016, -2.105050863655339111 ) ) ;
#64004=CIRCLE ( 'NONE', #43865, 0.07874015748031502893 ) ;
#64006=CARTESIAN_POINT ( 'NONE',  ( -0.4501861592487448327, 1.384549727180958811, -3.911202737410993890 ) ) ;
#64023=DIRECTION ( 'NONE',  ( 0.000000000000000000, 0.000000000000000000, 1.000000000000000000 ) ) ;
#64028=ORIENTED_EDGE ( 'NONE', *, *, #55811, .F. ) ;
#64034=DIRECTION ( 'NONE',  ( -0.000000000000000000, -1.000000000000000000, -0.000000000000000000 ) ) ;
#64036=CARTESIAN_POINT ( 'NONE',  ( 0.4177787735907000366, 0.4110443821404751730, -1.559171609364239375 ) ) ;
#64044=DIRECTION ( 'NONE',  ( -0.000000000000000000, -1.000000000000000000, -0.000000000000000000 ) ) ;
#64046=VERTEX_POINT ( 'NONE', #52198 ) ;
#64058=EDGE_CURVE ( 'NONE', #45287, #27710, #65276, .T. ) ;
#64065=ORIENTED_EDGE ( 'NONE', *, *, #32224, .T. ) ;
#64067=CONICAL_SURFACE ( 'NONE', #70805, 3.444881889763779625, 0.7853981633974500554 ) ;
#64070=VECTOR ( 'NONE', #59809, 39.37007874015748143 ) ;
#64071=AXIS2_PLACEMENT_3D ( 'NONE', #17069, #23768, #60417 ) ;
#64096=CARTESIAN_POINT ( 'NONE',  ( -0.4567021909596216678, 1.408136488465067782, 2.130977159290117662 ) ) ;
#64100=EDGE_CURVE ( 'NONE', #68995, #67810, #80389, .T. ) ;
#64102=FACE_OUTER_BOUND ( 'NONE', #34151, .T. ) ;
#64110=ADVANCED_FACE ( 'NONE', ( #39587 ), #15861, .F. ) ;
#64111=CARTESIAN_POINT ( 'NONE',  ( 2.554262525012303442, 1.554943921348592717, 0.4744094488188975722 ) ) ;
#64142=DIRECTION ( 'NONE',  ( 1.049727191138616477E-16, -0.5150380749100564870, 0.8571673007021107793 ) ) ;
#64170=ORIENTED_EDGE ( 'NONE', *, *, #14676, .T. ) ;
#64178=CARTESIAN_POINT ( 'NONE',  ( -0.1340670299283584221, 1.082026165109803317, 2.856419976764481117 ) ) ;
#64179=DIRECTION ( 'NONE',  ( 0.000000000000000000, 0.000000000000000000, -1.000000000000000000 ) ) ;
#64186=VERTEX_POINT ( 'NONE', #27795 ) ;
#64195=ORIENTED_EDGE ( 'NONE', *, *, #22408, .F. ) ;
#64217=DIRECTION ( 'NONE',  ( 0.000000000000000000, 0.000000000000000000, -1.000000000000000000 ) ) ;
#64235=CARTESIAN_POINT ( 'NONE',  ( 1.024278008493452630, 1.664615899758172368, 0.4581426849250264111 ) ) ;
#64246=AXIS2_PLACEMENT_3D ( 'NONE', #13503, #34111, #26545 ) ;
#64262=VERTEX_POINT ( 'NONE', #42886 ) ;
#64264=ORIENTED_EDGE ( 'NONE', *, *, #23392, .T. ) ;
#64287=CARTESIAN_POINT ( 'NONE',  ( 1.895263394252414857, 1.111778211650222170, 0.2101609992702619945 ) ) ;
#64300=CARTESIAN_POINT ( 'NONE',  ( -0.06112347087428735004, 1.066921639274551081, -1.448920818111165021 ) ) ;
#64310=DIRECTION ( 'NONE',  ( -0.000000000000000000, -1.000000000000000000, -0.000000000000000000 ) ) ;
#64318=CARTESIAN_POINT ( 'NONE',  ( 3.821484228344193657, 2.755905511811024056, -0.5314960629921260393 ) ) ;
#64334=CARTESIAN_POINT ( 'NONE',  ( -1.559171609364246924, 0.3937007874015748254, 0.5949441279213820710 ) ) ;
#64340=ADVANCED_FACE ( 'NONE', ( #74496 ), #81223, .F. ) ;
#64364=ORIENTED_EDGE ( 'NONE', *, *, #68219, .T. ) ;
#64366=ORIENTED_EDGE ( 'NONE', *, *, #4386, .F. ) ;
#64406=EDGE_CURVE ( 'NONE', #57884, #65284, #9275, .T. ) ;
#64423=B_SPLINE_CURVE_WITH_KNOTS ( 'NONE', 3,
 ( #28459, #66358, #79834, #54955 ),
 .UNSPECIFIED., .F., .F.,
 ( 4, 4 ),
 ( 2.888536477665436318E-07, 0.001436607511248042500 ),
 .UNSPECIFIED. ) ;
#64425=CARTESIAN_POINT ( 'NONE',  ( -3.937007874015748143, 1.724409448818897905, 0.4359958488159719758 ) ) ;
#64463=CARTESIAN_POINT ( 'NONE',  ( -0.4698620426709900766, 1.469755830210692560, -2.159222551273901836 ) ) ;
#64467=ORIENTED_EDGE ( 'NONE', *, *, #41459, .T. ) ;
#64483=ORIENTED_EDGE ( 'NONE', *, *, #52190, .F. ) ;
#64484=ADVANCED_FACE ( 'NONE', ( #21892 ), #29852, .T. ) ;
#64495=CARTESIAN_POINT ( 'NONE',  ( -1.559171609364246924, 0.3937007874015748254, 0.1028181436694137613 ) ) ;
#64511=CARTESIAN_POINT ( 'NONE',  ( -0.3812543623607988486, 1.253662731238188721, 2.019864340580467932 ) ) ;
#64589=DIRECTION ( 'NONE',  ( 0.000000000000000000, 0.000000000000000000, 1.000000000000000000 ) ) ;
#64597=VERTEX_POINT ( 'NONE', #16426 ) ;
#64598=AXIS2_PLACEMENT_3D ( 'NONE', #54440, #7029, #7454 ) ;
#64599=CARTESIAN_POINT ( 'NONE',  ( -1.120392597725979655, 1.066916830561088103, -0.06289000371407697798 ) ) ;
#64616=AXIS2_PLACEMENT_3D ( 'NONE', #16440, #66534, #8865 ) ;
#64625=ADVANCED_FACE ( 'NONE', ( #10521, #67767 ), #10103, .T. ) ;
#64633=ADVANCED_FACE ( 'NONE', ( #4189 ), #55515, .F. ) ;
#64663=EDGE_LOOP ( 'NONE', ( #36006, #31541, #78247, #52221, #37858, #76298, #33438 ) ) ;
#64669=CARTESIAN_POINT ( 'NONE',  ( 0.5314960629921393620, 2.755905511811024056, -3.821484228344191880 ) ) ;
#64680=DIRECTION ( 'NONE',  ( -1.000000000000000000, -0.000000000000000000, -0.000000000000000000 ) ) ;
#64690=LINE ( 'NONE', #78591, #78072 ) ;
#64696=VERTEX_POINT ( 'NONE', #18879 ) ;
#64697=VERTEX_POINT ( 'NONE', #75730 ) ;
#64704=CARTESIAN_POINT ( 'NONE',  ( -0.4682703957577433740, 1.459763210197655647, 3.909061675276500392 ) ) ;
#64717=CARTESIAN_POINT ( 'NONE',  ( -0.05584411899101405369, 1.066260977814800670, -1.627668078129365314 ) ) ;
#64730=EDGE_CURVE ( 'NONE', #9834, #82476, #3761, .T. ) ;
#64738=FACE_OUTER_BOUND ( 'NONE', #8379, .T. ) ;
#64746=DIRECTION ( 'NONE',  ( 0.000000000000000000, 1.000000000000000000, 0.000000000000000000 ) ) ;
#64753=DIRECTION ( 'NONE',  ( -0.000000000000000000, -1.000000000000000000, -0.000000000000000000 ) ) ;
#64761=CARTESIAN_POINT ( 'NONE',  ( 0.03098326503090165565, 1.062992125984251635, -3.937007874015749920 ) ) ;
#64814=DIRECTION ( 'NONE',  ( -0.000000000000000000, -1.000000000000000000, -0.000000000000000000 ) ) ;
#64817=DIRECTION ( 'NONE',  ( -1.000000000000000000, -0.000000000000000000, -0.000000000000000000 ) ) ;
#64821=B_SPLINE_CURVE_WITH_KNOTS ( 'NONE', 3,
 ( #6988, #72229, #33082, #65074, #685, #57900, #77707, #14158, #53259, #44843, #70540, #39814 ),
 .UNSPECIFIED., .F., .F.,
 ( 4, 2, 2, 2, 2, 4 ),
 ( 0.007992874908874613230, 0.009303755029336854485, 0.01061463514979909574, 0.01192551527026133873, 0.01258095533049245415, 0.01323639539072356958 ),
 .UNSPECIFIED. ) ;
#64857=CARTESIAN_POINT ( 'NONE',  ( -1.881759086957760285, 2.742776672516394232, 0.5314960629921260393 ) ) ;
#64858=CARTESIAN_POINT ( 'NONE',  ( 0.000000000000000000, 0.000000000000000000, 0.000000000000000000 ) ) ;
#64866=VERTEX_POINT ( 'NONE', #5426 ) ;
#64873=FACE_OUTER_BOUND ( 'NONE', #76489, .T. ) ;
#64875=DIRECTION ( 'NONE',  ( -0.000000000000000000, -1.000000000000000000, -0.000000000000000000 ) ) ;
#64881=FACE_OUTER_BOUND ( 'NONE', #59362, .T. ) ;
#64894=ADVANCED_FACE ( 'NONE', ( #5830 ), #31981, .F. ) ;
#64903=CARTESIAN_POINT ( 'NONE',  ( -0.5314960629921393620, 2.755905511811024056, 3.826707563893390951 ) ) ;
#64905=CARTESIAN_POINT ( 'NONE',  ( 3.908320185825791881, 1.537401574803149984, -0.4744094488188970171 ) ) ;
#64914=LINE ( 'NONE', #13163, #63204 ) ;
#64932=DIRECTION ( 'NONE',  ( -1.000000000000000000, 0.000000000000000000, -3.491481338843132961E-15 ) ) ;
#64961=EDGE_CURVE ( 'NONE', #51378, #55951, #48706, .T. ) ;
#64973=CARTESIAN_POINT ( 'NONE',  ( -1.519422763189357539, 0.2755905511811023723, 0.7302211324797359682 ) ) ;
#64982=EDGE_CURVE ( 'NONE', #50071, #72444, #2027, .T. ) ;
#64985=CARTESIAN_POINT ( 'NONE',  ( 0.3855990896080964681, 1.260602825228276602, 1.053749523914724318 ) ) ;
#64996=VECTOR ( 'NONE', #32325, 39.37007874015748143 ) ;
#65004=ORIENTED_EDGE ( 'NONE', *, *, #18159, .T. ) ;
#65009=DIRECTION ( 'NONE',  ( -0.000000000000000000, -1.000000000000000000, -0.000000000000000000 ) ) ;
#65019=CARTESIAN_POINT ( 'NONE',  ( -3.937007874015748143, 2.165354330708661568, 0.3149606299212595606 ) ) ;
#65026=ORIENTED_EDGE ( 'NONE', *, *, #43993, .T. ) ;
#65027=CARTESIAN_POINT ( 'NONE',  ( -1.854472803289052507, 2.716535433070866645, -0.5314960629921260393 ) ) ;
#65042=EDGE_CURVE ( 'NONE', #29487, #80970, #32755, .T. ) ;
#65055=AXIS2_PLACEMENT_3D ( 'NONE', #61271, #72668, #73084 ) ;
#65059=ORIENTED_EDGE ( 'NONE', *, *, #61531, .T. ) ;
#65074=CARTESIAN_POINT ( 'NONE',  ( 0.4562095852119599781, 1.668416680336031188, 2.594411373832410828 ) ) ;
#65093=DIRECTION ( 'NONE',  ( 0.000000000000000000, -1.000000000000000000, 0.000000000000000000 ) ) ;
#65105=EDGE_LOOP ( 'NONE', ( #12298, #25204, #62294, #27539 ) ) ;
#65117=FACE_OUTER_BOUND ( 'NONE', #75120, .T. ) ;
#65122=ADVANCED_FACE ( 'NONE', ( #59259 ), #13830, .F. ) ;
#65125=ORIENTED_EDGE ( 'NONE', *, *, #78984, .T. ) ;
#65167=CARTESIAN_POINT ( 'NONE',  ( -2.583694225513480713, 2.755905511811024056, -0.5314960629921260393 ) ) ;
#65176=CARTESIAN_POINT ( 'NONE',  ( 1.348312163386739426, 0.2755905511811023723, 0.8577811012195456497 ) ) ;
#65182=VERTEX_POINT ( 'NONE', #65176 ) ;
#65192=CARTESIAN_POINT ( 'NONE',  ( 0.4116952507455398091, 1.299637793558053644, -3.915461318743572505 ) ) ;
#65196=VERTEX_POINT ( 'NONE', #79067 ) ;
#65197=CIRCLE ( 'NONE', #28904, 1.889763779527559251 ) ;
#65211=VERTEX_POINT ( 'NONE', #39913 ) ;
#65213=ORIENTED_EDGE ( 'NONE', *, *, #35790, .T. ) ;
#65216=CARTESIAN_POINT ( 'NONE',  ( 2.872985923768004213, 1.064103292658513666, 0.03357545743407176764 ) ) ;
#65223=DIRECTION ( 'NONE',  ( -3.491481338843132961E-15, -0.000000000000000000, 1.000000000000000000 ) ) ;
#65231=B_SPLINE_CURVE_WITH_KNOTS ( 'NONE', 3,
 ( #78183, #12951, #12531, #19247, #321, #71862, #14212, #27233, #31882, #25975, #39020, #51221, #39870, #65559, #38609, #52892, #38192, #25554, #52056, #57542, #83233, #20094, #64287, #51633, #77337, #8302, #65966, #1987, #53724, #48247, #21344, #41114, #3645, #8716, #66803, #2408, #21750, #47829, #9138, #34809, #22170, #9958, #72690, #73532, #46997, #33970, #73104, #59631, #41932, #15038, #60468, #27650, #79431, #46584, #14629, #72283, #22586, #40693, #80680, #67627 ),
 .UNSPECIFIED., .F., .F.,
 ( 4, 2, 2, 2, 2, 2, 2, 2, 2, 2, 2, 2, 2, 2, 2, 2, 2, 2, 2, 2, 2, 2, 2, 2, 2, 2, 2, 2, 2, 4 ),
 ( 0.01323639539072356784, 0.01388181161316722097, 0.01452722783561087409, 0.01581806028049817514, 0.01710889272538547792, 0.01839972517027278071, 0.02098139006004740015, 0.02356305494982201612, 0.02485388739470933625, 0.02614471983959665291, 0.02743555228448397304, 0.02872638472937128623, 0.03130804961914591955, 0.03259888206403323274, 0.03388971450892054593, 0.03453513073136420253, 0.03518054695380785912, 0.03647137939869517925, 0.03776221184358249244, 0.03905304428846980563, 0.04034387673335712576, 0.04163470917824443895, 0.04421637406801907921, 0.04679803895779371253, 0.04937970384756834585, 0.05067053629245565904, 0.05196136873734297223, 0.05325220118223029236, 0.05389761740467396284, 0.05454303362711762637 ),
 .UNSPECIFIED. ) ;
#65258=AXIS2_PLACEMENT_3D ( 'NONE', #26904, #78272, #20603 ) ;
#65259=CYLINDRICAL_SURFACE ( 'NONE', #8602, 0.4744094488188972947 ) ;
#65276=LINE ( 'NONE', #79163, #11818 ) ;
#65281=CARTESIAN_POINT ( 'NONE',  ( -0.03443470937339728616, 0.000000000000000000, -1.537015892239756099 ) ) ;
#65284=VERTEX_POINT ( 'NONE', #76743 ) ;
#65295=DIRECTION ( 'NONE',  ( 0.000000000000000000, 1.000000000000000000, -0.000000000000000000 ) ) ;
#65297=B_SPLINE_CURVE_WITH_KNOTS ( 'NONE', 3,
 ( #13935, #76646, #25698, #7620 ),
 .UNSPECIFIED., .F., .F.,
 ( 4, 4 ),
 ( 0.05218731980467056220, 0.05362944292333609447 ),
 .UNSPECIFIED. ) ;
#65303=ORIENTED_EDGE ( 'NONE', *, *, #79432, .T. ) ;
#65309=CARTESIAN_POINT ( 'NONE',  ( -1.559171609364246924, 1.299212598425196985, 0.4177787735906735578 ) ) ;
#65315=CARTESIAN_POINT ( 'NONE',  ( 0.000000000000000000, 2.755905511811024056, 0.000000000000000000 ) ) ;
#65316=ADVANCED_FACE ( 'NONE', ( #77585 ), #57361, .T. ) ;
#65319=ORIENTED_EDGE ( 'NONE', *, *, #46418, .F. ) ;
#65340=ORIENTED_EDGE ( 'NONE', *, *, #22702, .F. ) ;
#65350=FACE_OUTER_BOUND ( 'NONE', #3304, .T. ) ;
#65364=AXIS2_PLACEMENT_3D ( 'NONE', #71050, #59242, #21369 ) ;
#65365=AXIS2_PLACEMENT_3D ( 'NONE', #43070, #51031, #62444 ) ;
#65367=DIRECTION ( 'NONE',  ( 0.000000000000000000, 0.000000000000000000, 1.000000000000000000 ) ) ;
#65368=CYLINDRICAL_SURFACE ( 'NONE', #44613, 0.09842519685039351207 ) ;
#65377=CARTESIAN_POINT ( 'NONE',  ( 1.016821367227983774, 1.537401574803149984, -0.4744094488188970171 ) ) ;
#65380=CARTESIAN_POINT ( 'NONE',  ( 0.1229937836670168122, 1.078949693266341603, 3.935114318630247077 ) ) ;
#65414=CARTESIAN_POINT ( 'NONE',  ( 0.4437891188668303677, 1.369016496689889895, 1.030574033111541166 ) ) ;
#65425=APPLICATION_CONTEXT ( 'automotive_design' ) ;
#65436=ORIENTED_EDGE ( 'NONE', *, *, #58210, .T. ) ;
#65446=DIRECTION ( 'NONE',  ( 0.000000000000000000, 0.000000000000000000, -1.000000000000000000 ) ) ;
#65450=EDGE_CURVE ( 'NONE', #39649, #48388, #19637, .T. ) ;
#65458=VERTEX_POINT ( 'NONE', #45984 ) ;
#65476=VECTOR ( 'NONE', #2694, 39.37007874015748143 ) ;
#65514=DIRECTION ( 'NONE',  ( -0.000000000000000000, 1.000000000000000000, -0.000000000000000000 ) ) ;
#65517=ORIENTED_EDGE ( 'NONE', *, *, #54718, .T. ) ;
#65518=ORIENTED_EDGE ( 'NONE', *, *, #80096, .T. ) ;
#65534=AXIS2_PLACEMENT_3D ( 'NONE', #53747, #79457, #81007 ) ;
#65535=VERTEX_POINT ( 'NONE', #47236 ) ;
#65537=CIRCLE ( 'NONE', #46708, 1.122047244094488194 ) ;
#65553=ORIENTED_EDGE ( 'NONE', *, *, #72539, .T. ) ;
#65559=CARTESIAN_POINT ( 'NONE',  ( 2.020039340939663752, 1.253873987468406392, 0.3814095263789863965 ) ) ;
#65567=DIRECTION ( 'NONE',  ( 0.000000000000000000, 0.000000000000000000, 1.000000000000000000 ) ) ;
#65572=CARTESIAN_POINT ( 'NONE',  ( 2.362204724409448620, 1.724409448818900570, 8.247593713802677664E-15 ) ) ;
#65582=ADVANCED_FACE ( 'NONE', ( #26644 ), #946, .F. ) ;
#65585=FACE_OUTER_BOUND ( 'NONE', #80616, .T. ) ;
#65601=CARTESIAN_POINT ( 'NONE',  ( -3.908320185825792326, 1.521933560353155857, -0.4744094488188975722 ) ) ;
#65610=CARTESIAN_POINT ( 'NONE',  ( 1.141392835773559211, 1.299212598425196985, 1.141392835773562764 ) ) ;
#65618=CARTESIAN_POINT ( 'NONE',  ( -3.911372956956467029, 1.694725607269298218, 0.4487278785265438885 ) ) ;
#65634=EDGE_CURVE ( 'NONE', #80735, #21338, #76216, .T. ) ;
#65638=ORIENTED_EDGE ( 'NONE', *, *, #34659, .F. ) ;
#65640=ORIENTED_EDGE ( 'NONE', *, *, #69856, .F. ) ;
#65643=CARTESIAN_POINT ( 'NONE',  ( 2.829418903715935407, 1.111478976311908617, 0.2095522481616418631 ) ) ;
#65662=EDGE_CURVE ( 'NONE', #58992, #64597, #47874, .T. ) ;
#65708=DIRECTION ( 'NONE',  ( 0.000000000000000000, 0.000000000000000000, -1.000000000000000000 ) ) ;
#65715=CYLINDRICAL_SURFACE ( 'NONE', #71351, 0.4744094488188972947 ) ;
#65731=CARTESIAN_POINT ( 'NONE',  ( 0.01715078996012292523, 1.063284142118728903, -1.620408976207265761 ) ) ;
#65740=EDGE_LOOP ( 'NONE', ( #31659, #21302, #26287, #41909 ) ) ;
#65755=CARTESIAN_POINT ( 'NONE',  ( -0.5314960629921393620, 2.751923335154144556, 3.846978723397334488 ) ) ;
#65757=CARTESIAN_POINT ( 'NONE',  ( 3.927301751045197964, 1.151648106155687801, -0.2765835404858998925 ) ) ;
#65768=CARTESIAN_POINT ( 'NONE',  ( -0.03443470937339728616, 1.062992125984252079, -1.537015892239756099 ) ) ;
#65792=CYLINDRICAL_SURFACE ( 'NONE', #50436, 0.4744094488188972947 ) ;
#65795=CARTESIAN_POINT ( 'NONE',  ( 0.06179341360373440117, 1.065997766574747319, 3.936642186895995987 ) ) ;
#65802=CARTESIAN_POINT ( 'NONE',  ( -3.224202737261815166, 2.716535433070866645, 0.5314960629921260393 ) ) ;
#65828=CARTESIAN_POINT ( 'NONE',  ( -0.4418045515502812548, 1.710866862483978013, -2.103588674771180500 ) ) ;
#65847=ORIENTED_EDGE ( 'NONE', *, *, #81602, .F. ) ;
#65851=CARTESIAN_POINT ( 'NONE',  ( -0.4725553370316754043, 1.494684982616656832, 2.558793778315643586 ) ) ;
#65855=DIRECTION ( 'NONE',  ( 0.000000000000000000, 1.000000000000000000, -0.000000000000000000 ) ) ;
#65860=DIRECTION ( 'NONE',  ( 0.000000000000000000, 8.326672684688674053E-16, 1.000000000000000000 ) ) ;
#65884=EDGE_CURVE ( 'NONE', #41808, #6386, #63000, .T. ) ;
#65899=ORIENTED_EDGE ( 'NONE', *, *, #4970, .F. ) ;
#65914=CARTESIAN_POINT ( 'NONE',  ( 0.3162942679073420527, 1.183613643627707157, -1.704860272166652146 ) ) ;
#65925=ORIENTED_EDGE ( 'NONE', *, *, #31058, .F. ) ;
#65935=AXIS2_PLACEMENT_3D ( 'NONE', #9052, #48166, #73444 ) ;
#65941=VERTEX_POINT ( 'NONE', #44436 ) ;
#65943=EDGE_LOOP ( 'NONE', ( #23477, #14604, #697, #79312 ) ) ;
#65966=CARTESIAN_POINT ( 'NONE',  ( 1.854728618660368422, 1.067671560069314296, 0.06860298820095168948 ) ) ;
#65989=CARTESIAN_POINT ( 'NONE',  ( 0.4497368882408442348, 1.386401378945496532, -1.551431943024248472 ) ) ;
#65991=DIRECTION ( 'NONE',  ( 0.000000000000000000, -1.000000000000000000, 0.000000000000000000 ) ) ;
#66013=CARTESIAN_POINT ( 'NONE',  ( 0.4744094488189065095, 1.537401574803149984, -2.554262525012259477 ) ) ;
#66014=EDGE_CURVE ( 'NONE', #26718, #40163, #44847, .T. ) ;
#66025=ORIENTED_EDGE ( 'NONE', *, *, #36840, .F. ) ;
#66027=ORIENTED_EDGE ( 'NONE', *, *, #35630, .T. ) ;
#66043=ORIENTED_EDGE ( 'NONE', *, *, #83060, .F. ) ;
#66046=DIRECTION ( 'NONE',  ( -0.000000000000000000, -1.000000000000000000, 0.000000000000000000 ) ) ;
#66080=LINE ( 'NONE', #54256, #48033 ) ;
#66086=CARTESIAN_POINT ( 'NONE',  ( 0.5314960629920849611, 2.682389230697235671, 3.900966923095593675 ) ) ;
#66088=EDGE_CURVE ( 'NONE', #21419, #20068, #62169, .T. ) ;
#66096=EDGE_CURVE ( 'NONE', #9504, #76416, #75642, .T. ) ;
#66105=DIRECTION ( 'NONE',  ( 0.000000000000000000, -1.000000000000000000, 0.000000000000000000 ) ) ;
#66116=DIRECTION ( 'NONE',  ( 0.000000000000000000, -0.000000000000000000, 1.000000000000000000 ) ) ;
#66118=DIRECTION ( 'NONE',  ( -0.000000000000000000, -1.000000000000000000, -0.000000000000000000 ) ) ;
#66126=VERTEX_POINT ( 'NONE', #17981 ) ;
#66135=CARTESIAN_POINT ( 'NONE',  ( 0.02109673867167633637, 1.063447502424408775, -1.617503877632567422 ) ) ;
#66141=LINE ( 'NONE', #8479, #64070 ) ;
#66144=CARTESIAN_POINT ( 'NONE',  ( -0.4672625608940637609, 1.453874696264121802, -2.153215735734194336 ) ) ;
#66148=ORIENTED_EDGE ( 'NONE', *, *, #733, .T. ) ;
#66168=DIRECTION ( 'NONE',  ( -0.000000000000000000, -1.000000000000000000, -0.000000000000000000 ) ) ;
#66191=CARTESIAN_POINT ( 'NONE',  ( -0.4563452811745912219, 0.01305114060239447211, -2.130073781772667374 ) ) ;
#66204=CARTESIAN_POINT ( 'NONE',  ( 0.03098196894106152940, 1.062992125984253411, 3.937007874015747699 ) ) ;
#66226=ORIENTED_EDGE ( 'NONE', *, *, #8016, .F. ) ;
#66237=CARTESIAN_POINT ( 'NONE',  ( 0.1088160626412674192, 1.075376824458859959, 1.116863795850121521 ) ) ;
#66259=CARTESIAN_POINT ( 'NONE',  ( 3.250800428249174256, 2.742781089625998980, -0.5314960629921260393 ) ) ;
#66260=PLANE ( 'NONE',  #58443 ) ;
#66265=CIRCLE ( 'NONE', #29955, 0.1771653543307085410 ) ;
#66268=ORIENTED_EDGE ( 'NONE', *, *, #66096, .T. ) ;
#66270=CARTESIAN_POINT ( 'NONE',  ( -1.102273020300588602, 1.111722227514729155, -0.2117565784830439668 ) ) ;
#66284=AXIS2_PLACEMENT_3D ( 'NONE', #22317, #28211, #66528 ) ;
#66295=DIRECTION ( 'NONE',  ( 0.000000000000000000, -0.000000000000000000, -1.000000000000000000 ) ) ;
#66338=VERTEX_POINT ( 'NONE', #41156 ) ;
#66345=CARTESIAN_POINT ( 'NONE',  ( -0.5314960629921122726, 2.559055118110236560, -3.937007874015763687 ) ) ;
#66358=CARTESIAN_POINT ( 'NONE',  ( -2.130073781772662489, 0.01305114060239441834, -0.4563452811746135374 ) ) ;
#66364=FACE_OUTER_BOUND ( 'NONE', #278, .T. ) ;
#66365=LINE ( 'NONE', #4042, #43131 ) ;
#66367=EDGE_CURVE ( 'NONE', #28871, #10316, #52727, .T. ) ;
#66374=VERTEX_POINT ( 'NONE', #66844 ) ;
#66402=CARTESIAN_POINT ( 'NONE',  ( 0.4177787735906991484, 1.312623414240987163, -1.404325600637324367 ) ) ;
#66411=LINE ( 'NONE', #34419, #21986 ) ;
#66426=FACE_BOUND ( 'NONE', #79170, .T. ) ;
#66439=VERTEX_POINT ( 'NONE', #1618 ) ;
#66456=ORIENTED_EDGE ( 'NONE', *, *, #60880, .F. ) ;
#66459=CARTESIAN_POINT ( 'NONE',  ( -1.485206097856770269, 1.138394384027662243, 0.2566527756886388123 ) ) ;
#66471=ORIENTED_EDGE ( 'NONE', *, *, #68170, .T. ) ;
#66494=DIRECTION ( 'NONE',  ( 0.000000000000000000, 1.000000000000000000, -0.000000000000000000 ) ) ;
#66500=CARTESIAN_POINT ( 'NONE',  ( -0.5314960629921127166, 2.755905511811024056, -3.831929248781930308 ) ) ;
#66525=VECTOR ( 'NONE', #23803, 39.37007874015748143 ) ;
#66528=DIRECTION ( 'NONE',  ( 0.000000000000000000, 1.387778780781445676E-15, -1.000000000000000000 ) ) ;
#66529=ORIENTED_EDGE ( 'NONE', *, *, #22849, .F. ) ;
#66534=DIRECTION ( 'NONE',  ( 0.000000000000000000, 1.000000000000000000, 0.000000000000000000 ) ) ;
#66542=EDGE_LOOP ( 'NONE', ( #61170, #26571, #32286, #14970 ) ) ;
#66551=DIRECTION ( 'NONE',  ( 0.000000000000000000, -1.000000000000000000, 0.000000000000000000 ) ) ;
#66560=VERTEX_POINT ( 'NONE', #46629 ) ;
#66580=DIRECTION ( 'NONE',  ( -0.000000000000000000, 1.000000000000000000, -0.000000000000000000 ) ) ;
#66584=CARTESIAN_POINT ( 'NONE',  ( -0.4563452811745912219, 0.01305114060239447385, 2.130073781772667374 ) ) ;
#66591=DIRECTION ( 'NONE',  ( 1.408710688920637755E-15, -1.000000000000000000, 4.918487082195260922E-30 ) ) ;
#66595=EDGE_CURVE ( 'NONE', #57500, #75161, #78226, .T. ) ;
#66599=CARTESIAN_POINT ( 'NONE',  ( -0.01569160312983191446, 1.062992125984252967, -1.122047244094488194 ) ) ;
#66606=CARTESIAN_POINT ( 'NONE',  ( 0.000000000000000000, 2.559055118110236560, 0.000000000000000000 ) ) ;
#66656=CARTESIAN_POINT ( 'NONE',  ( 0.000000000000000000, 1.062992125984252745, 1.122047244094488194 ) ) ;
#66675=VERTEX_POINT ( 'NONE', #7515 ) ;
#66677=ORIENTED_EDGE ( 'NONE', *, *, #68728, .T. ) ;
#66681=AXIS2_PLACEMENT_3D ( 'NONE', #56120, #25368, #30864 ) ;
#66682=CARTESIAN_POINT ( 'NONE',  ( 0.000000000000000000, 2.755905511811024056, 0.000000000000000000 ) ) ;
#66694=LINE ( 'NONE', #28790, #33094 ) ;
#66700=AXIS2_PLACEMENT_3D ( 'NONE', #38076, #37664, #13670 ) ;
#66702=DIRECTION ( 'NONE',  ( -0.000000000000000000, -1.000000000000000000, -0.000000000000000000 ) ) ;
#66709=CARTESIAN_POINT ( 'NONE',  ( -2.362204724409448620, 0.03937007874015751446, -2.474278114140802984E-14 ) ) ;
#66737=VECTOR ( 'NONE', #20414, 39.37007874015748854 ) ;
#66741=VECTOR ( 'NONE', #22201, 39.37007874015748143 ) ;
#66742=VECTOR ( 'NONE', #70552, 39.37007874015748143 ) ;
#66761=CARTESIAN_POINT ( 'NONE',  ( 0.000000000000000000, 0.03937007874015751446, -2.362204724409448620 ) ) ;
#66762=VECTOR ( 'NONE', #7892, 39.37007874015748143 ) ;
#66764=ORIENTED_EDGE ( 'NONE', *, *, #64982, .T. ) ;
#66800=FACE_OUTER_BOUND ( 'NONE', #18723, .T. ) ;
#66803=CARTESIAN_POINT ( 'NONE',  ( 1.857147851633400792, 1.070284760220071352, -0.08454815954499718400 ) ) ;
#66805=VECTOR ( 'NONE', #16186, 39.37007874015748143 ) ;
#66812=FACE_OUTER_BOUND ( 'NONE', #30285, .T. ) ;
#66829=CYLINDRICAL_SURFACE ( 'NONE', #29051, 0.4744094488188972947 ) ;
#66844=CARTESIAN_POINT ( 'NONE',  ( 3.924389226575468737, 2.165354330708661568, -0.3149606299212595606 ) ) ;
#66848=CARTESIAN_POINT ( 'NONE',  ( 0.4359958488159816348, 1.724409448818897905, -2.630268417803909298 ) ) ;
#66851=AXIS2_PLACEMENT_3D ( 'NONE', #15722, #16130, #48094 ) ;
#66858=CONICAL_SURFACE ( 'NONE', #58781, 2.165354330708661568, 0.7853981633974500554 ) ;
#66861=CARTESIAN_POINT ( 'NONE',  ( 3.861135848600278475, 2.745602313593968447, 0.5314960629921260393 ) ) ;
#66865=ORIENTED_EDGE ( 'NONE', *, *, #14300, .T. ) ;
#66881=EDGE_LOOP ( 'NONE', ( #76351, #53289 ) ) ;
#66884=CARTESIAN_POINT ( 'NONE',  ( -1.559171609364246924, 1.128537896298103416, 0.2406134192599649890 ) ) ;
#66890=CARTESIAN_POINT ( 'NONE',  ( 0.4422863986689484772, 1.709743469447152719, 1.031222268885702231 ) ) ;
#66897=DIRECTION ( 'NONE',  ( -3.491481338843133355E-15, -0.000000000000000000, 1.000000000000000000 ) ) ;
#66922=CIRCLE ( 'NONE', #57498, 0.09842519685039351207 ) ;
#66936=EDGE_CURVE ( 'NONE', #30111, #48126, #11867, .T. ) ;
#66955=DIRECTION ( 'NONE',  ( 0.000000000000000000, 0.000000000000000000, 1.000000000000000000 ) ) ;
#66962=ORIENTED_EDGE ( 'NONE', *, *, #61781, .T. ) ;
#66965=VERTEX_POINT ( 'NONE', #18586 ) ;
#66971=CARTESIAN_POINT ( 'NONE',  ( 0.02826831778055379635, 1.063821329225880019, -1.462794063659299093 ) ) ;
#66979=ORIENTED_EDGE ( 'NONE', *, *, #73302, .T. ) ;
#66983=VECTOR ( 'NONE', #24865, 39.37007874015748143 ) ;
#67016=CARTESIAN_POINT ( 'NONE',  ( -0.4744094488188934089, 1.521776870516600821, -1.016821367227985551 ) ) ;
#67046=CARTESIAN_POINT ( 'NONE',  ( -1.559171609364246924, 1.128537896298103416, 0.2406134192599649890 ) ) ;
#67084=CARTESIAN_POINT ( 'NONE',  ( -0.4744094488188880798, 1.537401574803149984, -2.554262525012305218 ) ) ;
#67086=DIRECTION ( 'NONE',  ( 1.000000000000000000, 1.387778780781445676E-15, 0.000000000000000000 ) ) ;
#67089=ORIENTED_EDGE ( 'NONE', *, *, #51971, .F. ) ;
#67090=ADVANCED_FACE ( 'NONE', ( #37520 ), #34753, .F. ) ;
#67094=CARTESIAN_POINT ( 'NONE',  ( 0.4744094488188900782, 1.537401574803149984, 2.170146923806596906 ) ) ;
#67097=CARTESIAN_POINT ( 'NONE',  ( -0.4712114270530097793, 1.601157653251831903, 3.908712503217392609 ) ) ;
#67112=CARTESIAN_POINT ( 'NONE',  ( -3.908417273630399258, 1.569223574151384470, -0.4736117085908965185 ) ) ;
#67119=CARTESIAN_POINT ( 'NONE',  ( 2.558921551581142317, 1.580736828574225150, -0.4725026149319433433 ) ) ;
#67131=AXIS2_PLACEMENT_3D ( 'NONE', #39220, #77963, #33345 ) ;
#67140=LINE ( 'NONE', #22922, #24607 ) ;
#67169=EDGE_CURVE ( 'NONE', #53039, #62716, #22440, .T. ) ;
#67175=EDGE_LOOP ( 'NONE', ( #6503, #51696, #45622, #14690 ) ) ;
#67176=ORIENTED_EDGE ( 'NONE', *, *, #41242, .T. ) ;
#67193=ORIENTED_EDGE ( 'NONE', *, *, #52442, .F. ) ;
#67194=CARTESIAN_POINT ( 'NONE',  ( -1.518978356207579372, 1.376229525351539973, 0.4462089517855873932 ) ) ;
#67199=CARTESIAN_POINT ( 'NONE',  ( 0.4744094488188940750, 1.537401574803149984, 1.016821367227985329 ) ) ;
#67220=DIRECTION ( 'NONE',  ( 0.000000000000000000, 1.000000000000000000, 0.000000000000000000 ) ) ;
#67221=ADVANCED_FACE ( 'NONE', ( #53043 ), #34541, .T. ) ;
#67239=CARTESIAN_POINT ( 'NONE',  ( -2.583694225513480713, 2.755905511811024056, 0.5314960629921260393 ) ) ;
#67244=CARTESIAN_POINT ( 'NONE',  ( 0.000000000000000000, 0.000000000000000000, 0.000000000000000000 ) ) ;
#67246=B_SPLINE_CURVE_WITH_KNOTS ( 'NONE', 3,
 ( #56994, #50683, #5662, #82691 ),
 .UNSPECIFIED., .F., .F.,
 ( 4, 4 ),
 ( 0.1635406000437870655, 0.1649189557199158829 ),
 .UNSPECIFIED. ) ;
#67258=AXIS2_PLACEMENT_3D ( 'NONE', #27950, #61177, #53609 ) ;
#67271=ORIENTED_EDGE ( 'NONE', *, *, #46853, .F. ) ;
#67286=EDGE_LOOP ( 'NONE', ( #79742, #62101, #48226 ) ) ;
#67291=CARTESIAN_POINT ( 'NONE',  ( 0.000000000000000000, 2.755905511811024056, 0.000000000000000000 ) ) ;
#67305=ORIENTED_EDGE ( 'NONE', *, *, #29099, .T. ) ;
#67320=EDGE_CURVE ( 'NONE', #43965, #76998, #33381, .T. ) ;
#67334=CARTESIAN_POINT ( 'NONE',  ( -2.077216372526510479, 1.325969025732672391, -0.4256800600601859941 ) ) ;
#67363=CARTESIAN_POINT ( 'NONE',  ( 0.3801136020054692310, 1.252211066003288131, -1.385051565532328111 ) ) ;
#67375=ORIENTED_EDGE ( 'NONE', *, *, #78984, .F. ) ;
#67409=EDGE_CURVE ( 'NONE', #82725, #10316, #37210, .T. ) ;
#67416=EDGE_CURVE ( 'NONE', #77721, #19150, #53771, .T. ) ;
#67419=CARTESIAN_POINT ( 'NONE',  ( 2.570293859026651972, 2.742779986175213569, 0.5314960629921260393 ) ) ;
#67426=CARTESIAN_POINT ( 'NONE',  ( -0.3769492730837889494, 1.247705490064275446, -1.056993455451901376 ) ) ;
#67432=CARTESIAN_POINT ( 'NONE',  ( -0.4744094488189005143, 1.537401574803149984, 1.016821367227982220 ) ) ;
#67439=CIRCLE ( 'NONE', #13659, 0.3149606299212598381 ) ;
#67465=VERTEX_POINT ( 'NONE', #25500 ) ;
#67469=EDGE_CURVE ( 'NONE', #72870, #55060, #34725, .T. ) ;
#67494=DIRECTION ( 'NONE',  ( 0.000000000000000000, -1.000000000000000000, 0.000000000000000000 ) ) ;
#67496=AXIS2_PLACEMENT_3D ( 'NONE', #9792, #10631, #80516 ) ;
#67499=ORIENTED_EDGE ( 'NONE', *, *, #23397, .T. ) ;
#67503=CARTESIAN_POINT ( 'NONE',  ( 0.6299212598424784870, 2.165354330708661568, 3.937007874015796105 ) ) ;
#67504=CARTESIAN_POINT ( 'NONE',  ( 0.4744094488189113945, 1.537401574803149984, -3.937007874015760578 ) ) ;
#67506=CARTESIAN_POINT ( 'NONE',  ( -0.4359958488159683676, 1.724409448818897905, -1.033875059083678272 ) ) ;
#67522=DIRECTION ( 'NONE',  ( 1.000000000000000000, -0.000000000000000000, -0.000000000000000000 ) ) ;
#67540=EDGE_CURVE ( 'NONE', #58460, #52853, #8250, .T. ) ;
#67558=ORIENTED_EDGE ( 'NONE', *, *, #51210, .T. ) ;
#67559=EDGE_CURVE ( 'NONE', #38353, #45259, #52417, .T. ) ;
#67573=DIRECTION ( 'NONE',  ( 0.000000000000000000, 0.000000000000000000, -1.000000000000000000 ) ) ;
#67603=ORIENTED_EDGE ( 'NONE', *, *, #40920, .T. ) ;
#67606=CARTESIAN_POINT ( 'NONE',  ( -1.313877454013331780, 1.062992125984252079, 0.6999040823587869831 ) ) ;
#67614=VECTOR ( 'NONE', #25037, 39.37007874015748143 ) ;
#67621=VERTEX_POINT ( 'NONE', #27599 ) ;
#67626=EDGE_CURVE ( 'NONE', #74015, #77721, #64821, .T. ) ;
#67627=CARTESIAN_POINT ( 'NONE',  ( 2.170146923806634653, 1.537401574803149984, -0.4744094488188970171 ) ) ;
#67634=CARTESIAN_POINT ( 'NONE',  ( 3.937007874015748143, 2.559055118110236560, 0.5314960629921260393 ) ) ;
#67656=AXIS2_PLACEMENT_3D ( 'NONE', #4394, #17461, #68788 ) ;
#67664=DIRECTION ( 'NONE',  ( -1.000000000000000000, -0.000000000000000000, -0.000000000000000000 ) ) ;
#67668=AXIS2_PLACEMENT_3D ( 'NONE', #70748, #63597, #13508 ) ;
#67684=ORIENTED_EDGE ( 'NONE', *, *, #79905, .T. ) ;
#67686=ORIENTED_EDGE ( 'NONE', *, *, #19758, .T. ) ;
#67704=DIRECTION ( 'NONE',  ( -0.000000000000000000, -1.000000000000000000, -0.000000000000000000 ) ) ;
#67721=DIRECTION ( 'NONE',  ( 0.000000000000000000, -1.387778780781445676E-15, -1.000000000000000000 ) ) ;
#67725=EDGE_CURVE ( 'NONE', #82476, #5673, #79901, .T. ) ;
#67735=EDGE_CURVE ( 'NONE', #77301, #68995, #6570, .T. ) ;
#67748=CARTESIAN_POINT ( 'NONE',  ( -2.159196716652983739, 1.469708627452553706, -0.4698506773045486029 ) ) ;
#67757=PLANE ( 'NONE',  #68964 ) ;
#67767=FACE_OUTER_BOUND ( 'NONE', #19596, .T. ) ;
#67777=CARTESIAN_POINT ( 'NONE',  ( 0.4744094488188886904, 1.537401574803149984, 2.554262525012303886 ) ) ;
#67783=DIRECTION ( 'NONE',  ( -0.000000000000000000, -1.000000000000000000, -0.000000000000000000 ) ) ;
#67792=ORIENTED_EDGE ( 'NONE', *, *, #81099, .F. ) ;
#67803=DIRECTION ( 'NONE',  ( -0.000000000000000000, -1.000000000000000000, -0.000000000000000000 ) ) ;
#67807=ORIENTED_EDGE ( 'NONE', *, *, #36043, .F. ) ;
#67810=VERTEX_POINT ( 'NONE', #9493 ) ;
#67836=CARTESIAN_POINT ( 'NONE',  ( 0.5314960629921373636, 2.755905511811024056, -3.264097702071371288 ) ) ;
#67853=AXIS2_PLACEMENT_3D ( 'NONE', #36349, #28375, #22066 ) ;
#67876=CARTESIAN_POINT ( 'NONE',  ( -1.724509498540856889, 1.220656357563485228, 0.3534487381068502909 ) ) ;
#67879=CARTESIAN_POINT ( 'NONE',  ( 0.000000000000000000, 2.716535433070866645, 0.000000000000000000 ) ) ;
#67906=CIRCLE ( 'NONE', #22181, 0.2165354330708659791 ) ;
#67919=ORIENTED_EDGE ( 'NONE', *, *, #8676, .F. ) ;
#67925=CARTESIAN_POINT ( 'NONE',  ( -0.03443470937339728616, 0.000000000000000000, -1.537015892239756099 ) ) ;
#67935=PLANE ( 'NONE',  #74793 ) ;
#67947=CARTESIAN_POINT ( 'NONE',  ( 2.554262525012263474, 1.546132656481029155, -0.4744094488188972392 ) ) ;
#67957=AXIS2_PLACEMENT_3D ( 'NONE', #82541, #50120, #70310 ) ;
#67968=CARTESIAN_POINT ( 'NONE',  ( 0.2100141437675508982, 1.111707297776196812, 1.895198704147436741 ) ) ;
#67978=CARTESIAN_POINT ( 'NONE',  ( -2.112655059233905508, 1.697151583350147153, -0.4469586986359067593 ) ) ;
#67999=CIRCLE ( 'NONE', #18366, 3.307086614173228689 ) ;
#68011=EDGE_CURVE ( 'NONE', #30111, #72870, #32607, .T. ) ;
#68017=ORIENTED_EDGE ( 'NONE', *, *, #7858, .T. ) ;
#68019=ORIENTED_EDGE ( 'NONE', *, *, #80061, .T. ) ;
#68024=CARTESIAN_POINT ( 'NONE',  ( -0.4744094488188832504, 1.537401574803149984, -3.937007874015763687 ) ) ;
#68025=FACE_OUTER_BOUND ( 'NONE', #64663, .T. ) ;
#68034=ORIENTED_EDGE ( 'NONE', *, *, #52780, .T. ) ;
#68057=AXIS2_PLACEMENT_3D ( 'NONE', #40185, #22069, #26720 ) ;
#68059=VECTOR ( 'NONE', #80309, 39.37007874015748143 ) ;
#68078=DIRECTION ( 'NONE',  ( -1.000000000000000000, -0.000000000000000000, -0.000000000000000000 ) ) ;
#68096=ORIENTED_EDGE ( 'NONE', *, *, #37207, .T. ) ;
#68098=VERTEX_POINT ( 'NONE', #33817 ) ;
#68112=CIRCLE ( 'NONE', #17057, 0.5118110236220472231 ) ;
#68113=ORIENTED_EDGE ( 'NONE', *, *, #68170, .F. ) ;
#68125=CARTESIAN_POINT ( 'NONE',  ( 0.1406185367545949583, 0.2755905511811023723, -1.409564117849439802 ) ) ;
#68138=DIRECTION ( 'NONE',  ( -1.000000000000000000, -0.000000000000000000, -0.000000000000000000 ) ) ;
#68146=EDGE_CURVE ( 'NONE', #36842, #77755, #74822, .T. ) ;
#68168=CARTESIAN_POINT ( 'NONE',  ( 0.000000000000000000, 1.724409448818897461, 0.000000000000000000 ) ) ;
#68170=EDGE_CURVE ( 'NONE', #78980, #69205, #15302, .T. ) ;
#68179=VECTOR ( 'NONE', #16649, 39.37007874015748143 ) ;
#68188=DIRECTION ( 'NONE',  ( 0.000000000000000000, -1.734723475976808327E-16, -1.000000000000000000 ) ) ;
#68195=DIRECTION ( 'NONE',  ( 0.000000000000000000, 0.000000000000000000, 1.000000000000000000 ) ) ;
#68198=CARTESIAN_POINT ( 'NONE',  ( 0.000000000000000000, 0.000000000000000000, 0.000000000000000000 ) ) ;
#68202=ORIENTED_EDGE ( 'NONE', *, *, #63295, .T. ) ;
#68215=B_SPLINE_CURVE_WITH_KNOTS ( 'NONE', 3,
 ( #67094, #32279, #33542, #1565, #26385, #39856, #47710, #71009, #73408, #78169, #52880, #27219 ),
 .UNSPECIFIED., .F., .F.,
 ( 4, 2, 2, 2, 2, 4 ),
 ( 0.05454303362711801495, 0.05585633982237168255, 0.05651299291999852675, 0.05716964601762537096, 0.05848295221287905937, 0.05979625840813274779 ),
 .UNSPECIFIED. ) ;
#68218=CARTESIAN_POINT ( 'NONE',  ( 0.000000000000000000, 2.755905511811024056, 0.000000000000000000 ) ) ;
#68219=EDGE_CURVE ( 'NONE', #51179, #51564, #73794, .T. ) ;
#68226=ORIENTED_EDGE ( 'NONE', *, *, #64961, .T. ) ;
#68254=CARTESIAN_POINT ( 'NONE',  ( 2.556891438210028067, 2.729656593086051242, 0.5314960629921260393 ) ) ;
#68261=CARTESIAN_POINT ( 'NONE',  ( -2.585397804484597550, 1.422882880004781914, 0.4606469518571247312 ) ) ;
#68264=CARTESIAN_POINT ( 'NONE',  ( 1.443709154632419265E-16, 0.4177165354330708569, 1.178877988035069047 ) ) ;
#68293=CARTESIAN_POINT ( 'NONE',  ( -1.735579908797700410, 1.274882798674454421, 0.3961561098831279382 ) ) ;
#68294=FACE_OUTER_BOUND ( 'NONE', #10543, .T. ) ;
#68296=DIRECTION ( 'NONE',  ( 0.000000000000000000, 0.000000000000000000, -1.000000000000000000 ) ) ;
#68297=CIRCLE ( 'NONE', #19861, 3.307086614173228689 ) ;
#68302=ORIENTED_EDGE ( 'NONE', *, *, #61363, .F. ) ;
#68308=CARTESIAN_POINT ( 'NONE',  ( 0.000000000000000000, 1.062992125984252745, 1.122047244094488194 ) ) ;
#68330=CARTESIAN_POINT ( 'NONE',  ( -0.5314960629921122726, 2.755905511811024056, -3.937007874015763687 ) ) ;
#68338=FACE_OUTER_BOUND ( 'NONE', #13781, .T. ) ;
#68350=PRODUCT_CONTEXT ( 'NONE', #65425, 'mechanical' ) ;
#68355=PLANE ( 'NONE',  #40927 ) ;
#68366=CARTESIAN_POINT ( 'NONE',  ( 0.4177787735907000366, 0.3937007874015748254, -1.559171609364239375 ) ) ;
#68373=CARTESIAN_POINT ( 'NONE',  ( 0.4493346515394942009, 1.385193209801244940, -1.573425852207795961 ) ) ;
#68390=VERTEX_POINT ( 'NONE', #28328 ) ;
#68394=CARTESIAN_POINT ( 'NONE',  ( -2.167227123902250696, 1.572090529166658479, -0.4732185887570802274 ) ) ;
#68418=CARTESIAN_POINT ( 'NONE',  ( 0.000000000000000000, 2.755905511811024056, 0.000000000000000000 ) ) ;
#68428=ORIENTED_EDGE ( 'NONE', *, *, #74844, .T. ) ;
#68430=ORIENTED_EDGE ( 'NONE', *, *, #20213, .T. ) ;
#68431=CARTESIAN_POINT ( 'NONE',  ( 0.000000000000000000, 0.000000000000000000, 3.858267716535433323 ) ) ;
#68449=CARTESIAN_POINT ( 'NONE',  ( 2.094141031014959520, 1.724409448818898127, 0.4359958488159723644 ) ) ;
#68450=ADVANCED_FACE ( 'NONE', ( #73373 ), #79702, .F. ) ;
#68454=CARTESIAN_POINT ( 'NONE',  ( 0.000000000000000000, 2.716535433070866645, 0.000000000000000000 ) ) ;
#68476=CARTESIAN_POINT ( 'NONE',  ( -3.900966923095589678, 2.677165354330708791, 0.5314960629921260393 ) ) ;
#68503=ORIENTED_EDGE ( 'NONE', *, *, #50047, .T. ) ;
#68505=ORIENTED_EDGE ( 'NONE', *, *, #69856, .T. ) ;
#68522=CARTESIAN_POINT ( 'NONE',  ( -1.385122803245538714, 1.251927150221335605, 0.3798795596076748882 ) ) ;
#68534=ORIENTED_EDGE ( 'NONE', *, *, #33608, .T. ) ;
#68543=CARTESIAN_POINT ( 'NONE',  ( -0.2508763215440125705, 1.134457504807420802, 3.929027568737346154 ) ) ;
#68562=CARTESIAN_POINT ( 'NONE',  ( -2.169549780153866347, 1.520054044952883876, 0.4741688556381176700 ) ) ;
#68593=FACE_OUTER_BOUND ( 'NONE', #44236, .T. ) ;
#68594=EDGE_CURVE ( 'NONE', #44792, #19641, #54676, .T. ) ;
#68597=FACE_OUTER_BOUND ( 'NONE', #63023, .T. ) ;
#68601=ORIENTED_EDGE ( 'NONE', *, *, #41459, .F. ) ;
#68604=ORIENTED_EDGE ( 'NONE', *, *, #63199, .T. ) ;
#68653=AXIS2_PLACEMENT_3D ( 'NONE', #55941, #14682, #59270 ) ;
#68654=CARTESIAN_POINT ( 'NONE',  ( 0.4744094488189011805, 1.537401574803149984, -1.016821367227981998 ) ) ;
#68657=CARTESIAN_POINT ( 'NONE',  ( -2.873826567705916712, 1.063196196511239089, -0.01636564761922175773 ) ) ;
#68660=DIRECTION ( 'NONE',  ( 0.000000000000000000, 0.000000000000000000, 1.000000000000000000 ) ) ;
#68661=ADVANCED_FACE ( 'NONE', ( #62805 ), #3907, .F. ) ;
#68670=CARTESIAN_POINT ( 'NONE',  ( 0.03140460581128053097, 1.062992125984252301, -1.122047244094487972 ) ) ;
#68674=CARTESIAN_POINT ( 'NONE',  ( 0.1807872349014829905, 1.098494004316914019, -1.883123530778055610 ) ) ;
#68706=AXIS2_PLACEMENT_3D ( 'NONE', #54774, #23609, #40909 ) ;
#68716=CARTESIAN_POINT ( 'NONE',  ( 6.265965269058076312E-17, 1.062992125984252745, -1.850393700787401619 ) ) ;
#68728=EDGE_CURVE ( 'NONE', #2780, #59692, #11463, .T. ) ;
#68731=CARTESIAN_POINT ( 'NONE',  ( -0.4672528563079629271, 1.453807508635540868, -2.571216978929444785 ) ) ;
#68733=DIRECTION ( 'NONE',  ( -0.000000000000000000, -1.000000000000000000, -0.000000000000000000 ) ) ;
#68736=ORIENTED_EDGE ( 'NONE', *, *, #42480, .T. ) ;
#68737=ORIENTED_EDGE ( 'NONE', *, *, #45798, .F. ) ;
#68740=DIRECTION ( 'NONE',  ( 1.047444401652940007E-14, 0.000000000000000000, -1.000000000000000000 ) ) ;
#68767=CARTESIAN_POINT ( 'NONE',  ( -0.03443470937339727228, 0.2755905511811023723, -1.438590695389362573 ) ) ;
#68775=CARTESIAN_POINT ( 'NONE',  ( 1.096712450468791955, 1.126169283821023770, 0.2385660781250339146 ) ) ;
#68788=DIRECTION ( 'NONE',  ( 0.000000000000000000, 0.000000000000000000, -1.000000000000000000 ) ) ;
#68844=LINE ( 'NONE', #11607, #60639 ) ;
#68853=CARTESIAN_POINT ( 'NONE',  ( 3.937007874015748143, 1.724409448818898127, 0.6299212598425202314 ) ) ;
#68860=CARTESIAN_POINT ( 'NONE',  ( -0.5314960629921146040, 2.755905511811024056, -3.264097702071374840 ) ) ;
#68869=CIRCLE ( 'NONE', #75610, 0.1771653543307085410 ) ;
#68884=ORIENTED_EDGE ( 'NONE', *, *, #55811, .T. ) ;
#68911=ORIENTED_EDGE ( 'NONE', *, *, #13087, .T. ) ;
#68934=CARTESIAN_POINT ( 'NONE',  ( 0.000000000000000000, 1.929133858267716661, -2.362204724409448620 ) ) ;
#68937=CARTESIAN_POINT ( 'NONE',  ( 3.912791665790199769, 1.724409448818897905, 0.4359958488159722534 ) ) ;
#68943=ORIENTED_EDGE ( 'NONE', *, *, #22956, .F. ) ;
#68946=ORIENTED_EDGE ( 'NONE', *, *, #40920, .F. ) ;
#68952=DIRECTION ( 'NONE',  ( -0.000000000000000000, -1.000000000000000000, -0.000000000000000000 ) ) ;
#68964=AXIS2_PLACEMENT_3D ( 'NONE', #22298, #34519, #9265 ) ;
#68977=VECTOR ( 'NONE', #31925, 39.37007874015748143 ) ;
#68981=DIRECTION ( 'NONE',  ( 0.000000000000000000, -1.000000000000000000, 0.000000000000000000 ) ) ;
#68990=CARTESIAN_POINT ( 'NONE',  ( -3.926394065941670508, 1.160970718358689702, 0.2891465379911152822 ) ) ;
#68994=CARTESIAN_POINT ( 'NONE',  ( -3.264097702071373064, 2.755905511811024056, 0.5314960629921260393 ) ) ;
#68995=VERTEX_POINT ( 'NONE', #56470 ) ;
#68999=B_SPLINE_CURVE_WITH_KNOTS ( 'NONE', 3,
 ( #14387, #27824, #73702, #1745, #21510, #16042, #47168, #15209, #41688, #9715, #29064, #54735 ),
 .UNSPECIFIED., .F., .F.,
 ( 4, 2, 2, 2, 2, 4 ),
 ( 7.152448122690996019E-18, 0.001328432419540397699, 0.002656864839080788025, 0.003985297258621178784, 0.004649513468391363973, 0.005313729678161549161 ),
 .UNSPECIFIED. ) ;
#69005=FACE_OUTER_BOUND ( 'NONE', #29307, .T. ) ;
#69009=ORIENTED_EDGE ( 'NONE', *, *, #34103, .T. ) ;
#69012=ORIENTED_EDGE ( 'NONE', *, *, #12663, .F. ) ;
#69019=DIRECTION ( 'NONE',  ( -0.000000000000000000, 1.000000000000000000, -0.000000000000000000 ) ) ;
#69023=CARTESIAN_POINT ( 'NONE',  ( 0.4314295484911171985, 1.339559522712171491, -2.637768908735144358 ) ) ;
#69029=VERTEX_POINT ( 'NONE', #75444 ) ;
#69058=DIRECTION ( 'NONE',  ( -3.491481338843132961E-15, -0.000000000000000000, 1.000000000000000000 ) ) ;
#69059=DIMENSIONAL_EXPONENTS ( 1.000000000000000000, 0.000000000000000000, 0.000000000000000000, 0.000000000000000000, 0.000000000000000000, 0.000000000000000000, 0.000000000000000000 ) ;
#69065=CARTESIAN_POINT ( 'NONE',  ( -2.610466197084866824, 1.379671404989095018, -0.4476723508032712240 ) ) ;
#69068=FACE_OUTER_BOUND ( 'NONE', #18725, .T. ) ;
#69071=EDGE_CURVE ( 'NONE', #48388, #24500, #24891, .T. ) ;
#69079=CARTESIAN_POINT ( 'NONE',  ( 0.3853249588699879657, 1.260224081467387958, -1.053849663494103250 ) ) ;
#69090=DIRECTION ( 'NONE',  ( 0.000000000000000000, 1.000000000000000000, -0.000000000000000000 ) ) ;
#69101=DIRECTION ( 'NONE',  ( -0.000000000000000000, 1.000000000000000000, -0.000000000000000000 ) ) ;
#69110=ORIENTED_EDGE ( 'NONE', *, *, #31423, .F. ) ;
#69126=CARTESIAN_POINT ( 'NONE',  ( -0.03411923929626390489, 1.063910482648554146, -1.851245305700470967 ) ) ;
#69138=VECTOR ( 'NONE', #67522, 39.37007874015748143 ) ;
#69141=DIRECTION ( 'NONE',  ( -0.000000000000000000, -1.000000000000000000, -1.408710688920637755E-15 ) ) ;
#69147=ORIENTED_EDGE ( 'NONE', *, *, #50692, .F. ) ;
#69151=DIRECTION ( 'NONE',  ( 1.000000000000000000, 0.000000000000000000, 1.047444401652940007E-14 ) ) ;
#69155=DIRECTION ( 'NONE',  ( -1.000000000000000000, -0.000000000000000000, -0.000000000000000000 ) ) ;
#69170=CARTESIAN_POINT ( 'NONE',  ( -0.01711686753222916441, 1.062992125984252301, 1.850393700787401619 ) ) ;
#69184=CARTESIAN_POINT ( 'NONE',  ( 1.121720580570839010, 1.063763119642385124, -0.03131331025603343449 ) ) ;
#69191=ADVANCED_FACE ( 'NONE', ( #64873 ), #81635, .F. ) ;
#69205=VERTEX_POINT ( 'NONE', #44648 ) ;
#69234=EDGE_CURVE ( 'NONE', #65182, #77311, #2322, .T. ) ;
#69251=VERTEX_POINT ( 'NONE', #63619 ) ;
#69254=CARTESIAN_POINT ( 'NONE',  ( 3.937007874015748143, 1.724409448818898127, 0.6299212598425202314 ) ) ;
#69259=LINE ( 'NONE', #75169, #66525 ) ;
#69260=FACE_OUTER_BOUND ( 'NONE', #7955, .T. ) ;
#69271=CARTESIAN_POINT ( 'NONE',  ( -0.4359958488159582091, 1.724409448818897905, -3.937007874015763687 ) ) ;
#69303=VERTEX_POINT ( 'NONE', #25304 ) ;
#69315=CARTESIAN_POINT ( 'NONE',  ( 0.3535010496217478315, 1.220715222164475922, -1.393813936465888359 ) ) ;
#69327=CYLINDRICAL_SURFACE ( 'NONE', #59993, 0.5118110236220471121 ) ;
#69328=AXIS2_PLACEMENT_3D ( 'NONE', #60262, #23089, #59012 ) ;
#69342=VERTEX_POINT ( 'NONE', #19419 ) ;
#69354=DIRECTION ( 'NONE',  ( -3.491481338843132961E-15, -0.000000000000000000, 1.000000000000000000 ) ) ;
#69363=ORIENTED_EDGE ( 'NONE', *, *, #76206, .F. ) ;
#69369=LINE ( 'NONE', #44086, #26423 ) ;
#69372=AXIS2_PLACEMENT_3D ( 'NONE', #20102, #75794, #43770 ) ;
#69388=VECTOR ( 'NONE', #19146, 39.37007874015748143 ) ;
#69389=CARTESIAN_POINT ( 'NONE',  ( -1.882930639362831116, 1.098283573398308954, 0.1802708669123980201 ) ) ;
#69392=ADVANCED_FACE ( 'NONE', ( #58122 ), #25003, .T. ) ;
#69408=CARTESIAN_POINT ( 'NONE',  ( -3.936915166329627347, 1.063759665227983708, -0.03114301994267879015 ) ) ;
#69412=PLANE ( 'NONE',  #11193 ) ;
#69413=ORIENTED_EDGE ( 'NONE', *, *, #32546, .F. ) ;
#69414=DIRECTION ( 'NONE',  ( -0.000000000000000000, -1.000000000000000000, -0.000000000000000000 ) ) ;
#69422=CARTESIAN_POINT ( 'NONE',  ( -2.554262525012222174, 1.537401574803149984, 0.4744094488188970171 ) ) ;
#69423=AXIS2_PLACEMENT_3D ( 'NONE', #46617, #8746, #40316 ) ;
#69424=CIRCLE ( 'NONE', #82942, 3.937007874015748143 ) ;
#69428=ORIENTED_EDGE ( 'NONE', *, *, #890, .F. ) ;
#69444=ORIENTED_EDGE ( 'NONE', *, *, #3777, .F. ) ;
#69448=VECTOR ( 'NONE', #65223, 39.37007874015748143 ) ;
#69474=LINE ( 'NONE', #62323, #63351 ) ;
#69479=CARTESIAN_POINT ( 'NONE',  ( -2.759487654322792416, 1.189595890467141759, 0.3229789317950594874 ) ) ;
#69482=VECTOR ( 'NONE', #78552, 39.37007874015748143 ) ;
#69486=CIRCLE ( 'NONE', #31855, 3.858267716535433323 ) ;
#69487=AXIS2_PLACEMENT_3D ( 'NONE', #82602, #11074, #62833 ) ;
#69495=CARTESIAN_POINT ( 'NONE',  ( 0.4490240974115876638, 1.383493637049404423, -1.028295962660220608 ) ) ;
#69498=CARTESIAN_POINT ( 'NONE',  ( 0.4732434500808813116, 1.503067092966738683, -2.167287614618209179 ) ) ;
#69503=CARTESIAN_POINT ( 'NONE',  ( -0.4744094488188831948, 1.521917890488208469, -3.908320185825792770 ) ) ;
#69516=CARTESIAN_POINT ( 'NONE',  ( -2.154527559055123831, 0.03937007874015747977, 0.4677827689124697264 ) ) ;
#69540=VECTOR ( 'NONE', #28181, 39.37007874015748143 ) ;
#69541=CARTESIAN_POINT ( 'NONE',  ( -0.5314960629921324786, 2.716535433070866645, 1.854472803289050509 ) ) ;
#69561=ORIENTED_EDGE ( 'NONE', *, *, #1707, .T. ) ;
#69562=EDGE_LOOP ( 'NONE', ( #36952, #49558, #59895, #47289 ) ) ;
#69569=DIRECTION ( 'NONE',  ( 0.000000000000000000, -1.000000000000000000, -0.000000000000000000 ) ) ;
#69591=DIRECTION ( 'NONE',  ( 0.000000000000000000, 0.000000000000000000, 1.000000000000000000 ) ) ;
#69599=CARTESIAN_POINT ( 'NONE',  ( 1.053828262837742225, 1.260305573253202915, 0.3853833445747810726 ) ) ;
#69615=EDGE_CURVE ( 'NONE', #21108, #43005, #76666, .T. ) ;
#69630=CARTESIAN_POINT ( 'NONE',  ( -0.2894808532238192234, 1.161235014983161173, 1.084132210936307628 ) ) ;
#69637=EDGE_CURVE ( 'NONE', #80330, #11040, #51862, .T. ) ;
#69659=ORIENTED_EDGE ( 'NONE', *, *, #32546, .T. ) ;
#69661=ORIENTED_EDGE ( 'NONE', *, *, #27842, .T. ) ;
#69668=DIRECTION ( 'NONE',  ( 0.000000000000000000, 0.000000000000000000, -1.000000000000000000 ) ) ;
#69676=ORIENTED_EDGE ( 'NONE', *, *, #62649, .F. ) ;
#69678=FACE_OUTER_BOUND ( 'NONE', #74834, .T. ) ;
#69686=CARTESIAN_POINT ( 'NONE',  ( 0.5314960629921061663, 2.755905511811024056, 1.895394334970797345 ) ) ;
#69712=ORIENTED_EDGE ( 'NONE', *, *, #36661, .T. ) ;
#69724=CARTESIAN_POINT ( 'NONE',  ( 0.08477834984147555875, 1.070319560067212850, 2.867229352980811274 ) ) ;
#69728=DIRECTION ( 'NONE',  ( 1.000000000000000000, -0.000000000000000000, -0.000000000000000000 ) ) ;
#69731=EDGE_CURVE ( 'NONE', #67621, #57500, #76107, .T. ) ;
#69736=CARTESIAN_POINT ( 'NONE',  ( -3.937007874015748143, 2.165354330708661568, 0.6299212598425196763 ) ) ;
#69739=ORIENTED_EDGE ( 'NONE', *, *, #35062, .T. ) ;
#69759=DIRECTION ( 'NONE',  ( -0.000000000000000000, -1.000000000000000000, -0.000000000000000000 ) ) ;
#69761=CYLINDRICAL_SURFACE ( 'NONE', #60388, 0.3149606299212597826 ) ;
#69773=ORIENTED_EDGE ( 'NONE', *, *, #511, .T. ) ;
#69780=CARTESIAN_POINT ( 'NONE',  ( -0.5314960629921122726, 2.755905511811024056, -3.937007874015763687 ) ) ;
#69797=CARTESIAN_POINT ( 'NONE',  ( -1.915796337058206955, 1.134406187872333938, 0.2508088161067916766 ) ) ;
#69821=ORIENTED_EDGE ( 'NONE', *, *, #7492, .T. ) ;
#69822=FACE_OUTER_BOUND ( 'NONE', #50363, .T. ) ;
#69827=CARTESIAN_POINT ( 'NONE',  ( -0.5314960629921172686, 2.755905511811024056, -2.503252890251017604 ) ) ;
#69830=LINE ( 'NONE', #63515, #52977 ) ;
#69834=ORIENTED_EDGE ( 'NONE', *, *, #10031, .F. ) ;
#69849=ORIENTED_EDGE ( 'NONE', *, *, #23437, .T. ) ;
#69856=EDGE_CURVE ( 'NONE', #10035, #61855, #55777, .T. ) ;
#69884=CARTESIAN_POINT ( 'NONE',  ( -2.704643427489245244, 1.253539720428387572, -0.3811758253792954521 ) ) ;
#69899=CARTESIAN_POINT ( 'NONE',  ( 0.2248261898302408024, 1.118407866122129724, -1.901322016725929931 ) ) ;
#69904=CARTESIAN_POINT ( 'NONE',  ( -0.2375791879843439092, 1.126472371288131047, -3.929857012155298257 ) ) ;
#69916=CARTESIAN_POINT ( 'NONE',  ( 1.854472803289052507, 2.716535433070866645, -0.5314960629921260393 ) ) ;
#69917=CARTESIAN_POINT ( 'NONE',  ( 1.348312163386739204, 1.122131950691689140, 0.7386866130305692613 ) ) ;
#69930=DIRECTION ( 'NONE',  ( -0.000000000000000000, -1.000000000000000000, -0.000000000000000000 ) ) ;
#69932=CARTESIAN_POINT ( 'NONE',  ( 0.5314960629921372526, 2.716535433070866645, -3.224202737261813834 ) ) ;
#69942=FACE_OUTER_BOUND ( 'NONE', #72041, .T. ) ;
#69943=EDGE_LOOP ( 'NONE', ( #54533, #38166, #68503 ) ) ;
#69962=ORIENTED_EDGE ( 'NONE', *, *, #82449, .F. ) ;
#69963=ORIENTED_EDGE ( 'NONE', *, *, #15090, .F. ) ;
#70000=DIRECTION ( 'NONE',  ( 0.000000000000000000, 1.000000000000000000, -0.000000000000000000 ) ) ;
#70014=EDGE_CURVE ( 'NONE', #32076, #27377, #4859, .T. ) ;
#70016=CIRCLE ( 'NONE', #33750, 1.968503937007874072 ) ;
#70018=ORIENTED_EDGE ( 'NONE', *, *, #46613, .T. ) ;
#70030=CARTESIAN_POINT ( 'NONE',  ( -0.4252145377707324814, 1.326453916767273977, 1.038386062493871886 ) ) ;
#70057=EDGE_LOOP ( 'NONE', ( #29698, #72646, #47410, #4533 ) ) ;
#70060=DIRECTION ( 'NONE',  ( 0.000000000000000000, 0.000000000000000000, -1.000000000000000000 ) ) ;
#70065=DIRECTION ( 'NONE',  ( 0.000000000000000000, 0.000000000000000000, -1.000000000000000000 ) ) ;
#70066=DIRECTION ( 'NONE',  ( -8.881784197001252323E-16, -9.738798461624180871E-16, 1.000000000000000000 ) ) ;
#70073=ORIENTED_EDGE ( 'NONE', *, *, #64982, .F. ) ;
#70074=ADVANCED_FACE ( 'NONE', ( #48232 ), #42496, .F. ) ;
#70078=CARTESIAN_POINT ( 'NONE',  ( 0.4128810003509036930, 1.303691442895980490, -1.728827638849821824 ) ) ;
#70082=ORIENTED_EDGE ( 'NONE', *, *, #12663, .T. ) ;
#70109=VECTOR ( 'NONE', #60764, 39.37007874015748143 ) ;
#70111=ORIENTED_EDGE ( 'NONE', *, *, #23437, .F. ) ;
#70125=CARTESIAN_POINT ( 'NONE',  ( 0.000000000000000000, 0.000000000000000000, 2.362204724409448620 ) ) ;
#70136=DIRECTION ( 'NONE',  ( 0.000000000000000000, 1.000000000000000000, 0.000000000000000000 ) ) ;
#70152=ORIENTED_EDGE ( 'NONE', *, *, #50364, .T. ) ;
#70154=ORIENTED_EDGE ( 'NONE', *, *, #69615, .F. ) ;
#70164=DIRECTION ( 'NONE',  ( -3.491481338843132961E-15, 0.000000000000000000, 1.000000000000000000 ) ) ;
#70174=CIRCLE ( 'NONE', #12388, 2.637795275590551380 ) ;
#70216=DIRECTION ( 'NONE',  ( 0.000000000000000000, 0.000000000000000000, -1.000000000000000000 ) ) ;
#70218=EDGE_CURVE ( 'NONE', #41616, #22014, #10908, .T. ) ;
#70221=CARTESIAN_POINT ( 'NONE',  ( -0.4485266855423988286, 1.695194674715583494, 1.028590675108155716 ) ) ;
#70222=AXIS2_PLACEMENT_3D ( 'NONE', #83130, #82315, #44793 ) ;
#70224=ORIENTED_EDGE ( 'NONE', *, *, #58316, .T. ) ;
#70240=ORIENTED_EDGE ( 'NONE', *, *, #45026, .T. ) ;
#70246=CARTESIAN_POINT ( 'NONE',  ( -1.313877454013331780, 0.2929341459200028863, 0.6999040823587868720 ) ) ;
#70259=CARTESIAN_POINT ( 'NONE',  ( 2.554262525012262586, 1.537401574803149984, -0.4744094488188970171 ) ) ;
#70277=EDGE_CURVE ( 'NONE', #37754, #66965, #43689, .T. ) ;
#70286=CIRCLE ( 'NONE', #55502, 0.2165354330708659791 ) ;
#70290=CARTESIAN_POINT ( 'NONE',  ( -2.594245572444953130, 1.668131542012049717, -0.4562955581495596324 ) ) ;
#70307=CARTESIAN_POINT ( 'NONE',  ( -3.900966923095589678, 2.677165354330708791, -0.5314960629921260393 ) ) ;
#70310=DIRECTION ( 'NONE',  ( 0.000000000000000000, 0.000000000000000000, 1.000000000000000000 ) ) ;
#70316=CARTESIAN_POINT ( 'NONE',  ( -0.2508553453239640851, 1.134444486973533062, -3.929028906623472928 ) ) ;
#70330=PLANE ( 'NONE',  #251 ) ;
#70341=AXIS2_PLACEMENT_3D ( 'NONE', #56794, #77002, #50477 ) ;
#70371=FACE_OUTER_BOUND ( 'NONE', #57914, .T. ) ;
#70374=EDGE_LOOP ( 'NONE', ( #8448, #40174, #7460, #9726, #75252, #46480, #39223, #32190, #80005, #3737, #64366, #8893, #41075, #9850 ) ) ;
#70375=ORIENTED_EDGE ( 'NONE', *, *, #238, .T. ) ;
#70416=FACE_OUTER_BOUND ( 'NONE', #42732, .T. ) ;
#70444=AXIS2_PLACEMENT_3D ( 'NONE', #69254, #82300, #49470 ) ;
#70455=CARTESIAN_POINT ( 'NONE',  ( 0.000000000000000000, 1.724409448818897905, 0.000000000000000000 ) ) ;
#70458=AXIS2_PLACEMENT_3D ( 'NONE', #49223, #42902, #50454 ) ;
#70472=ORIENTED_EDGE ( 'NONE', *, *, #71659, .T. ) ;
#70474=VERTEX_POINT ( 'NONE', #49607 ) ;
#70480=CARTESIAN_POINT ( 'NONE',  ( -0.4672469119858430053, 1.453788974454129912, 2.571228699324735079 ) ) ;
#70488=EDGE_LOOP ( 'NONE', ( #38388, #50460, #14793, #53306 ) ) ;
#70497=DIRECTION ( 'NONE',  ( 0.000000000000000000, 0.000000000000000000, -1.000000000000000000 ) ) ;
#70504=CIRCLE ( 'NONE', #10025, 3.937007874015748143 ) ;
#70521=DIRECTION ( 'NONE',  ( 0.000000000000000000, 0.000000000000000000, 1.000000000000000000 ) ) ;
#70525=ORIENTED_EDGE ( 'NONE', *, *, #36983, .F. ) ;
#70540=CARTESIAN_POINT ( 'NONE',  ( 0.4744094488188886349, 1.546132656481029599, 2.554262525012303886 ) ) ;
#70552=DIRECTION ( 'NONE',  ( 1.000000000000000000, -0.000000000000000000, -0.000000000000000000 ) ) ;
#70562=LINE ( 'NONE', #71405, #12739 ) ;
#70581=AXIS2_PLACEMENT_3D ( 'NONE', #74322, #41081, #78988 ) ;
#70590=ORIENTED_EDGE ( 'NONE', *, *, #34333, .T. ) ;
#70597=CARTESIAN_POINT ( 'NONE',  ( -3.900966923095589678, 2.677165354330708791, 0.5314960629921260393 ) ) ;
#70610=CARTESIAN_POINT ( 'NONE',  ( -0.04000121214432307559, 1.064648596787614032, -1.441347525760512838 ) ) ;
#70634=AXIS2_PLACEMENT_3D ( 'NONE', #30357, #30775, #56436 ) ;
#70637=CARTESIAN_POINT ( 'NONE',  ( -3.908778449111570463, 1.475589138410839052, -0.4706212595521235831 ) ) ;
#70645=DIRECTION ( 'NONE',  ( -0.000000000000000000, -1.000000000000000000, -0.000000000000000000 ) ) ;
#70657=B_SPLINE_CURVE_WITH_KNOTS ( 'NONE', 3,
 ( #55085, #66086, #2108, #9667, #54679, #60590, #79558, #22290, #35336, #48361, #53437, #47536, #73654, #9256 ),
 .UNSPECIFIED., .F., .F.,
 ( 4, 2, 2, 2, 2, 2, 4 ),
 ( 0.000000000000000000, 0.0003923887041693363098, 0.0007847774083386726196, 0.001177166112508008875, 0.001569554816677345239, 0.002354332225016047241, 0.003139109633354749025 ),
 .UNSPECIFIED. ) ;
#70659=ORIENTED_EDGE ( 'NONE', *, *, #1862, .F. ) ;
#70677=ORIENTED_EDGE ( 'NONE', *, *, #2876, .F. ) ;
#70679=ORIENTED_EDGE ( 'NONE', *, *, #18297, .T. ) ;
#70682=CIRCLE ( 'NONE', #39806, 0.5118110236220471121 ) ;
#70686=ADVANCED_FACE ( 'NONE', ( #39473 ), #766, .F. ) ;
#70713=EDGE_CURVE ( 'NONE', #63415, #43601, #22191, .T. ) ;
#70714=CARTESIAN_POINT ( 'NONE',  ( -2.586063147568568699, 1.653225543546882781, -0.4603267246303533455 ) ) ;
#70741=VECTOR ( 'NONE', #17079, 39.37007874015748143 ) ;
#70743=CARTESIAN_POINT ( 'NONE',  ( -0.2893689214265932619, 1.160196156542221413, -3.926443535894562409 ) ) ;
#70748=CARTESIAN_POINT ( 'NONE',  ( -0.03443470937339728616, 0.2929341459200028863, -1.537015892239756099 ) ) ;
#70756=DIRECTION ( 'NONE',  ( 0.000000000000000000, -1.000000000000000000, 0.000000000000000000 ) ) ;
#70760=B_SPLINE_CURVE_WITH_KNOTS ( 'NONE', 3,
 ( #14843, #66599, #27872, #41336, #47634, #73328, #16505, #35847, #54361, #80073, #61096, #22390, #15258, #15675, #10182, #28699, #67426, #35020, #55182, #40503, #61516, #80484, #22797, #3861, #59852, #60275, #67016, #79240 ),
 .UNSPECIFIED., .F., .F.,
 ( 4, 2, 2, 2, 2, 2, 2, 2, 2, 2, 2, 2, 2, 4 ),
 ( 0.01906920098334001501, 0.02026021391800203117, 0.02145122685266404733, 0.02264223978732606696, 0.02383325272198808312, 0.02621527859131211544, 0.02740629152597413160, 0.02859730446063614429, 0.03097933032996016273, 0.03217034326462216154, 0.03336135619928416729, 0.03574338206860819267, 0.03693439500327019842, 0.03812540793793221111 ),
 .UNSPECIFIED. ) ;
#70762=CIRCLE ( 'NONE', #72097, 1.122047244094488194 ) ;
#70766=ORIENTED_EDGE ( 'NONE', *, *, #49461, .T. ) ;
#70784=CARTESIAN_POINT ( 'NONE',  ( -0.4567483893478792578, 1.408297760469687798, -2.131068205843717145 ) ) ;
#70788=ORIENTED_EDGE ( 'NONE', *, *, #68011, .F. ) ;
#70800=CARTESIAN_POINT ( 'NONE',  ( -0.5314960629921396951, 2.697992270790283698, 3.898836503597931991 ) ) ;
#70802=DIRECTION ( 'NONE',  ( 0.000000000000000000, -0.000000000000000000, -1.000000000000000000 ) ) ;
#70804=VERTEX_POINT ( 'NONE', #39897 ) ;
#70805=AXIS2_PLACEMENT_3D ( 'NONE', #36352, #41833, #42660 ) ;
#70809=AXIS2_PLACEMENT_3D ( 'NONE', #50676, #51080, #31740 ) ;
#70814=EDGE_CURVE ( 'NONE', #48318, #77301, #82826, .T. ) ;
#70822=EDGE_CURVE ( 'NONE', #79813, #65941, #45768, .T. ) ;
#70834=CARTESIAN_POINT ( 'NONE',  ( -0.4122368018044647031, 1.300920202588027541, 2.057881464606095889 ) ) ;
#70845=DIRECTION ( 'NONE',  ( 1.000000000000000000, -0.000000000000000000, -0.000000000000000000 ) ) ;
#70875=CARTESIAN_POINT ( 'NONE',  ( -3.924389226575468737, 2.755905511811024056, 0.3149606299212597271 ) ) ;
#70902=ORIENTED_EDGE ( 'NONE', *, *, #9160, .T. ) ;
#70904=ORIENTED_EDGE ( 'NONE', *, *, #4484, .F. ) ;
#70918=ORIENTED_EDGE ( 'NONE', *, *, #1240, .T. ) ;
#70919=CARTESIAN_POINT ( 'NONE',  ( -1.044296345234789758, 1.299058944788251901, -0.4104848940941682733 ) ) ;
#70927=CIRCLE ( 'NONE', #49409, 1.122047244094488194 ) ;
#70930=CARTESIAN_POINT ( 'NONE',  ( 0.000000000000000000, 2.165354330708661568, 0.000000000000000000 ) ) ;
#70936=CARTESIAN_POINT ( 'NONE',  ( -0.4359958488159647039, 1.724409448818897905, -2.094141031014960408 ) ) ;
#70951=FACE_OUTER_BOUND ( 'NONE', #60463, .T. ) ;
#70955=ORIENTED_EDGE ( 'NONE', *, *, #43993, .F. ) ;
#70982=ORIENTED_EDGE ( 'NONE', *, *, #32702, .T. ) ;
#71000=DIRECTION ( 'NONE',  ( -1.000000000000000000, -0.000000000000000000, -0.000000000000000000 ) ) ;
#71009=CARTESIAN_POINT ( 'NONE',  ( 0.4603267246303430760, 1.653225543546893439, 2.138346301250358739 ) ) ;
#71023=CARTESIAN_POINT ( 'NONE',  ( -2.103512204792533868, 1.710976477253047801, 0.4417575354491484751 ) ) ;
#71031=CARTESIAN_POINT ( 'NONE',  ( -0.5314960629921147151, 2.716535433070866645, -3.224202737261816942 ) ) ;
#71037=CARTESIAN_POINT ( 'NONE',  ( -0.03443470937339819515, 1.064243487142144673, -1.633358474390059989 ) ) ;
#71050=CARTESIAN_POINT ( 'NONE',  ( -3.937007874015748143, 2.165354330708662012, -0.6299212598425202314 ) ) ;
#71064=CARTESIAN_POINT ( 'NONE',  ( -3.918945891830401429, 1.247862022481391886, -0.3770874914321828419 ) ) ;
#71068=LINE ( 'NONE', #26447, #68977 ) ;
#71069=B_SPLINE_CURVE_WITH_KNOTS ( 'NONE', 3,
 ( #49477, #49059, #30536, #31347 ),
 .UNSPECIFIED., .F., .F.,
 ( 4, 4 ),
 ( 0.08422315286269926871, 0.08567085022608394995 ),
 .UNSPECIFIED. ) ;
#71073=CARTESIAN_POINT ( 'NONE',  ( -1.291027602697912169, 0.2755905511811023723, 0.5830028338522510456 ) ) ;
#71085=ORIENTED_EDGE ( 'NONE', *, *, #21721, .F. ) ;
#71087=ORIENTED_EDGE ( 'NONE', *, *, #71221, .T. ) ;
#71103=ORIENTED_EDGE ( 'NONE', *, *, #23392, .F. ) ;
#71135=EDGE_CURVE ( 'NONE', #80330, #17178, #33166, .T. ) ;
#71156=ADVANCED_FACE ( 'NONE', ( #65585 ), #54580, .F. ) ;
#71175=CARTESIAN_POINT ( 'NONE',  ( 0.4724973665168182846, 1.580780302271975080, -2.165475543433776462 ) ) ;
#71203=ORIENTED_EDGE ( 'NONE', *, *, #40191, .T. ) ;
#71221=EDGE_CURVE ( 'NONE', #47373, #39419, #1187, .T. ) ;
#71223=FACE_OUTER_BOUND ( 'NONE', #63504, .T. ) ;
#71225=ORIENTED_EDGE ( 'NONE', *, *, #37212, .F. ) ;
#71229=DIRECTION ( 'NONE',  ( 0.000000000000000000, 0.000000000000000000, -1.000000000000000000 ) ) ;
#71235=DIRECTION ( 'NONE',  ( 0.000000000000000000, 0.000000000000000000, -1.000000000000000000 ) ) ;
#71253=CARTESIAN_POINT ( 'NONE',  ( -0.4732185887570871108, 1.572090529166659811, 2.167227123902327079 ) ) ;
#71268=DIRECTION ( 'NONE',  ( 1.408710688920637755E-15, -1.000000000000000000, 4.918487082195260922E-30 ) ) ;
#71278=LINE ( 'NONE', #46001, #1874 ) ;
#71282=ADVANCED_FACE ( 'NONE', ( #79459, #41956 ), #66829, .F. ) ;
#71286=DIRECTION ( 'NONE',  ( 0.000000000000000000, 1.000000000000000000, -0.000000000000000000 ) ) ;
#71297=CARTESIAN_POINT ( 'NONE',  ( -0.4741627488320071526, 1.554989095716458269, -2.169534490215677902 ) ) ;
#71318=ORIENTED_EDGE ( 'NONE', *, *, #82137, .F. ) ;
#71331=ORIENTED_EDGE ( 'NONE', *, *, #30606, .T. ) ;
#71332=AXIS2_PLACEMENT_3D ( 'NONE', #18227, #29193, #3527 ) ;
#71335=LINE ( 'NONE', #7357, #73471 ) ;
#71347=DIRECTION ( 'NONE',  ( -0.000000000000000000, -1.000000000000000000, -0.000000000000000000 ) ) ;
#71351=AXIS2_PLACEMENT_3D ( 'NONE', #21082, #2139, #27807 ) ;
#71365=FACE_OUTER_BOUND ( 'NONE', #55634, .T. ) ;
#71385=CARTESIAN_POINT ( 'NONE',  ( 1.018747574612958173, 1.602034772339061330, 0.4702623840880322259 ) ) ;
#71399=ORIENTED_EDGE ( 'NONE', *, *, #27431, .F. ) ;
#71405=CARTESIAN_POINT ( 'NONE',  ( 1.348312163386739426, 0.2755905511811023723, 0.6195921248415929838 ) ) ;
#71407=AXIS2_PLACEMENT_3D ( 'NONE', #35013, #66591, #81294 ) ;
#71415=ORIENTED_EDGE ( 'NONE', *, *, #69731, .F. ) ;
#71425=CARTESIAN_POINT ( 'NONE',  ( -3.937007874015748143, 1.537401574803149984, -2.901595197523589142E-16 ) ) ;
#71427=CARTESIAN_POINT ( 'NONE',  ( -0.01115035570243675701, 1.063087231634078922, -1.441367282966121488 ) ) ;
#71433=VERTEX_POINT ( 'NONE', #42365 ) ;
#71440=DIRECTION ( 'NONE',  ( 0.000000000000000000, 1.000000000000000000, -0.000000000000000000 ) ) ;
#71473=CARTESIAN_POINT ( 'NONE',  ( -2.556891446142596447, 2.729656600850901782, -0.5314960629921260393 ) ) ;
#71490=CARTESIAN_POINT ( 'NONE',  ( -3.861135848600278475, 2.745602313593968447, -0.5314960629921260393 ) ) ;
#71498=CARTESIAN_POINT ( 'NONE',  ( 0.3134705033195891999, 1.179969644333642709, -3.924569983224646563 ) ) ;
#71499=CARTESIAN_POINT ( 'NONE',  ( -0.3149606299212633909, 2.559055118110236560, 1.076935383196056417 ) ) ;
#71502=ORIENTED_EDGE ( 'NONE', *, *, #39374, .F. ) ;
#71504=EDGE_LOOP ( 'NONE', ( #17667, #79322, #62958, #1551 ) ) ;
#71513=CIRCLE ( 'NONE', #76913, 0.09842519685039351207 ) ;
#71518=ORIENTED_EDGE ( 'NONE', *, *, #69234, .F. ) ;
#71523=CARTESIAN_POINT ( 'NONE',  ( 2.822444539845176958, 1.119136672863569881, -0.2244172274865228744 ) ) ;
#71552=CARTESIAN_POINT ( 'NONE',  ( 3.886287458032462006, 1.724409448818897905, -0.6299212598425196763 ) ) ;
#71555=LINE ( 'NONE', #25671, #18417 ) ;
#71562=CARTESIAN_POINT ( 'NONE',  ( 1.348312163386739426, 1.062992125984252079, 0.6402614161801758463 ) ) ;
#71586=ORIENTED_EDGE ( 'NONE', *, *, #44453, .F. ) ;
#71597=DIRECTION ( 'NONE',  ( 0.000000000000000000, 8.673617379884024625E-16, 1.000000000000000000 ) ) ;
#71612=EDGE_CURVE ( 'NONE', #72444, #39742, #42379, .T. ) ;
#71617=DIRECTION ( 'NONE',  ( 0.000000000000000000, -1.000000000000000000, 0.000000000000000000 ) ) ;
#71628=AXIS2_PLACEMENT_3D ( 'NONE', #81257, #36611, #62290 ) ;
#71637=CARTESIAN_POINT ( 'NONE',  ( -0.5314960629921395840, 2.748002881374839834, 3.856579543051779524 ) ) ;
#71639=FACE_OUTER_BOUND ( 'NONE', #44663, .T. ) ;
#71640=ADVANCED_FACE ( 'NONE', ( #74813 ), #10825, .F. ) ;
#71647=CARTESIAN_POINT ( 'NONE',  ( 0.9881811337016640495, 2.755905511811024056, -0.5314960629921260393 ) ) ;
#71659=EDGE_CURVE ( 'NONE', #25547, #40163, #41971, .T. ) ;
#71666=CARTESIAN_POINT ( 'NONE',  ( 1.392101432702376629, 0.2755905511811023723, 0.9507481457704560768 ) ) ;
#71670=DIRECTION ( 'NONE',  ( 0.000000000000000000, 0.000000000000000000, -1.000000000000000000 ) ) ;
#71673=AXIS2_PLACEMENT_3D ( 'NONE', #76440, #24663, #70521 ) ;
#71677=CARTESIAN_POINT ( 'NONE',  ( 1.038339513766209476, 1.326687365142510178, -0.4253272082265546761 ) ) ;
#71686=DIRECTION ( 'NONE',  ( -0.000000000000000000, 0.000000000000000000, -1.000000000000000000 ) ) ;
#71733=EDGE_LOOP ( 'NONE', ( #67807, #78668, #18900, #50590 ) ) ;
#71735=ORIENTED_EDGE ( 'NONE', *, *, #58451, .T. ) ;
#71740=CARTESIAN_POINT ( 'NONE',  ( -0.4498537592782897998, 0.000000000000000000, 2.118110236220472675 ) ) ;
#71745=CARTESIAN_POINT ( 'NONE',  ( 0.4744094488189112835, 1.537401574803149984, -3.908320185825791881 ) ) ;
#71752=CARTESIAN_POINT ( 'NONE',  ( -0.03443470937339728616, 0.000000000000000000, -1.753551325310622078 ) ) ;
#71756=EDGE_LOOP ( 'NONE', ( #81795, #15604, #68096, #31853, #30403, #50285, #53718, #45063, #18403, #83165, #60237, #38586, #69110, #6405 ) ) ;
#71757=DIRECTION ( 'NONE',  ( 1.000000000000000000, -0.000000000000000000, -0.000000000000000000 ) ) ;
#71759=ADVANCED_FACE ( 'NONE', ( #4501 ), #5330, .F. ) ;
#71784=CYLINDRICAL_SURFACE ( 'NONE', #46112, 0.2165354330708660069 ) ;
#71805=VECTOR ( 'NONE', #17677, 39.37007874015748143 ) ;
#71820=ORIENTED_EDGE ( 'NONE', *, *, #78000, .F. ) ;
#71836=ORIENTED_EDGE ( 'NONE', *, *, #38498, .T. ) ;
#71846=DIRECTION ( 'NONE',  ( 0.000000000000000000, 0.000000000000000000, -1.000000000000000000 ) ) ;
#71847=FACE_OUTER_BOUND ( 'NONE', #56480, .T. ) ;
#71849=DIRECTION ( 'NONE',  ( 0.000000000000000000, 0.000000000000000000, 1.000000000000000000 ) ) ;
#71852=CIRCLE ( 'NONE', #73171, 0.2165354330708660069 ) ;
#71862=CARTESIAN_POINT ( 'NONE',  ( 2.159196716653021930, 1.469708627452553928, 0.4698506773045486029 ) ) ;
#71873=VECTOR ( 'NONE', #81074, 39.37007874015748143 ) ;
#71892=PLANE ( 'NONE',  #19672 ) ;
#71894=CARTESIAN_POINT ( 'NONE',  ( 1.348312163386739426, 0.2755905511811023723, 0.6195921248415929838 ) ) ;
#71910=ORIENTED_EDGE ( 'NONE', *, *, #26715, .T. ) ;
#71920=CARTESIAN_POINT ( 'NONE',  ( 0.4744094488189115055, 1.506021921081838633, -3.908320185825790993 ) ) ;
#71944=CARTESIAN_POINT ( 'NONE',  ( -1.545038802164343306, 1.128537896298102305, 0.2406134192599649335 ) ) ;
#71951=CARTESIAN_POINT ( 'NONE',  ( -0.9881811337016640495, 2.755905511811024056, -0.5314960629921260393 ) ) ;
#71977=CARTESIAN_POINT ( 'NONE',  ( -2.557132292622109837, 1.503024749832831519, -0.4732391302016651369 ) ) ;
#72014=CARTESIAN_POINT ( 'NONE',  ( 0.4732141852945755400, 1.572163861244850303, -2.167216380768100858 ) ) ;
#72015=DIRECTION ( 'NONE',  ( 0.000000000000000000, 0.000000000000000000, -1.000000000000000000 ) ) ;
#72022=EDGE_LOOP ( 'NONE', ( #25221, #47056 ) ) ;
#72031=CARTESIAN_POINT ( 'NONE',  ( 5.333846858410640380E-15, 1.062992125984252079, -1.444810848096780953 ) ) ;
#72041=EDGE_LOOP ( 'NONE', ( #16775, #54307, #25338, #7224 ) ) ;
#72097=AXIS2_PLACEMENT_3D ( 'NONE', #13788, #20514, #20928 ) ;
#72104=CARTESIAN_POINT ( 'NONE',  ( -1.559171609364246924, 0.3937007874015747699, 0.6156134192599649335 ) ) ;
#72131=DIRECTION ( 'NONE',  ( 0.000000000000000000, 1.000000000000000000, -0.000000000000000000 ) ) ;
#72132=VECTOR ( 'NONE', #30551, 39.37007874015748143 ) ;
#72153=VERTEX_POINT ( 'NONE', #19188 ) ;
#72155=ORIENTED_EDGE ( 'NONE', *, *, #4418, .T. ) ;
#72159=CARTESIAN_POINT ( 'NONE',  ( -0.4477177017962782335, 1.379801381128185511, 2.610383882218336282 ) ) ;
#72175=EDGE_LOOP ( 'NONE', ( #76557, #55971, #11199, #9524, #30799, #6136 ) ) ;
#72177=FACE_OUTER_BOUND ( 'NONE', #54198, .T. ) ;
#72187=EDGE_CURVE ( 'NONE', #59983, #15514, #50594, .T. ) ;
#72195=CARTESIAN_POINT ( 'NONE',  ( 2.516666458167341691, 2.742784437388869012, 0.5314960629921260393 ) ) ;
#72198=CIRCLE ( 'NONE', #58720, 0.3149606299212598381 ) ;
#72207=CARTESIAN_POINT ( 'NONE',  ( -1.313877454013331780, 0.2755905511811023723, 0.7983292792091805090 ) ) ;
#72213=ORIENTED_EDGE ( 'NONE', *, *, #45608, .T. ) ;
#72215=EDGE_CURVE ( 'NONE', #8202, #36894, #66141, .T. ) ;
#72229=CARTESIAN_POINT ( 'NONE',  ( 0.4417590601942769646, 1.710972922415834097, 2.620894764083904871 ) ) ;
#72241=ORIENTED_EDGE ( 'NONE', *, *, #63554, .T. ) ;
#72246=DIRECTION ( 'NONE',  ( 0.000000000000000000, 0.000000000000000000, -1.000000000000000000 ) ) ;
#72255=ORIENTED_EDGE ( 'NONE', *, *, #79291, .T. ) ;
#72257=ORIENTED_EDGE ( 'NONE', *, *, #18704, .T. ) ;
#72263=CARTESIAN_POINT ( 'NONE',  ( 0.4177787735907000366, 0.3937007874015748254, -1.559171609364239375 ) ) ;
#72274=EDGE_LOOP ( 'NONE', ( #21111, #67686, #55968, #32341, #67558, #73418, #49467, #22565, #41419, #64483, #45925, #62699 ) ) ;
#72282=EDGE_CURVE ( 'NONE', #52658, #76474, #12196, .T. ) ;
#72283=CARTESIAN_POINT ( 'NONE',  ( 2.165607527688952594, 1.494646310179101656, -0.4725519687354808873 ) ) ;
#72306=CARTESIAN_POINT ( 'NONE',  ( 0.4411264095795432993, 1.362677836172179635, -1.627053844800393501 ) ) ;
#72308=CARTESIAN_POINT ( 'NONE',  ( -1.017203447268042016, 1.569595554511555857, -0.4735931522784879721 ) ) ;
#72312=FACE_OUTER_BOUND ( 'NONE', #56711, .T. ) ;
#72329=DIRECTION ( 'NONE',  ( 0.000000000000000000, -0.000000000000000000, 1.000000000000000000 ) ) ;
#72338=CARTESIAN_POINT ( 'NONE',  ( 3.890345922373659615, 2.716830163678111365, 0.5314960629921260393 ) ) ;
#72344=ORIENTED_EDGE ( 'NONE', *, *, #10031, .T. ) ;
#72358=ORIENTED_EDGE ( 'NONE', *, *, #38868, .T. ) ;
#72363=CARTESIAN_POINT ( 'NONE',  ( -1.407440972164865967, 1.192216805462484874, 0.3257083040380834293 ) ) ;
#72369=FACE_OUTER_BOUND ( 'NONE', #9169, .T. ) ;
#72375=CARTESIAN_POINT ( 'NONE',  ( -2.554262525012222174, 1.537401574803149984, 0.4744094488188970171 ) ) ;
#72402=CARTESIAN_POINT ( 'NONE',  ( -1.901964908973693635, 1.119136672863556559, -0.2244172274864991157 ) ) ;
#72432=CARTESIAN_POINT ( 'NONE',  ( 0.4744094488189052328, 1.546091976385118638, -2.170146923806634653 ) ) ;
#72433=CARTESIAN_POINT ( 'NONE',  ( -0.5314960629921122726, 2.559055118110236560, -3.937007874015763687 ) ) ;
#72439=ADVANCED_FACE ( 'NONE', ( #79200 ), #35855, .T. ) ;
#72444=VERTEX_POINT ( 'NONE', #39626 ) ;
#72450=CARTESIAN_POINT ( 'NONE',  ( 0.04809640131873983010, 1.065410365535384596, -1.583836855790661913 ) ) ;
#72473=CARTESIAN_POINT ( 'NONE',  ( 2.556891461833387336, 2.729656616209943376, -0.5314960629921260393 ) ) ;
#72478=PLANE ( 'NONE',  #67131 ) ;
#72501=CARTESIAN_POINT ( 'NONE',  ( -0.4677827689124922084, 0.03937007874015747977, -2.154527559055118946 ) ) ;
#72505=CARTESIAN_POINT ( 'NONE',  ( -0.4697171261336051673, 1.606100245667703819, 2.158884350236656591 ) ) ;
#72511=DIRECTION ( 'NONE',  ( 0.000000000000000000, 0.000000000000000000, -1.000000000000000000 ) ) ;
#72528=ADVANCED_FACE ( 'NONE', ( #64881 ), #26405, .F. ) ;
#72539=EDGE_CURVE ( 'NONE', #2386, #70474, #23761, .T. ) ;
#72549=CARTESIAN_POINT ( 'NONE',  ( -0.4359958488159647039, 1.724409448818897905, -2.094141031014960408 ) ) ;
#72571=DIRECTION ( 'NONE',  ( -0.000000000000000000, 1.000000000000000000, 0.000000000000000000 ) ) ;
#72573=CARTESIAN_POINT ( 'NONE',  ( -0.4359958488159582091, 1.724409448818897905, -3.937007874015763687 ) ) ;
#72576=CARTESIAN_POINT ( 'NONE',  ( 0.4744094488189112280, 1.569730808353063445, -3.908320185825790993 ) ) ;
#72599=CARTESIAN_POINT ( 'NONE',  ( -1.559171609364246924, 0.3937007874015748254, 0.4177787735906735578 ) ) ;
#72617=FACE_OUTER_BOUND ( 'NONE', #20157, .T. ) ;
#72620=CYLINDRICAL_SURFACE ( 'NONE', #75716, 3.937007874015748143 ) ;
#72646=ORIENTED_EDGE ( 'NONE', *, *, #45034, .F. ) ;
#72658=ADVANCED_FACE ( 'NONE', ( #35804 ), #80850, .T. ) ;
#72668=DIRECTION ( 'NONE',  ( 0.000000000000000000, -1.000000000000000000, 0.000000000000000000 ) ) ;
#72683=CARTESIAN_POINT ( 'NONE',  ( 0.5314960629921396951, 2.687614851728676424, -3.900966923095589234 ) ) ;
#72690=CARTESIAN_POINT ( 'NONE',  ( 1.923433685342916144, 1.142877263639046959, -0.2639061591570168175 ) ) ;
#72691=ADVANCED_FACE ( 'NONE', ( #55965 ), #74115, .F. ) ;
#72698=CARTESIAN_POINT ( 'NONE',  ( -0.4668652553835747621, 1.622068519643040219, 2.571961977011489875 ) ) ;
#72714=CARTESIAN_POINT ( 'NONE',  ( -0.4744094488188934089, 1.553403318890016482, -1.016821367227985329 ) ) ;
#72737=CARTESIAN_POINT ( 'NONE',  ( -3.869764100875850765, 2.739927440807262471, -0.5314960629921260393 ) ) ;
#72746=CARTESIAN_POINT ( 'NONE',  ( 3.846978723397335376, 2.751923335154144556, 0.5314960629921260393 ) ) ;
#72750=ORIENTED_EDGE ( 'NONE', *, *, #9628, .F. ) ;
#72766=ORIENTED_EDGE ( 'NONE', *, *, #80939, .T. ) ;
#72769=CARTESIAN_POINT ( 'NONE',  ( 2.554262525012303442, 1.528780496884629025, 0.4744094488188976277 ) ) ;
#72797=EDGE_CURVE ( 'NONE', #3191, #45375, #82879, .T. ) ;
#72829=DIRECTION ( 'NONE',  ( 0.000000000000000000, 0.000000000000000000, -1.000000000000000000 ) ) ;
#72836=ORIENTED_EDGE ( 'NONE', *, *, #77992, .T. ) ;
#72850=ORIENTED_EDGE ( 'NONE', *, *, #50355, .F. ) ;
#72854=ORIENTED_EDGE ( 'NONE', *, *, #21327, .F. ) ;
#72867=EDGE_CURVE ( 'NONE', #15345, #60855, #74532, .T. ) ;
#72870=VERTEX_POINT ( 'NONE', #3819 ) ;
#72873=VERTEX_POINT ( 'NONE', #10955 ) ;
#72899=CARTESIAN_POINT ( 'NONE',  ( 2.543486866223389153, 2.716535433070866645, 0.5314960629921260393 ) ) ;
#72908=DIRECTION ( 'NONE',  ( -0.000000000000000000, -1.000000000000000000, -0.000000000000000000 ) ) ;
#72915=EDGE_CURVE ( 'NONE', #43005, #32472, #18364, .T. ) ;
#72960=CARTESIAN_POINT ( 'NONE',  ( -0.4562720003150207426, 1.668198494846153457, -2.130121299646748234 ) ) ;
#72978=VERTEX_POINT ( 'NONE', #36612 ) ;
#72984=CARTESIAN_POINT ( 'NONE',  ( 3.900966923095589678, 2.755905511811024056, -0.5314960629921260393 ) ) ;
#72989=TOROIDAL_SURFACE ( 'NONE', #25920, 1.178877988035069047, 0.01968503937007873988 ) ;
#73001=ORIENTED_EDGE ( 'NONE', *, *, #67409, .F. ) ;
#73003=DIRECTION ( 'NONE',  ( 0.000000000000000000, 1.601283208593975810E-15, -1.000000000000000000 ) ) ;
#73008=AXIS2_PLACEMENT_3D ( 'NONE', #53870, #47561, #21075 ) ;
#73035=VERTEX_POINT ( 'NONE', #41291 ) ;
#73051=CARTESIAN_POINT ( 'NONE',  ( -0.4359958488159811907, 1.724409448818897905, 2.630268417803910186 ) ) ;
#73071=DIRECTION ( 'NONE',  ( -0.000000000000000000, -1.000000000000000000, -0.000000000000000000 ) ) ;
#73083=ORIENTED_EDGE ( 'NONE', *, *, #42797, .F. ) ;
#73084=DIRECTION ( 'NONE',  ( 0.000000000000000000, 0.000000000000000000, -1.000000000000000000 ) ) ;
#73088=DIRECTION ( 'NONE',  ( 0.000000000000000000, -1.000000000000000000, -0.000000000000000000 ) ) ;
#73090=CARTESIAN_POINT ( 'NONE',  ( 0.5314960629921371416, 2.755905511811024056, -3.184294706754629001 ) ) ;
#73098=CARTESIAN_POINT ( 'NONE',  ( 0.5314960629921393620, 2.755905511811024056, -3.826707563893390951 ) ) ;
#73099=ORIENTED_EDGE ( 'NONE', *, *, #41242, .F. ) ;
#73102=SHAPE_REPRESENTATION_RELATIONSHIP ( 'NONE' , 'NONE' ,  #7298, #79514 ) ;
#73104=CARTESIAN_POINT ( 'NONE',  ( 2.019766021329699512, 1.253539720428401560, -0.3811758253793051110 ) ) ;
#73105=EDGE_CURVE ( 'NONE', #44550, #712, #75408, .T. ) ;
#73112=CARTESIAN_POINT ( 'NONE',  ( 2.170146923806595129, 1.537401574803149984, 0.4744094488188975722 ) ) ;
#73118=CIRCLE ( 'NONE', #34181, 0.09842519685039351207 ) ;
#73122=UNCERTAINTY_MEASURE_WITH_UNIT (LENGTH_MEASURE( 1.000000000000000082E-05 ), #36337, 'distance_accuracy_value', 'NONE');
#73131=DIRECTION ( 'NONE',  ( 1.000000000000000000, -0.000000000000000000, -0.000000000000000000 ) ) ;
#73138=DIRECTION ( 'NONE',  ( 0.000000000000000000, -1.000000000000000000, 0.000000000000000000 ) ) ;
#73162=CARTESIAN_POINT ( 'NONE',  ( -0.5314960629921349211, 2.716535433070866645, 2.543486866223387377 ) ) ;
#73171=AXIS2_PLACEMENT_3D ( 'NONE', #22177, #9964, #29317 ) ;
#73181=ORIENTED_EDGE ( 'NONE', *, *, #49228, .F. ) ;
#73186=CARTESIAN_POINT ( 'NONE',  ( 2.860656214895214156, 1.077434660671929167, 0.1173752429317640178 ) ) ;
#73201=ORIENTED_EDGE ( 'NONE', *, *, #58706, .F. ) ;
#73227=CARTESIAN_POINT ( 'NONE',  ( -2.167269426034507784, 1.502969453419624513, -0.4732359647714766693 ) ) ;
#73241=ADVANCED_FACE ( 'NONE', ( #72312 ), #71892, .F. ) ;
#73252=AXIS2_PLACEMENT_3D ( 'NONE', #60763, #2701, #54442 ) ;
#73256=ORIENTED_EDGE ( 'NONE', *, *, #57249, .F. ) ;
#73266=DIRECTION ( 'NONE',  ( 0.000000000000000000, 0.000000000000000000, 1.000000000000000000 ) ) ;
#73280=CARTESIAN_POINT ( 'NONE',  ( 0.03820975525947114398, 1.064507315957821998, -1.600359255881266041 ) ) ;
#73289=ORIENTED_EDGE ( 'NONE', *, *, #46574, .T. ) ;
#73302=EDGE_CURVE ( 'NONE', #9114, #29875, #39901, .T. ) ;
#73312=AXIS2_PLACEMENT_3D ( 'NONE', #12771, #43078, #76740 ) ;
#73328=CARTESIAN_POINT ( 'NONE',  ( -0.1090865357759267934, 1.075440515114686191, -1.116837428146558064 ) ) ;
#73338=B_SPLINE_CURVE_WITH_KNOTS ( 'NONE', 3,
 ( #75544, #76365, #81864, #57393 ),
 .UNSPECIFIED., .F., .F.,
 ( 4, 4 ),
 ( 0.1208891233417057898, 0.1223338575624300234 ),
 .UNSPECIFIED. ) ;
#73363=CARTESIAN_POINT ( 'NONE',  ( 2.167714792466672868, 1.572145545125847033, -0.4734416007054413345 ) ) ;
#73373=FACE_OUTER_BOUND ( 'NONE', #5171, .T. ) ;
#73388=EDGE_CURVE ( 'NONE', #62716, #53039, #58662, .T. ) ;
#73395=ADVANCED_FACE ( 'NONE', ( #8333 ), #33999, .F. ) ;
#73402=ORIENTED_EDGE ( 'NONE', *, *, #72915, .T. ) ;
#73403=ORIENTED_EDGE ( 'NONE', *, *, #9959, .T. ) ;
#73406=VECTOR ( 'NONE', #51660, 39.37007874015748143 ) ;
#73408=CARTESIAN_POINT ( 'NONE',  ( 0.4562955581495489743, 1.668131542012062596, 2.130163876373972531 ) ) ;
#73411=DIRECTION ( 'NONE',  ( -0.8660254037844433705, 0.000000000000000000, 0.4999999999999920064 ) ) ;
#73418=ORIENTED_EDGE ( 'NONE', *, *, #34082, .F. ) ;
#73426=AXIS2_PLACEMENT_3D ( 'NONE', #31360, #22994, #62122 ) ;
#73434=DIRECTION ( 'NONE',  ( 0.000000000000000000, 0.000000000000000000, 1.000000000000000000 ) ) ;
#73442=B_SPLINE_CURVE_WITH_KNOTS ( 'NONE', 3,
 ( #76304, #63242, #51419, #51843 ),
 .UNSPECIFIED., .F., .F.,
 ( 4, 4 ),
 ( 0.05218731980467040954, 0.05362944292333594182 ),
 .UNSPECIFIED. ) ;
#73444=DIRECTION ( 'NONE',  ( -5.329070518200751394E-15, 0.000000000000000000, -1.000000000000000000 ) ) ;
#73455=CARTESIAN_POINT ( 'NONE',  ( 0.2240801135442004322, 1.118954560528815589, 1.901799418834396738 ) ) ;
#73458=DIRECTION ( 'NONE',  ( 8.659560562354908206E-17, -0.7071067811865496822, 0.7071067811865454633 ) ) ;
#73471=VECTOR ( 'NONE', #58695, 39.37007874015748143 ) ;
#73491=ORIENTED_EDGE ( 'NONE', *, *, #60347, .T. ) ;
#73493=ORIENTED_EDGE ( 'NONE', *, *, #66096, .F. ) ;
#73509=ORIENTED_EDGE ( 'NONE', *, *, #51081, .F. ) ;
#73516=CARTESIAN_POINT ( 'NONE',  ( -0.9285414500055709786, 1.724409448818897905, 0.6299212598425196763 ) ) ;
#73532=CARTESIAN_POINT ( 'NONE',  ( 1.947231901457292969, 1.169463170161823440, -0.3010181502270611320 ) ) ;
#73578=CARTESIAN_POINT ( 'NONE',  ( 3.937007874015748143, 1.537401574803149984, -0.4744094488188970171 ) ) ;
#73585=CARTESIAN_POINT ( 'NONE',  ( -3.910253683044872197, 1.664255196667159042, 0.4582455874901649184 ) ) ;
#73586=CONICAL_SURFACE ( 'NONE', #74904, 0.09842519685039351207, 1.029744258676652091 ) ;
#73594=EDGE_CURVE ( 'NONE', #25136, #23894, #45097, .T. ) ;
#73608=ORIENTED_EDGE ( 'NONE', *, *, #28505, .T. ) ;
#73610=ORIENTED_EDGE ( 'NONE', *, *, #38141, .F. ) ;
#73613=CARTESIAN_POINT ( 'NONE',  ( -1.436918669920151492, 1.161451126500848918, 0.2894072871544302039 ) ) ;
#73620=FACE_OUTER_BOUND ( 'NONE', #76179, .T. ) ;
#73624=ORIENTED_EDGE ( 'NONE', *, *, #81513, .T. ) ;
#73626=CYLINDRICAL_SURFACE ( 'NONE', #77548, 0.4744094488188972947 ) ;
#73654=CARTESIAN_POINT ( 'NONE',  ( 0.5314960629920858493, 2.755905511811024056, 3.831929248781932973 ) ) ;
#73680=DIRECTION ( 'NONE',  ( 0.000000000000000000, -1.000000000000000000, 0.000000000000000000 ) ) ;
#73684=DIRECTION ( 'NONE',  ( -0.000000000000000000, -1.000000000000000000, -0.000000000000000000 ) ) ;
#73686=FACE_OUTER_BOUND ( 'NONE', #42320, .T. ) ;
#73689=DIRECTION ( 'NONE',  ( 0.000000000000000000, 1.000000000000000000, -0.000000000000000000 ) ) ;
#73702=CARTESIAN_POINT ( 'NONE',  ( -0.4470293165555038195, 1.696956328257585911, -2.611628156437945325 ) ) ;
#73707=DIRECTION ( 'NONE',  ( 0.000000000000000000, 0.000000000000000000, 1.000000000000000000 ) ) ;
#73710=ORIENTED_EDGE ( 'NONE', *, *, #48095, .T. ) ;
#73714=AXIS2_PLACEMENT_3D ( 'NONE', #44032, #42082, #82765 ) ;
#73728=EDGE_CURVE ( 'NONE', #47922, #55882, #78404, .T. ) ;
#73734=CARTESIAN_POINT ( 'NONE',  ( 3.912496512833623985, 1.354998764345328510, 0.4387572725319323075 ) ) ;
#73744=PLANE ( 'NONE',  #74135 ) ;
#73751=DIRECTION ( 'NONE',  ( 0.000000000000000000, 0.000000000000000000, -1.000000000000000000 ) ) ;
#73781=CARTESIAN_POINT ( 'NONE',  ( -1.633215945612316311, 1.138418561298297771, 0.2566901766734876467 ) ) ;
#73783=PLANE ( 'NONE',  #52692 ) ;
#73785=CARTESIAN_POINT ( 'NONE',  ( 2.149112266099340918, 1.629972608277047819, -0.4653577321740515194 ) ) ;
#73794=LINE ( 'NONE', #54406, #54879 ) ;
#73819=DIRECTION ( 'NONE',  ( -3.491481338843132961E-15, -0.000000000000000000, 1.000000000000000000 ) ) ;
#73821=DIRECTION ( 'NONE',  ( -0.000000000000000000, 1.000000000000000000, -0.000000000000000000 ) ) ;
#73828=PLANE ( 'NONE',  #27690 ) ;
#73829=CARTESIAN_POINT ( 'NONE',  ( -0.4574222058066962360, 1.664230899554594467, 3.910347713755335963 ) ) ;
#73838=CARTESIAN_POINT ( 'NONE',  ( -1.122045408380372367, 1.062996467714767634, 0.03161692930310931043 ) ) ;
#73840=CARTESIAN_POINT ( 'NONE',  ( -1.895394334970792016, 2.755905511811024056, -0.5314960629921260393 ) ) ;
#73846=CARTESIAN_POINT ( 'NONE',  ( -0.9285414500055713116, 0.000000000000000000, 0.6299212598425196763 ) ) ;
#73853=CARTESIAN_POINT ( 'NONE',  ( 2.620894764083865347, 1.710972922415818331, -0.4417590601942915640 ) ) ;
#73873=CARTESIAN_POINT ( 'NONE',  ( 0.4672469119858274067, 1.453788974454132132, 2.153180749494128854 ) ) ;
#73876=ADVANCED_FACE ( 'NONE', ( #75622 ), #9991, .T. ) ;
#73877=FACE_OUTER_BOUND ( 'NONE', #22354, .T. ) ;
#73892=DIRECTION ( 'NONE',  ( -0.000000000000000000, 1.000000000000000000, -0.000000000000000000 ) ) ;
#73904=EDGE_LOOP ( 'NONE', ( #29040, #55259, #25751, #42926 ) ) ;
#73905=ORIENTED_EDGE ( 'NONE', *, *, #70014, .T. ) ;
#73929=CARTESIAN_POINT ( 'NONE',  ( 1.024290093949184799, 1.664773289199195982, -0.4581164262379300856 ) ) ;
#73975=CARTESIAN_POINT ( 'NONE',  ( 0.000000000000000000, 2.559055118110236560, 0.000000000000000000 ) ) ;
#73981=CARTESIAN_POINT ( 'NONE',  ( 3.937007874015748143, 1.537401574803149984, 2.901595197523589142E-16 ) ) ;
#73986=AXIS2_PLACEMENT_3D ( 'NONE', #27874, #78821, #34612 ) ;
#73999=EDGE_LOOP ( 'NONE', ( #31958, #32761, #11261, #20255, #38504, #40670 ) ) ;
#74001=EDGE_LOOP ( 'NONE', ( #70788, #7535, #1043 ) ) ;
#74015=VERTEX_POINT ( 'NONE', #77263 ) ;
#74018=CARTESIAN_POINT ( 'NONE',  ( -1.382164990278195615, 1.299212598425196985, 0.4102808022082835571 ) ) ;
#74024=DIRECTION ( 'NONE',  ( 0.000000000000000000, 1.000000000000000000, 0.000000000000000000 ) ) ;
#74031=LINE ( 'NONE', #16794, #27792 ) ;
#74052=CIRCLE ( 'NONE', #65935, 1.122047244094488194 ) ;
#74054=DIRECTION ( 'NONE',  ( 1.408710688920637755E-15, -1.000000000000000000, 4.918487082195260922E-30 ) ) ;
#74057=ADVANCED_FACE ( 'NONE', ( #50742 ), #45254, .F. ) ;
#74060=DIRECTION ( 'NONE',  ( -0.000000000000000000, -1.000000000000000000, 0.000000000000000000 ) ) ;
#74091=DIRECTION ( 'NONE',  ( 0.000000000000000000, 0.000000000000000000, 1.000000000000000000 ) ) ;
#74094=DIRECTION ( 'NONE',  ( 0.000000000000000000, 0.000000000000000000, 1.000000000000000000 ) ) ;
#74110=DIRECTION ( 'NONE',  ( -3.491481338843132961E-15, -0.000000000000000000, 1.000000000000000000 ) ) ;
#74115=CYLINDRICAL_SURFACE ( 'NONE', #45182, 0.2165354330708660069 ) ;
#74135=AXIS2_PLACEMENT_3D ( 'NONE', #4257, #74567, #48043 ) ;
#74150=CARTESIAN_POINT ( 'NONE',  ( 0.5314960629921396951, 2.755905511811024056, -3.937007874015760578 ) ) ;
#74172=CONICAL_SURFACE ( 'NONE', #9637, 2.637795275590551380, 0.7853981633974500554 ) ;
#74186=ADVANCED_FACE ( 'NONE', ( #71365 ), #12052, .T. ) ;
#74192=FACE_OUTER_BOUND ( 'NONE', #39829, .T. ) ;
#74198=ORIENTED_EDGE ( 'NONE', *, *, #47097, .T. ) ;
#74208=B_SPLINE_CURVE_WITH_KNOTS ( 'NONE', 3,
 ( #23321, #17035, #81419, #72306, #2011, #15061, #14653, #68373, #55299, #65989, #8327, #33993, #59655, #40717, #27674, #53340, #21367, #66402 ),
 .UNSPECIFIED., .F., .F.,
 ( 4, 2, 2, 2, 2, 2, 2, 2, 4 ),
 ( 0.001226984380451624388, 0.003469327704077891823, 0.004590499365891025432, 0.005151085196797592670, 0.005711671027704158174, 0.006272256858610725412, 0.006832842689517291783, 0.007954014351330434066, 0.01019635767495674639 ),
 .UNSPECIFIED. ) ;
#74229=CARTESIAN_POINT ( 'NONE',  ( -0.3230994083235659842, 1.189706270649608655, -2.759390867997893348 ) ) ;
#74231=CIRCLE ( 'NONE', #79587, 0.1190944881889763746 ) ;
#74232=CARTESIAN_POINT ( 'NONE',  ( 1.374111565972423831E-16, 0.000000000000000000, -1.122047244094488194 ) ) ;
#74238=DIRECTION ( 'NONE',  ( 0.000000000000000000, -1.000000000000000000, 0.000000000000000000 ) ) ;
#74241=CARTESIAN_POINT ( 'NONE',  ( -0.4614848114146354319, 1.648560354533844308, 3.909868722774259453 ) ) ;
#74250=CARTESIAN_POINT ( 'NONE',  ( -1.067249829279471429, 1.213052584328227157, 0.3465489493959020839 ) ) ;
#74256=CARTESIAN_POINT ( 'NONE',  ( -0.3149606299212733274, 2.165354330708661568, 3.924389226575467404 ) ) ;
#74258=LINE ( 'NONE', #16599, #69138 ) ;
#74285=CARTESIAN_POINT ( 'NONE',  ( 0.03430998917087475092, 1.064156075168071869, 1.851472435485761237 ) ) ;
#74290=ORIENTED_EDGE ( 'NONE', *, *, #8460, .T. ) ;
#74316=EDGE_LOOP ( 'NONE', ( #59194, #48916, #65899, #65303, #4613, #15754, #65517, #79932, #10860, #43840, #16218, #79930, #61559, #47598 ) ) ;
#74322=CARTESIAN_POINT ( 'NONE',  ( 0.3149606299212737159, 2.165354330708661568, -3.937007874015761022 ) ) ;
#74334=ORIENTED_EDGE ( 'NONE', *, *, #37360, .F. ) ;
#74344=AXIS2_PLACEMENT_3D ( 'NONE', #9068, #34739, #22100 ) ;
#74348=ADVANCED_FACE ( 'NONE', ( #5718 ), #72989, .F. ) ;
#74364=LINE ( 'NONE', #11625, #7444 ) ;
#74380=CARTESIAN_POINT ( 'NONE',  ( -2.570293878819217337, 2.742780005561834322, 0.5314960629921260393 ) ) ;
#74389=ADVANCED_FACE ( 'NONE', ( #70951 ), #34002, .F. ) ;
#74428=EDGE_LOOP ( 'NONE', ( #71910, #81894, #19128, #42398 ) ) ;
#74433=CARTESIAN_POINT ( 'NONE',  ( -1.559171609364246924, 0.000000000000000000, 0.7327394035119333404 ) ) ;
#74440=DIRECTION ( 'NONE',  ( 0.000000000000000000, 1.000000000000000000, -0.000000000000000000 ) ) ;
#74441=CARTESIAN_POINT ( 'NONE',  ( 0.3149606299212184268, 2.559055118110236560, 3.937007874015792552 ) ) ;
#74446=ORIENTED_EDGE ( 'NONE', *, *, #1221, .T. ) ;
#74448=CARTESIAN_POINT ( 'NONE',  ( 0.5314960629920995050, 2.729661064330338061, 2.530077726415326023 ) ) ;
#74455=LINE ( 'NONE', #34597, #10218 ) ;
#74471=CARTESIAN_POINT ( 'NONE',  ( -0.5314960629921123836, 2.677165354330708791, -3.900966923095591454 ) ) ;
#74476=CARTESIAN_POINT ( 'NONE',  ( -2.139067083128550983, 1.422987107291908249, 0.4606739315415592229 ) ) ;
#74487=B_SPLINE_CURVE_WITH_KNOTS ( 'NONE', 3,
 ( #43255, #10483, #36136, #4149, #82010, #29814, #5388, #23919, #61809, #75280, #68543, #49169, #31049, #56719, #10884, #11302, #62638, #42850, #4982, #82416, #6622, #64704, #45745, #63867, #39445, #26817 ),
 .UNSPECIFIED., .F., .F.,
 ( 4, 2, 2, 2, 2, 2, 2, 2, 2, 2, 2, 2, 4 ),
 ( 0.01885842312717905811, 0.02003652323609797156, 0.02121462334501688501, 0.02357082356285470845, 0.02474892367177362190, 0.02592702378069253535, 0.02828322399853035532, 0.03063942421636817875, 0.03181752432528708874, 0.03299562443420599872, 0.03535182465204379787, 0.03652992476096270091, 0.03770802486988160396 ),
 .UNSPECIFIED. ) ;
#74496=FACE_OUTER_BOUND ( 'NONE', #3209, .T. ) ;
#74504=AXIS2_PLACEMENT_3D ( 'NONE', #28044, #27627, #15860 ) ;
#74518=VECTOR ( 'NONE', #81239, 39.37007874015748143 ) ;
#74520=ORIENTED_EDGE ( 'NONE', *, *, #17653, .T. ) ;
#74532=LINE ( 'NONE', #61471, #61370 ) ;
#74567=DIRECTION ( 'NONE',  ( 1.000000000000000000, 0.000000000000000000, 1.047444401652940007E-14 ) ) ;
#74575=CARTESIAN_POINT ( 'NONE',  ( -2.557140022784271327, 1.502969453419624513, 0.4732359647714760587 ) ) ;
#74585=CIRCLE ( 'NONE', #32857, 3.937007874015748143 ) ;
#74592=CARTESIAN_POINT ( 'NONE',  ( -0.03443470937339819515, 1.064243487142144673, -1.633358474390059989 ) ) ;
#74608=CARTESIAN_POINT ( 'NONE',  ( 1.141392835773559211, 1.299212598425196985, 1.141392835773562764 ) ) ;
#74609=CARTESIAN_POINT ( 'NONE',  ( -0.6299212598425059095, 1.724409448818897905, -3.937007874015764131 ) ) ;
#74617=VERTEX_POINT ( 'NONE', #20018 ) ;
#74622=CARTESIAN_POINT ( 'NONE',  ( 2.142213561789872767, 0.02617651024168201127, 0.4623158380715620130 ) ) ;
#74639=VECTOR ( 'NONE', #34692, 39.37007874015748143 ) ;
#74648=DIRECTION ( 'NONE',  ( 0.000000000000000000, 0.000000000000000000, -1.000000000000000000 ) ) ;
#74650=FACE_OUTER_BOUND ( 'NONE', #2045, .T. ) ;
#74653=VERTEX_POINT ( 'NONE', #27156 ) ;
#74671=DIRECTION ( 'NONE',  ( 0.000000000000000000, -1.000000000000000000, -1.734723475976808327E-16 ) ) ;
#74692=AXIS2_PLACEMENT_3D ( 'NONE', #74441, #53405, #61796 ) ;
#74703=CARTESIAN_POINT ( 'NONE',  ( 0.3013144171194340193, 1.169708940200703040, 1.947449872764505541 ) ) ;
#74707=ORIENTED_EDGE ( 'NONE', *, *, #302, .F. ) ;
#74731=CIRCLE ( 'NONE', #80151, 0.3149606299212597826 ) ;
#74751=DIRECTION ( 'NONE',  ( -0.000000000000000000, -1.000000000000000000, -0.000000000000000000 ) ) ;
#74752=AXIS2_PLACEMENT_3D ( 'NONE', #50700, #38494, #1046 ) ;
#74757=CARTESIAN_POINT ( 'NONE',  ( 0.1273213304869930951, 0.2755905511811023723, -1.680969278250197707 ) ) ;
#74766=ORIENTED_EDGE ( 'NONE', *, *, #57094, .F. ) ;
#74769=CARTESIAN_POINT ( 'NONE',  ( 0.4177787735907000366, 1.299212598425196985, -1.559171609364239375 ) ) ;
#74791=VECTOR ( 'NONE', #67664, 39.37007874015748143 ) ;
#74793=AXIS2_PLACEMENT_3D ( 'NONE', #41828, #79327, #74671 ) ;
#74795=ADVANCED_FACE ( 'NONE', ( #1092 ), #33484, .F. ) ;
#74801=CARTESIAN_POINT ( 'NONE',  ( -3.881246834694716874, 2.729333734409945755, 0.5314960629921260393 ) ) ;
#74807=B_SPLINE_CURVE_WITH_KNOTS ( 'NONE', 3,
 ( #72501, #14850, #66191, #8527 ),
 .UNSPECIFIED., .F., .F.,
 ( 4, 4 ),
 ( 2.857347768991906607E-07, 0.001436604392377180406 ),
 .UNSPECIFIED. ) ;
#74813=FACE_OUTER_BOUND ( 'NONE', #46143, .T. ) ;
#74822=B_SPLINE_CURVE_WITH_KNOTS ( 'NONE', 3,
 ( #60728, #22843, #54827, #48502, #28744, #14887, #46845, #53990, #53574, #34235, #8566, #47261, #53153, #40547 ),
 .UNSPECIFIED., .F., .F.,
 ( 4, 2, 2, 2, 2, 2, 4 ),
 ( 0.000000000000000000, 0.0003923887041693346835, 0.0007847774083386693670, 0.001177166112508004105, 0.001569554816677338734, 0.002354332225016037266, 0.003139109633354736015 ),
 .UNSPECIFIED. ) ;
#74831=ADVANCED_FACE ( 'NONE', ( #72617 ), #71784, .F. ) ;
#74834=EDGE_LOOP ( 'NONE', ( #55863, #19753, #16036, #33702 ) ) ;
#74844=EDGE_CURVE ( 'NONE', #48126, #65535, #59977, .T. ) ;
#74849=ORIENTED_EDGE ( 'NONE', *, *, #13007, .T. ) ;
#74860=CARTESIAN_POINT ( 'NONE',  ( 0.4735861421683033035, 1.569672585540540899, 1.017206702362611903 ) ) ;
#74865=VERTEX_POINT ( 'NONE', #52820 ) ;
#74868=ORIENTED_EDGE ( 'NONE', *, *, #68011, .T. ) ;
#74892=CARTESIAN_POINT ( 'NONE',  ( -2.058019426306472166, 1.301092492065855089, 0.4123476441529934644 ) ) ;
#74904=AXIS2_PLACEMENT_3D ( 'NONE', #56421, #25256, #24436 ) ;
#74909=VECTOR ( 'NONE', #13476, 39.37007874015748143 ) ;
#74912=DIRECTION ( 'NONE',  ( 0.000000000000000000, 1.000000000000000000, 0.000000000000000000 ) ) ;
#74926=CARTESIAN_POINT ( 'NONE',  ( 0.000000000000000000, 2.755905511811024056, 0.000000000000000000 ) ) ;
#74929=FACE_BOUND ( 'NONE', #80561, .T. ) ;
#74942=DIRECTION ( 'NONE',  ( -0.000000000000000000, -1.000000000000000000, -0.000000000000000000 ) ) ;
#74972=CIRCLE ( 'NONE', #58784, 0.1771653543307085410 ) ;
#74981=LINE ( 'NONE', #24021, #12288 ) ;
#74985=CARTESIAN_POINT ( 'NONE',  ( 0.4581426849250296862, 1.664615899758173034, -1.024278008493450409 ) ) ;
#74988=CARTESIAN_POINT ( 'NONE',  ( -2.704370107879186413, 1.253873987468420603, 0.3814095263789963330 ) ) ;
#74991=DIRECTION ( 'NONE',  ( 0.000000000000000000, 1.000000000000000000, 0.000000000000000000 ) ) ;
#75000=CARTESIAN_POINT ( 'NONE',  ( 0.4620341399816233485, 1.428627056473853241, -1.022509594724332116 ) ) ;
#75004=CARTESIAN_POINT ( 'NONE',  ( 0.08529443231574072859, 1.070420337342308459, -1.857273270772795026 ) ) ;
#75021=CARTESIAN_POINT ( 'NONE',  ( -1.661807552036326463, 1.149545036241496510, 0.2732228506959576420 ) ) ;
#75022=CARTESIAN_POINT ( 'NONE',  ( -0.5314960629921349211, 2.729656497683583538, 2.556891340746902053 ) ) ;
#75025=AXIS2_PLACEMENT_3D ( 'NONE', #7615, #58948, #1306 ) ;
#75035=DIRECTION ( 'NONE',  ( -1.000000000000000000, -8.673617379884021667E-16, 0.000000000000000000 ) ) ;
#75066=PLANE ( 'NONE',  #8192 ) ;
#75067=DIRECTION ( 'NONE',  ( 0.000000000000000000, -1.408710688920637755E-15, -1.000000000000000000 ) ) ;
#75070=LENGTH_MEASURE_WITH_UNIT ( LENGTH_MEASURE( 0.02539999999999999897 ), #62419 );
#75092=DIRECTION ( 'NONE',  ( 0.000000000000000000, 1.000000000000000000, -0.000000000000000000 ) ) ;
#75100=ADVANCED_FACE ( 'NONE', ( #8644 ), #62232, .F. ) ;
#75101=DIRECTION ( 'NONE',  ( 0.000000000000000000, 1.000000000000000000, 0.000000000000000000 ) ) ;
#75116=CARTESIAN_POINT ( 'NONE',  ( 0.1340670299283531486, 1.082026165109806648, 1.867989472054414346 ) ) ;
#75120=EDGE_LOOP ( 'NONE', ( #54954, #40036, #4143, #44461 ) ) ;
#75124=DIRECTION ( 'NONE',  ( 0.000000000000000000, 1.000000000000000000, 0.000000000000000000 ) ) ;
#75132=CARTESIAN_POINT ( 'NONE',  ( -0.4713486786305523535, 1.475001655854108584, 1.018266755655268474 ) ) ;
#75161=VERTEX_POINT ( 'NONE', #35143 ) ;
#75167=DIRECTION ( 'NONE',  ( 0.000000000000000000, 0.000000000000000000, -1.000000000000000000 ) ) ;
#75169=CARTESIAN_POINT ( 'NONE',  ( 0.000000000000000000, 2.755905511811024056, -3.937007874015748143 ) ) ;
#75170=DIRECTION ( 'NONE',  ( -3.491481338843132961E-15, 0.000000000000000000, 1.000000000000000000 ) ) ;
#75180=CARTESIAN_POINT ( 'NONE',  ( 1.403614904275686858E-14, 1.537401574803149984, -3.937007874015761910 ) ) ;
#75249=EDGE_CURVE ( 'NONE', #62570, #63201, #59290, .T. ) ;
#75252=ORIENTED_EDGE ( 'NONE', *, *, #33485, .F. ) ;
#75254=ORIENTED_EDGE ( 'NONE', *, *, #19393, .T. ) ;
#75261=DIRECTION ( 'NONE',  ( 0.000000000000000000, 0.000000000000000000, -1.000000000000000000 ) ) ;
#75265=DIRECTION ( 'NONE',  ( -0.000000000000000000, -1.000000000000000000, -0.000000000000000000 ) ) ;
#75271=ORIENTED_EDGE ( 'NONE', *, *, #39342, .T. ) ;
#75280=CARTESIAN_POINT ( 'NONE',  ( -0.2376021588233629689, 1.126485847204533597, 3.929855605829966514 ) ) ;
#75315=CARTESIAN_POINT ( 'NONE',  ( -3.923617024849349377, 1.191103570792281241, 0.3246236190342044470 ) ) ;
#75320=ORIENTED_EDGE ( 'NONE', *, *, #81028, .F. ) ;
#75321=EDGE_CURVE ( 'NONE', #32589, #19658, #67140, .T. ) ;
#75347=CARTESIAN_POINT ( 'NONE',  ( 0.4477342634306737956, 1.379855024864605539, -2.610352282803159785 ) ) ;
#75370=B_SPLINE_CURVE_WITH_KNOTS ( 'NONE', 3,
 ( #3314, #55461, #74860, #29800, #23074, #80760, #15543, #17202, #66890, #23488 ),
 .UNSPECIFIED., .F., .F.,
 ( 4, 2, 2, 2, 4 ),
 ( 0.01907194592498655597, 0.02029034601373087832, 0.02150874610247520413, 0.02272714619121952648, 0.02394554627996384882 ),
 .UNSPECIFIED. ) ;
#75386=AXIS2_PLACEMENT_3D ( 'NONE', #16856, #42491, #66955 ) ;
#75387=CARTESIAN_POINT ( 'NONE',  ( 0.4359958488159758616, 1.724409448818897905, -1.033875059083675163 ) ) ;
#75390=CARTESIAN_POINT ( 'NONE',  ( -2.619510771202522292, 1.365902157108380477, -0.4425616331406683202 ) ) ;
#75399=DIRECTION ( 'NONE',  ( 0.000000000000000000, 1.000000000000000000, 0.000000000000000000 ) ) ;
#75408=B_SPLINE_CURVE_WITH_KNOTS ( 'NONE', 3,
 ( #4628, #16878, #22348, #9720, #61056, #9309, #3406, #34979, #60643, #35391, #48008, #29069, #80445, #22755, #48416, #63120, #57615, #63531, #5862, #43323, #69023, #11374, #75347, #25216, #50470, #37446, #38682, #17695, #37031, #62713 ),
 .UNSPECIFIED., .F., .F.,
 ( 4, 2, 2, 2, 2, 2, 2, 2, 2, 2, 2, 2, 2, 2, 4 ),
 ( 0.02630788966047398897, 0.02761938857346088114, 0.02893088748644776984, 0.03024238639943466200, 0.03155388531242155070, 0.03417688313839533504, 0.03548838205138224455, 0.03679988096436914713, 0.03942287879034296616, 0.04073437770332988261, 0.04204587661631679907, 0.04335737552930371552, 0.04466887444229063198, 0.04598037335527754843, 0.04729187226826446488 ),
 .UNSPECIFIED. ) ;
#75415=CARTESIAN_POINT ( 'NONE',  ( 1.895394334970792016, 2.755905511811024056, -0.5314960629921260393 ) ) ;
#75418=ADVANCED_FACE ( 'NONE', ( #36382 ), #20605, .F. ) ;
#75424=VECTOR ( 'NONE', #64753, 39.37007874015748143 ) ;
#75428=EDGE_CURVE ( 'NONE', #44792, #10316, #17905, .T. ) ;
#75439=ORIENTED_EDGE ( 'NONE', *, *, #6477, .T. ) ;
#75444=CARTESIAN_POINT ( 'NONE',  ( -0.9881811337016640495, 2.755905511811024056, 0.5314960629921260393 ) ) ;
#75446=VECTOR ( 'NONE', #48450, 39.37007874015748143 ) ;
#75455=CARTESIAN_POINT ( 'NONE',  ( -3.937007874015748143, 1.724409448818897905, -0.4359958488159722534 ) ) ;
#75456=DIRECTION ( 'NONE',  ( 0.000000000000000000, 1.000000000000000000, 0.000000000000000000 ) ) ;
#75475=ORIENTED_EDGE ( 'NONE', *, *, #3774, .T. ) ;
#75476=EDGE_LOOP ( 'NONE', ( #36538, #6250, #12909, #33490, #35789, #24399, #74290, #79510, #13428, #15640, #55438, #5632, #56070, #58353, #38996, #52205, #18005, #15517, #38251, #72257, #12003, #44660, #53781, #73402, #4111, #50788, #80451, #46990, #65125, #16961, #68034, #79000, #53181, #10256, #7791, #15096 ) ) ;
#75479=CARTESIAN_POINT ( 'NONE',  ( -2.543486866223389153, 2.716535433070866645, -0.5314960629921260393 ) ) ;
#75484=ADVANCED_FACE ( 'NONE', ( #38440 ), #77168, .T. ) ;
#75515=CARTESIAN_POINT ( 'NONE',  ( 2.565964038698667515, 1.605872332714551876, 0.4695140184743388789 ) ) ;
#75543=CARTESIAN_POINT ( 'NONE',  ( 0.000000000000000000, 1.929133858267716661, 1.850393700787401619 ) ) ;
#75544=CARTESIAN_POINT ( 'NONE',  ( -1.813482582612293559, 2.755905511811024056, -0.5314960629921260393 ) ) ;
#75549=AXIS2_PLACEMENT_3D ( 'NONE', #49703, #75399, #37491 ) ;
#75563=CARTESIAN_POINT ( 'NONE',  ( 2.170146923806634653, 1.537401574803149984, -0.4744094488188970171 ) ) ;
#75580=DIRECTION ( 'NONE',  ( -0.000000000000000000, -1.000000000000000000, -0.000000000000000000 ) ) ;
#75582=CARTESIAN_POINT ( 'NONE',  ( 0.4177787735907000366, 0.3937007874015747699, -1.559171609364239375 ) ) ;
#75585=EDGE_CURVE ( 'NONE', #82661, #36021, #43501, .T. ) ;
#75601=PLANE ( 'NONE',  #82822 ) ;
#75610=AXIS2_PLACEMENT_3D ( 'NONE', #32968, #21588, #26658 ) ;
#75622=FACE_OUTER_BOUND ( 'NONE', #65943, .T. ) ;
#75638=CARTESIAN_POINT ( 'NONE',  ( 0.2423360639762433821, 1.129538687396121954, -1.530894784087906357 ) ) ;
#75642=LINE ( 'NONE', #49533, #78935 ) ;
#75667=ORIENTED_EDGE ( 'NONE', *, *, #18320, .T. ) ;
#75677=LINE ( 'NONE', #4966, #44434 ) ;
#75686=ORIENTED_EDGE ( 'NONE', *, *, #41641, .F. ) ;
#75692=CARTESIAN_POINT ( 'NONE',  ( 0.5314960629920921775, 2.716535433070866645, 3.224202737261820939 ) ) ;
#75716=AXIS2_PLACEMENT_3D ( 'NONE', #1095, #26746, #27582 ) ;
#75730=CARTESIAN_POINT ( 'NONE',  ( 0.4177787735907000366, 0.3937007874015747699, -1.361336963694947944 ) ) ;
#75741=FACE_OUTER_BOUND ( 'NONE', #28773, .T. ) ;
#75749=VERTEX_POINT ( 'NONE', #30884 ) ;
#75794=DIRECTION ( 'NONE',  ( 0.000000000000000000, 1.000000000000000000, -0.000000000000000000 ) ) ;
#75796=DIRECTION ( 'NONE',  ( 1.000000000000000000, -0.000000000000000000, -0.000000000000000000 ) ) ;
#75800=CARTESIAN_POINT ( 'NONE',  ( -2.750540364621139933, 1.199841186584425845, 0.3336616047370347671 ) ) ;
#75806=EDGE_CURVE ( 'NONE', #41865, #29189, #53159, .T. ) ;
#75808=CARTESIAN_POINT ( 'NONE',  ( 2.362204724409448620, 1.724409448818900570, -0.5118110236220390075 ) ) ;
#75814=CARTESIAN_POINT ( 'NONE',  ( 0.4111343648323678157, 1.298683528505548468, -1.044172509125263160 ) ) ;
#75816=VECTOR ( 'NONE', #30112, 39.37007874015748143 ) ;
#75818=EDGE_CURVE ( 'NONE', #11040, #80330, #66265, .T. ) ;
#75819=CARTESIAN_POINT ( 'NONE',  ( 0.4698482617964849783, 1.469690627553814410, -2.159191069290731679 ) ) ;
#75824=ADVANCED_FACE ( 'NONE', ( #56839 ), #11009, .F. ) ;
#75825=CARTESIAN_POINT ( 'NONE',  ( -0.1232682223025967638, 1.078237662714072176, -3.935195272298547042 ) ) ;
#75830=CARTESIAN_POINT ( 'NONE',  ( -1.840814964558169287, 2.729664688135040596, 0.5314960629921260393 ) ) ;
#75837=CARTESIAN_POINT ( 'NONE',  ( 0.4177787735907000366, 0.4110443821404751730, -1.736336963694947944 ) ) ;
#75845=VERTEX_POINT ( 'NONE', #70307 ) ;
#75861=CARTESIAN_POINT ( 'NONE',  ( -0.3230088838496750214, 1.189621120221113770, -1.964944096575241828 ) ) ;
#75865=ORIENTED_EDGE ( 'NONE', *, *, #13485, .F. ) ;
#75883=ORIENTED_EDGE ( 'NONE', *, *, #27454, .F. ) ;
#75903=EDGE_CURVE ( 'NONE', #66338, #26273, #33277, .T. ) ;
#75907=CARTESIAN_POINT ( 'NONE',  ( -0.2885979965725595231, 1.160566086728933133, 1.939267709711407717 ) ) ;
#75913=CARTESIAN_POINT ( 'NONE',  ( 0.000000000000000000, 2.755905511811024056, 0.000000000000000000 ) ) ;
#75921=CARTESIAN_POINT ( 'NONE',  ( 1.016821367227983552, 1.537401574803149984, 0.4744094488188975722 ) ) ;
#75942=CARTESIAN_POINT ( 'NONE',  ( -2.170146923806554273, 1.537401574803149984, -0.4744094488188975722 ) ) ;
#75948=EDGE_CURVE ( 'NONE', #39954, #49578, #16589, .T. ) ;
#75952=CARTESIAN_POINT ( 'NONE',  ( -0.3247161055182421485, 1.191192147208269159, 1.074094784059450802 ) ) ;
#75971=PLANE ( 'NONE',  #54700 ) ;
#75983=ORIENTED_EDGE ( 'NONE', *, *, #68146, .F. ) ;
#75984=DIRECTION ( 'NONE',  ( 0.000000000000000000, 0.000000000000000000, -1.000000000000000000 ) ) ;
#75988=CARTESIAN_POINT ( 'NONE',  ( -3.821484228344193657, 2.755905511811024056, -0.5314960629921260393 ) ) ;
#75989=CARTESIAN_POINT ( 'NONE',  ( 0.000000000000000000, 1.724409448818897905, -2.362204724409448620 ) ) ;
#76006=EDGE_LOOP ( 'NONE', ( #34554, #56499, #53682, #62632 ) ) ;
#76020=B_SPLINE_CURVE_WITH_KNOTS ( 'NONE', 3,
 ( #25276, #44214, #43390, #75415 ),
 .UNSPECIFIED., .F., .F.,
 ( 4, 4 ),
 ( 0.08702371034448001808, 0.08847090869701748628 ),
 .UNSPECIFIED. ) ;
#76043=ADVANCED_FACE ( 'NONE', ( #6750 ), #26535, .T. ) ;
#76046=CARTESIAN_POINT ( 'NONE',  ( 0.4425803288943399583, 1.365943002350758384, 2.619481425262184526 ) ) ;
#76050=CARTESIAN_POINT ( 'NONE',  ( 1.076935383196057305, 5.463695987328539379E-17, 0.3149606299212603933 ) ) ;
#76060=ORIENTED_EDGE ( 'NONE', *, *, #28501, .F. ) ;
#76075=ORIENTED_EDGE ( 'NONE', *, *, #66367, .T. ) ;
#76083=FACE_OUTER_BOUND ( 'NONE', #37775, .T. ) ;
#76093=DIRECTION ( 'NONE',  ( 0.000000000000000000, 0.000000000000000000, 1.000000000000000000 ) ) ;
#76100=DIRECTION ( 'NONE',  ( -3.491481338843132961E-15, -0.000000000000000000, 1.000000000000000000 ) ) ;
#76107=CIRCLE ( 'NONE', #23697, 0.3149606299212597826 ) ;
#76108=CIRCLE ( 'NONE', #63949, 0.5118110236220472231 ) ;
#76140=CARTESIAN_POINT ( 'NONE',  ( -3.924565315667062126, 1.180549598472639961, -0.3129926727910089523 ) ) ;
#76147=CARTESIAN_POINT ( 'NONE',  ( 0.000000000000000000, 2.559055118110236560, 0.000000000000000000 ) ) ;
#76156=AXIS2_PLACEMENT_3D ( 'NONE', #33369, #64932, #7270 ) ;
#76164=ORIENTED_EDGE ( 'NONE', *, *, #15715, .T. ) ;
#76177=EDGE_LOOP ( 'NONE', ( #58761, #20593, #25072, #61803 ) ) ;
#76179=EDGE_LOOP ( 'NONE', ( #43314, #45407, #5765, #77503 ) ) ;
#76181=CARTESIAN_POINT ( 'NONE',  ( 2.571327113428977018, 1.453547212638085950, -0.4672029448317638889 ) ) ;
#76198=B_SPLINE_CURVE_WITH_KNOTS ( 'NONE', 3,
 ( #10775, #16686, #43557, #4040 ),
 .UNSPECIFIED., .F., .F.,
 ( 4, 4 ),
 ( 0.1183700917297995092, 0.1198164042326150397 ),
 .UNSPECIFIED. ) ;
#76206=EDGE_CURVE ( 'NONE', #27710, #39595, #61422, .T. ) ;
#76213=CARTESIAN_POINT ( 'NONE',  ( -2.666386537446475913, 1.301102360844756722, 0.4123394245947728520 ) ) ;
#76216=CIRCLE ( 'NONE', #3643, 1.122047244094488194 ) ;
#76220=AXIS2_PLACEMENT_3D ( 'NONE', #54781, #48050, #73751 ) ;
#76222=VECTOR ( 'NONE', #37631, 39.37007874015748143 ) ;
#76232=FACE_OUTER_BOUND ( 'NONE', #25191, .T. ) ;
#76263=CARTESIAN_POINT ( 'NONE',  ( 4.821444091131311894E-16, 2.755905511811024056, 3.937007874015748143 ) ) ;
#76267=ADVANCED_FACE ( 'NONE', ( #3772 ), #67757, .F. ) ;
#76275=DIRECTION ( 'NONE',  ( 0.000000000000000000, 0.000000000000000000, -1.000000000000000000 ) ) ;
#76276=AXIS2_PLACEMENT_3D ( 'NONE', #31282, #70000, #37601 ) ;
#76278=ORIENTED_EDGE ( 'NONE', *, *, #41310, .F. ) ;
#76298=ORIENTED_EDGE ( 'NONE', *, *, #26365, .F. ) ;
#76300=EDGE_LOOP ( 'NONE', ( #64364, #35148, #50872, #8806 ) ) ;
#76304=CARTESIAN_POINT ( 'NONE',  ( 0.5314960629921325896, 2.755905511811024056, -1.895394334970790018 ) ) ;
#76327=CARTESIAN_POINT ( 'NONE',  ( -0.3149606299212459048, 2.559055118110236560, -3.937007874015763242 ) ) ;
#76347=DIRECTION ( 'NONE',  ( 1.047444401652940007E-14, -0.000000000000000000, -1.000000000000000000 ) ) ;
#76351=ORIENTED_EDGE ( 'NONE', *, *, #50027, .T. ) ;
#76364=CARTESIAN_POINT ( 'NONE',  ( -0.1973832605630230219, 1.105719693649961810, 1.104646637927854336 ) ) ;
#76365=CARTESIAN_POINT ( 'NONE',  ( -1.827151725772330648, 2.742788129994044866, -0.5314960629921260393 ) ) ;
#76392=ORIENTED_EDGE ( 'NONE', *, *, #9399, .T. ) ;
#76399=PLANE ( 'NONE',  #36944 ) ;
#76408=ORIENTED_EDGE ( 'NONE', *, *, #82874, .T. ) ;
#76409=FACE_OUTER_BOUND ( 'NONE', #39339, .T. ) ;
#76410=B_SPLINE_CURVE_WITH_KNOTS ( 'NONE', 3,
 ( #14830, #66584, #8920, #53930 ),
 .UNSPECIFIED., .F., .F.,
 ( 4, 4 ),
 ( 2.888536477662776634E-07, 0.001436607511248048788 ),
 .UNSPECIFIED. ) ;
#76412=DIRECTION ( 'NONE',  ( 0.000000000000000000, 1.000000000000000000, 0.000000000000000000 ) ) ;
#76416=VERTEX_POINT ( 'NONE', #48370 ) ;
#76417=DIRECTION ( 'NONE',  ( -1.000000000000000000, -0.000000000000000000, -0.000000000000000000 ) ) ;
#76418=CARTESIAN_POINT ( 'NONE',  ( -3.924389226575468737, 2.755905511811024056, -0.3149606299212598381 ) ) ;
#76440=CARTESIAN_POINT ( 'NONE',  ( 0.000000000000000000, 2.755905511811024056, 0.000000000000000000 ) ) ;
#76461=CARTESIAN_POINT ( 'NONE',  ( 0.4102808022082889416, 1.299212598425196985, -1.382164990278189398 ) ) ;
#76474=VERTEX_POINT ( 'NONE', #5821 ) ;
#76489=EDGE_LOOP ( 'NONE', ( #56760, #66677, #27308, #31107 ) ) ;
#76496=FACE_OUTER_BOUND ( 'NONE', #60873, .T. ) ;
#76505=EDGE_LOOP ( 'NONE', ( #55466, #30724, #76164, #15969 ) ) ;
#76535=DIRECTION ( 'NONE',  ( 0.000000000000000000, 1.000000000000000000, 0.000000000000000000 ) ) ;
#76551=CARTESIAN_POINT ( 'NONE',  ( -3.911874546793528307, 1.370070907001625482, 0.4441891910510556429 ) ) ;
#76555=DIRECTION ( 'NONE',  ( 0.000000000000000000, 0.000000000000000000, 1.000000000000000000 ) ) ;
#76557=ORIENTED_EDGE ( 'NONE', *, *, #57094, .T. ) ;
#76563=CARTESIAN_POINT ( 'NONE',  ( -0.3149606299212459048, 2.559055118110236560, -3.937007874015763242 ) ) ;
#76566=DIRECTION ( 'NONE',  ( 1.000000000000000000, -0.000000000000000000, -0.000000000000000000 ) ) ;
#76572=EDGE_LOOP ( 'NONE', ( #80018, #11458, #78896, #52430 ) ) ;
#76585=EDGE_LOOP ( 'NONE', ( #54653, #60447 ) ) ;
#76587=VERTEX_POINT ( 'NONE', #24760 ) ;
#76589=CARTESIAN_POINT ( 'NONE',  ( 2.784923006909812759, 1.160811571118577579, -0.2889173282905524442 ) ) ;
#76605=EDGE_CURVE ( 'NONE', #15345, #45100, #82481, .T. ) ;
#76632=CARTESIAN_POINT ( 'NONE',  ( -1.559171609364246924, 0.4110443821404751730, 0.4177787735906735578 ) ) ;
#76635=CYLINDRICAL_SURFACE ( 'NONE', #70634, 0.09842519685039351207 ) ;
#76641=CARTESIAN_POINT ( 'NONE',  ( -0.4109163706260607896, 1.299800539985194403, -3.915511880786665788 ) ) ;
#76646=CARTESIAN_POINT ( 'NONE',  ( 1.881758995267131418, 2.742776584231126247, 0.5314960629921260393 ) ) ;
#76661=ORIENTED_EDGE ( 'NONE', *, *, #50364, .F. ) ;
#76666=LINE ( 'NONE', #77086, #38579 ) ;
#76668=LINE ( 'NONE', #51807, #79002 ) ;
#76679=ORIENTED_EDGE ( 'NONE', *, *, #57395, .F. ) ;
#76725=CARTESIAN_POINT ( 'NONE',  ( -0.2510736293007193032, 1.134572453438778883, 1.915946413328042386 ) ) ;
#76730=DIRECTION ( 'NONE',  ( 3.552713678800500929E-15, 0.000000000000000000, 1.000000000000000000 ) ) ;
#76736=AXIS2_PLACEMENT_3D ( 'NONE', #68934, #69759, #75261 ) ;
#76740=DIRECTION ( 'NONE',  ( 0.000000000000000000, 0.000000000000000000, -1.000000000000000000 ) ) ;
#76743=CARTESIAN_POINT ( 'NONE',  ( 0.9285414500055709786, 2.165354330708662012, 0.6299212598425202314 ) ) ;
#76749=FACE_OUTER_BOUND ( 'NONE', #46971, .T. ) ;
#76752=CARTESIAN_POINT ( 'NONE',  ( 0.000000000000000000, 2.755905511811024056, 0.000000000000000000 ) ) ;
#76757=EDGE_CURVE ( 'NONE', #50071, #80735, #18060, .T. ) ;
#76790=CIRCLE ( 'NONE', #48551, 2.204724409448819422 ) ;
#76795=EDGE_LOOP ( 'NONE', ( #11767, #39938, #29246, #37841 ) ) ;
#76797=VERTEX_POINT ( 'NONE', #42877 ) ;
#76812=DIRECTION ( 'NONE',  ( -3.491481338843133355E-15, -0.000000000000000000, 1.000000000000000000 ) ) ;
#76819=CARTESIAN_POINT ( 'NONE',  ( 0.6299212598424790421, 2.165354330708661568, 3.886287458032468667 ) ) ;
#76828=EDGE_CURVE ( 'NONE', #77301, #48318, #55542, .T. ) ;
#76845=ORIENTED_EDGE ( 'NONE', *, *, #63016, .T. ) ;
#76862=CARTESIAN_POINT ( 'NONE',  ( 0.4732338166265936397, 1.502938029856536684, 2.557145251749653347 ) ) ;
#76876=ORIENTED_EDGE ( 'NONE', *, *, #14394, .T. ) ;
#76891=ORIENTED_EDGE ( 'NONE', *, *, #80504, .F. ) ;
#76901=CARTESIAN_POINT ( 'NONE',  ( 0.5314960629920847390, 2.559055118110236560, 3.937007874015794773 ) ) ;
#76903=CARTESIAN_POINT ( 'NONE',  ( 1.141392835773559211, 0.4110443821404751730, 1.141392835773562764 ) ) ;
#76913=AXIS2_PLACEMENT_3D ( 'NONE', #37108, #9793, #80925 ) ;
#76918=EDGE_CURVE ( 'NONE', #60631, #42276, #3178, .T. ) ;
#76960=CARTESIAN_POINT ( 'NONE',  ( -3.934081685436475517, 1.087899594981445617, -0.1524895619889924669 ) ) ;
#76983=ORIENTED_EDGE ( 'NONE', *, *, #34274, .F. ) ;
#76998=VERTEX_POINT ( 'NONE', #81214 ) ;
#77002=DIRECTION ( 'NONE',  ( 0.000000000000000000, -1.000000000000000000, 0.000000000000000000 ) ) ;
#77028=AXIS2_PLACEMENT_3D ( 'NONE', #61854, #4195, #10527 ) ;
#77035=CARTESIAN_POINT ( 'NONE',  ( 3.937007874015748143, 2.755905511811024056, -0.5314960629921260393 ) ) ;
#77057=CARTESIAN_POINT ( 'NONE',  ( -0.3575644331232493700, 1.224046602586773336, -3.920799917772898713 ) ) ;
#77065=VECTOR ( 'NONE', #60909, 39.37007874015748143 ) ;
#77070=FACE_OUTER_BOUND ( 'NONE', #70057, .T. ) ;
#77079=ORIENTED_EDGE ( 'NONE', *, *, #24269, .F. ) ;
#77083=ORIENTED_EDGE ( 'NONE', *, *, #80583, .T. ) ;
#77086=CARTESIAN_POINT ( 'NONE',  ( 3.937007874015748143, 2.165354330708661568, -0.6299212598425196763 ) ) ;
#77097=DIRECTION ( 'NONE',  ( 0.000000000000000000, -1.000000000000000000, 0.000000000000000000 ) ) ;
#77101=ORIENTED_EDGE ( 'NONE', *, *, #30460, .F. ) ;
#77113=DIRECTION ( 'NONE',  ( 0.000000000000000000, 1.000000000000000000, 1.408710688920637755E-15 ) ) ;
#77115=DIRECTION ( 'NONE',  ( -0.000000000000000000, -1.000000000000000000, -0.000000000000000000 ) ) ;
#77116=ORIENTED_EDGE ( 'NONE', *, *, #33182, .T. ) ;
#77117=ORIENTED_EDGE ( 'NONE', *, *, #5158, .F. ) ;
#77121=DIRECTION ( 'NONE',  ( 0.000000000000000000, -1.000000000000000000, -0.000000000000000000 ) ) ;
#77143=CARTESIAN_POINT ( 'NONE',  ( -3.900966923095589678, 2.755905511811024056, 0.5314960629921260393 ) ) ;
#77168=PLANE ( 'NONE',  #19193 ) ;
#77195=FACE_OUTER_BOUND ( 'NONE', #20591, .T. ) ;
#77216=CARTESIAN_POINT ( 'NONE',  ( -0.3149606299212558969, 2.559055118110236560, -1.076935383196058638 ) ) ;
#77221=CARTESIAN_POINT ( 'NONE',  ( 6.267877385347666114E-17, 1.062992125984252745, 2.874015748031495843 ) ) ;
#77229=ORIENTED_EDGE ( 'NONE', *, *, #53988, .F. ) ;
#77239=CARTESIAN_POINT ( 'NONE',  ( -2.362204724409448620, 0.03937007874015751446, 0.5118110236220224651 ) ) ;
#77259=AXIS2_PLACEMENT_3D ( 'NONE', #5678, #11606, #25028 ) ;
#77263=CARTESIAN_POINT ( 'NONE',  ( 0.4359958488159444423, 1.724409448818900570, 2.630268417803970138 ) ) ;
#77281=CARTESIAN_POINT ( 'NONE',  ( 0.2730112473383900507, 1.149291835544637319, -1.662080954481470529 ) ) ;
#77301=VERTEX_POINT ( 'NONE', #33968 ) ;
#77311=VERTEX_POINT ( 'NONE', #71894 ) ;
#77313=ORIENTED_EDGE ( 'NONE', *, *, #30007, .T. ) ;
#77314=CARTESIAN_POINT ( 'NONE',  ( 3.937007874015748143, 2.559055118110236560, 0.5314960629921260393 ) ) ;
#77329=ORIENTED_EDGE ( 'NONE', *, *, #6944, .F. ) ;
#77337=CARTESIAN_POINT ( 'NONE',  ( 1.867405098639527417, 1.081388112195863949, 0.1351566381869950262 ) ) ;
#77351=CARTESIAN_POINT ( 'NONE',  ( -0.08351193659984793016, 1.070350416549052497, -1.608688096019881497 ) ) ;
#77376=VECTOR ( 'NONE', #42739, 39.37007874015748143 ) ;
#77386=CARTESIAN_POINT ( 'NONE',  ( 0.000000000000000000, 1.929133858267716661, 2.362204724409448620 ) ) ;
#77389=EDGE_CURVE ( 'NONE', #21108, #42501, #13400, .T. ) ;
#77396=CARTESIAN_POINT ( 'NONE',  ( 0.000000000000000000, 0.03937007874015751446, 2.362204724409448620 ) ) ;
#77415=ORIENTED_EDGE ( 'NONE', *, *, #77389, .T. ) ;
#77419=AXIS2_PLACEMENT_3D ( 'NONE', #36848, #75580, #75167 ) ;
#77420=VECTOR ( 'NONE', #4780, 39.37007874015748143 ) ;
#77421=CARTESIAN_POINT ( 'NONE',  ( 2.619388402063373533, 1.366082762360723901, -0.4426340671871345500 ) ) ;
#77432=CARTESIAN_POINT ( 'NONE',  ( -2.586150256253501478, 1.653403552777528596, 0.4602852883866567768 ) ) ;
#77441=AXIS2_PLACEMENT_3D ( 'NONE', #59515, #15335, #9426 ) ;
#77451=CARTESIAN_POINT ( 'NONE',  ( -2.554262525012342966, 1.537401574803149984, -0.4744094488188975722 ) ) ;
#77475=AXIS2_PLACEMENT_3D ( 'NONE', #27967, #66702, #9035 ) ;
#77479=VECTOR ( 'NONE', #52428, 39.37007874015748143 ) ;
#77493=CARTESIAN_POINT ( 'NONE',  ( 0.4744094488189052328, 1.537401574803149984, -2.170146923806634653 ) ) ;
#77498=DIRECTION ( 'NONE',  ( 0.000000000000000000, -1.000000000000000000, 0.000000000000000000 ) ) ;
#77499=AXIS2_PLACEMENT_3D ( 'NONE', #35629, #54973, #61291 ) ;
#77503=ORIENTED_EDGE ( 'NONE', *, *, #27189, .F. ) ;
#77512=CARTESIAN_POINT ( 'NONE',  ( 6.372542394380578105E-15, 1.062992125984252523, -1.629220936382730134 ) ) ;
#77521=CARTESIAN_POINT ( 'NONE',  ( -0.4744094488188894121, 1.537401574803149984, -2.170146923806595574 ) ) ;
#77529=B_SPLINE_CURVE_WITH_KNOTS ( 'NONE', 3,
 ( #15775, #29620, #9857, #10278 ),
 .UNSPECIFIED., .F., .F.,
 ( 4, 4 ),
 ( 0.08422315286269969892, 0.08567085022608438016 ),
 .UNSPECIFIED. ) ;
#77536=CARTESIAN_POINT ( 'NONE',  ( 2.570293882282742803, 2.742780008954323723, -0.5314960629921260393 ) ) ;
#77541=DIRECTION ( 'NONE',  ( 0.000000000000000000, 0.000000000000000000, -1.000000000000000000 ) ) ;
#77542=EDGE_LOOP ( 'NONE', ( #72854, #7188, #39845, #49953 ) ) ;
#77544=CONICAL_SURFACE ( 'NONE', #3583, 0.1190944881889763746, 0.8726646259971648778 ) ;
#77548=AXIS2_PLACEMENT_3D ( 'NONE', #60150, #66897, #29400 ) ;
#77552=CARTESIAN_POINT ( 'NONE',  ( 0.4677827689124922084, 0.03937007874015747977, -2.154527559055118946 ) ) ;
#77575=FACE_OUTER_BOUND ( 'NONE', #69562, .T. ) ;
#77582=CARTESIAN_POINT ( 'NONE',  ( 1.044213977778944535, 1.299421820005424166, -0.4106937405380285400 ) ) ;
#77585=FACE_OUTER_BOUND ( 'NONE', #8381, .T. ) ;
#77597=AXIS2_PLACEMENT_3D ( 'NONE', #51381, #64034, #39618 ) ;
#77641=ORIENTED_EDGE ( 'NONE', *, *, #73388, .T. ) ;
#77645=CARTESIAN_POINT ( 'NONE',  ( -0.03430998917087550032, 1.064156075168070537, 2.872937013333135337 ) ) ;
#77654=DIRECTION ( 'NONE',  ( 1.000000000000000000, -0.000000000000000000, -0.000000000000000000 ) ) ;
#77663=LINE ( 'NONE', #51536, #58367 ) ;
#77668=ADVANCED_FACE ( 'NONE', ( #64738 ), #11232, .T. ) ;
#77693=EDGE_LOOP ( 'NONE', ( #82868, #55773, #61769, #19207 ) ) ;
#77707=CARTESIAN_POINT ( 'NONE',  ( 0.4697171261335883474, 1.606100245667710702, 2.565525098582279728 ) ) ;
#77719=CARTESIAN_POINT ( 'NONE',  ( 1.348312163386739426, 1.062992125984252079, 0.8371118098809627872 ) ) ;
#77720=ORIENTED_EDGE ( 'NONE', *, *, #64730, .F. ) ;
#77721=VERTEX_POINT ( 'NONE', #27263 ) ;
#77748=CARTESIAN_POINT ( 'NONE',  ( 5.333846858410640380E-15, 1.062992125984252079, -1.444810848096780953 ) ) ;
#77755=VERTEX_POINT ( 'NONE', #64318 ) ;
#77762=CARTESIAN_POINT ( 'NONE',  ( -2.167714792466712392, 1.572145545125847921, 0.4734416007054412789 ) ) ;
#77764=FACE_OUTER_BOUND ( 'NONE', #79425, .T. ) ;
#77795=EDGE_CURVE ( 'NONE', #40450, #20906, #30019, .T. ) ;
#77804=CARTESIAN_POINT ( 'NONE',  ( -3.911208592539883622, 1.384429027863568473, -0.4501334968650620993 ) ) ;
#77818=EDGE_CURVE ( 'NONE', #24318, #29055, #59135, .T. ) ;
#77821=CARTESIAN_POINT ( 'NONE',  ( 0.2507089876491974678, 1.134347693112636835, -3.929038657107195576 ) ) ;
#77827=ORIENTED_EDGE ( 'NONE', *, *, #33231, .T. ) ;
#77836=EDGE_CURVE ( 'NONE', #36023, #17178, #16650, .T. ) ;
#77845=PLANE ( 'NONE',  #54249 ) ;
#77909=ORIENTED_EDGE ( 'NONE', *, *, #41314, .F. ) ;
#77916=DIRECTION ( 'NONE',  ( -3.491481338843132961E-15, -0.000000000000000000, 1.000000000000000000 ) ) ;
#77924=ORIENTED_EDGE ( 'NONE', *, *, #51138, .F. ) ;
#77931=DIRECTION ( 'NONE',  ( -0.000000000000000000, -1.000000000000000000, -0.000000000000000000 ) ) ;
#77943=ORIENTED_EDGE ( 'NONE', *, *, #9565, .F. ) ;
#77956=ADVANCED_FACE ( 'NONE', ( #8748 ), #61321, .F. ) ;
#77963=DIRECTION ( 'NONE',  ( 1.000000000000000000, 1.734723475976808080E-16, 3.491481338843132961E-15 ) ) ;
#77968=CARTESIAN_POINT ( 'NONE',  ( -3.821484228344193657, 2.755905511811024056, 0.5314960629921260393 ) ) ;
#77984=EDGE_CURVE ( 'NONE', #52887, #75845, #41145, .T. ) ;
#77992=EDGE_CURVE ( 'NONE', #33187, #12202, #63662, .T. ) ;
#78000=EDGE_CURVE ( 'NONE', #69342, #26718, #35245, .T. ) ;
#78004=CARTESIAN_POINT ( 'NONE',  ( 0.3134538944422693985, 1.179955895207738914, 3.924571280271134111 ) ) ;
#78014=AXIS2_PLACEMENT_3D ( 'NONE', #43559, #18332, #42741 ) ;
#78018=FACE_OUTER_BOUND ( 'NONE', #60527, .T. ) ;
#78028=DIRECTION ( 'NONE',  ( 0.000000000000000000, 0.000000000000000000, -1.000000000000000000 ) ) ;
#78038=CARTESIAN_POINT ( 'NONE',  ( -0.4602855208775665785, 1.653389129435536509, -2.138261236553457678 ) ) ;
#78059=ORIENTED_EDGE ( 'NONE', *, *, #35860, .T. ) ;
#78063=CARTESIAN_POINT ( 'NONE',  ( -0.2100141437675596967, 1.111707297776193926, 2.829210744671456723 ) ) ;
#78064=CARTESIAN_POINT ( 'NONE',  ( 3.937007874015748143, 2.165354330708662012, 0.6299212598425202314 ) ) ;
#78071=ORIENTED_EDGE ( 'NONE', *, *, #6986, .T. ) ;
#78072=VECTOR ( 'NONE', #16165, 39.37007874015748143 ) ;
#78074=CARTESIAN_POINT ( 'NONE',  ( 0.000000000000000000, 2.165354330708661568, 0.000000000000000000 ) ) ;
#78076=CARTESIAN_POINT ( 'NONE',  ( 3.900966923095589678, 2.677165354330708791, -0.5314960629921260393 ) ) ;
#78112=EDGE_LOOP ( 'NONE', ( #22058, #51838, #38541, #65640 ) ) ;
#78126=CARTESIAN_POINT ( 'NONE',  ( 0.3443296571407519213, 1.210789077865271013, -1.720740846584503103 ) ) ;
#78141=ORIENTED_EDGE ( 'NONE', *, *, #50179, .F. ) ;
#78158=ORIENTED_EDGE ( 'NONE', *, *, #13121, .F. ) ;
#78159=LINE ( 'NONE', #46144, #20726 ) ;
#78166=CARTESIAN_POINT ( 'NONE',  ( -0.03443470937339728616, 0.2929341459200028863, -1.537015892239756099 ) ) ;
#78169=CARTESIAN_POINT ( 'NONE',  ( 0.4469779880791947546, 1.697109554835854572, 2.112686649479581735 ) ) ;
#78175=ORIENTED_EDGE ( 'NONE', *, *, #55030, .T. ) ;
#78176=VERTEX_POINT ( 'NONE', #40318 ) ;
#78183=CARTESIAN_POINT ( 'NONE',  ( 2.170146923806595129, 1.537401574803149984, 0.4744094488188975722 ) ) ;
#78191=DIRECTION ( 'NONE',  ( 0.000000000000000000, 0.000000000000000000, 1.000000000000000000 ) ) ;
#78209=CARTESIAN_POINT ( 'NONE',  ( -1.016821367227983997, 1.553445615596289908, -0.4744094488188977388 ) ) ;
#78215=DIRECTION ( 'NONE',  ( 0.000000000000000000, 0.000000000000000000, -1.000000000000000000 ) ) ;
#78226=LINE ( 'NONE', #20559, #26453 ) ;
#78230=ORIENTED_EDGE ( 'NONE', *, *, #20875, .T. ) ;
#78231=CARTESIAN_POINT ( 'NONE',  ( 0.4562720003150377845, 1.668198494846154567, -2.594288149172116142 ) ) ;
#78241=CARTESIAN_POINT ( 'NONE',  ( 0.1527255018715594492, 1.087979116479378616, -3.934072586421137441 ) ) ;
#78247=ORIENTED_EDGE ( 'NONE', *, *, #11555, .T. ) ;
#78262=VERTEX_POINT ( 'NONE', #27683 ) ;
#78265=CARTESIAN_POINT ( 'NONE',  ( 2.610466197084835294, 1.379671404989097239, 0.4476723508032718346 ) ) ;
#78272=DIRECTION ( 'NONE',  ( 0.000000000000000000, -1.000000000000000000, 0.000000000000000000 ) ) ;
#78295=CARTESIAN_POINT ( 'NONE',  ( -2.565964038698705707, 1.605872332714550099, -0.4695140184743391010 ) ) ;
#78309=VECTOR ( 'NONE', #38019, 39.37007874015748143 ) ;
#78330=ORIENTED_EDGE ( 'NONE', *, *, #57885, .F. ) ;
#78342=LINE ( 'NONE', #8869, #55605 ) ;
#78352=CARTESIAN_POINT ( 'NONE',  ( -1.559171609364246924, 0.4110443821404751730, 0.4177787735906735578 ) ) ;
#78361=CARTESIAN_POINT ( 'NONE',  ( 0.000000000000000000, 2.755905511811024056, 0.000000000000000000 ) ) ;
#78383=CARTESIAN_POINT ( 'NONE',  ( 3.920801026570782888, 1.224049986093448616, -0.3575349072971868991 ) ) ;
#78384=EDGE_CURVE ( 'NONE', #80970, #54650, #51501, .T. ) ;
#78390=CARTESIAN_POINT ( 'NONE',  ( 2.118110236220474007, 0.000000000000000000, -0.4498537592782824723 ) ) ;
#78404=B_SPLINE_CURVE_WITH_KNOTS ( 'NONE', 3,
 ( #22613, #36069, #4078, #4490 ),
 .UNSPECIFIED., .F., .F.,
 ( 4, 4 ),
 ( 0.09865403381126922056, 0.1000779257405588624 ),
 .UNSPECIFIED. ) ;
#78419=VECTOR ( 'NONE', #76347, 39.37007874015748143 ) ;
#78423=CARTESIAN_POINT ( 'NONE',  ( 1.017181940522988270, 1.506165534434959152, -0.4736389124302199383 ) ) ;
#78426=CARTESIAN_POINT ( 'NONE',  ( 0.000000000000000000, 0.000000000000000000, 0.000000000000000000 ) ) ;
#78455=EDGE_CURVE ( 'NONE', #66675, #43601, #66411, .T. ) ;
#78460=CARTESIAN_POINT ( 'NONE',  ( 0.2774227409090211371, 1.152252460295412062, 1.087290629417145382 ) ) ;
#78484=CARTESIAN_POINT ( 'NONE',  ( -0.5314960629921122726, 2.755905511811024056, -3.937007874015763687 ) ) ;
#78489=AXIS2_PLACEMENT_3D ( 'NONE', #8384, #66046, #41196 ) ;
#78491=PLANE ( 'NONE',  #26461 ) ;
#78496=CARTESIAN_POINT ( 'NONE',  ( 1.348312163386739426, 0.2929341459200028863, 0.8371118098809627872 ) ) ;
#78520=DIRECTION ( 'NONE',  ( 0.000000000000000000, -1.000000000000000000, 0.000000000000000000 ) ) ;
#78550=VECTOR ( 'NONE', #7165, 39.37007874015748143 ) ;
#78552=DIRECTION ( 'NONE',  ( -0.000000000000000000, -1.000000000000000000, -0.000000000000000000 ) ) ;
#78589=CYLINDRICAL_SURFACE ( 'NONE', #46916, 0.4744094488188972947 ) ;
#78591=CARTESIAN_POINT ( 'NONE',  ( 0.5314960629921396951, 2.755905511811024056, -3.937007874015760578 ) ) ;
#78594=VECTOR ( 'NONE', #73819, 39.37007874015748143 ) ;
#78599=VERTEX_POINT ( 'NONE', #18375 ) ;
#78605=CARTESIAN_POINT ( 'NONE',  ( -2.170146923806675510, 1.537401574803149984, 0.4744094488188970171 ) ) ;
#78612=CYLINDRICAL_SURFACE ( 'NONE', #59988, 1.122047244094488194 ) ;
#78628=FACE_OUTER_BOUND ( 'NONE', #28226, .T. ) ;
#78631=DIRECTION ( 'NONE',  ( 0.000000000000000000, 0.000000000000000000, -1.000000000000000000 ) ) ;
#78646=B_SPLINE_CURVE_WITH_KNOTS ( 'NONE', 3,
 ( #17606, #4964, #23485, #30631, #56296, #81993, #24307, #49977 ),
 .UNSPECIFIED., .F., .F.,
 ( 4, 2, 2, 4 ),
 ( 0.01399351151594419376, 0.01520974288759853639, 0.01642597425925287902, 0.01885843700256156080 ),
 .UNSPECIFIED. ) ;
#78653=DIRECTION ( 'NONE',  ( -0.000000000000000000, -1.000000000000000000, -0.000000000000000000 ) ) ;
#78665=EDGE_LOOP ( 'NONE', ( #62800, #5463, #75475, #20050 ) ) ;
#78666=VECTOR ( 'NONE', #52021, 39.37007874015748143 ) ;
#78668=ORIENTED_EDGE ( 'NONE', *, *, #33231, .F. ) ;
#78686=CARTESIAN_POINT ( 'NONE',  ( -1.456124044357799185, 1.149361882009420466, 0.2731108461632001383 ) ) ;
#78718=CARTESIAN_POINT ( 'NONE',  ( -0.5314960629921350321, 2.755905511811024056, 2.583694225513478937 ) ) ;
#78726=CARTESIAN_POINT ( 'NONE',  ( -0.5314960629921123836, 2.697625129285034173, -3.898413161119333115 ) ) ;
#78744=CARTESIAN_POINT ( 'NONE',  ( 0.000000000000000000, 0.000000000000000000, 0.000000000000000000 ) ) ;
#78762=AXIS2_PLACEMENT_3D ( 'NONE', #15362, #54888, #73434 ) ;
#78765=ORIENTED_EDGE ( 'NONE', *, *, #9399, .F. ) ;
#78768=ORIENTED_EDGE ( 'NONE', *, *, #48666, .T. ) ;
#78774=CARTESIAN_POINT ( 'NONE',  ( 0.05172391896678928819, 1.065813321887014276, -1.498852247951555583 ) ) ;
#78783=ORIENTED_EDGE ( 'NONE', *, *, #3893, .F. ) ;
#78786=ORIENTED_EDGE ( 'NONE', *, *, #79432, .F. ) ;
#78800=LINE ( 'NONE', #13989, #6327 ) ;
#78803=CARTESIAN_POINT ( 'NONE',  ( 3.933461957825151067, 1.093339152432855510, -0.1676739346958345533 ) ) ;
#78821=DIRECTION ( 'NONE',  ( -0.000000000000000000, -1.000000000000000000, -0.000000000000000000 ) ) ;
#78826=CIRCLE ( 'NONE', #42497, 1.122047244094488194 ) ;
#78832=CYLINDRICAL_SURFACE ( 'NONE', #82827, 0.2165354330708660624 ) ;
#78838=CARTESIAN_POINT ( 'NONE',  ( 1.047355619713164820, 1.286041797112411400, -0.4026416502575907441 ) ) ;
#78841=CARTESIAN_POINT ( 'NONE',  ( 0.4494576562008150700, 1.384774454230845109, 3.911270836792677841 ) ) ;
#78852=EDGE_CURVE ( 'NONE', #48126, #72870, #50256, .T. ) ;
#78869=EDGE_CURVE ( 'NONE', #66965, #46125, #82539, .T. ) ;
#78873=ADVANCED_FACE ( 'NONE', ( #24882 ), #44231, .F. ) ;
#78877=VECTOR ( 'NONE', #12757, 39.37007874015748143 ) ;
#78881=AXIS2_PLACEMENT_3D ( 'NONE', #78361, #20692, #73707 ) ;
#78882=CONICAL_SURFACE ( 'NONE', #42566, 0.1978346456692914035, 0.8726646259971685415 ) ;
#78896=ORIENTED_EDGE ( 'NONE', *, *, #32173, .F. ) ;
#78898=ORIENTED_EDGE ( 'NONE', *, *, #50835, .T. ) ;
#78902=DIRECTION ( 'NONE',  ( 0.000000000000000000, -1.000000000000000000, -0.000000000000000000 ) ) ;
#78903=LINE ( 'NONE', #72573, #32440 ) ;
#78911=CARTESIAN_POINT ( 'NONE',  ( -1.087387972035418926, 1.151979311713951182, -0.2770360422623977525 ) ) ;
#78918=ORIENTED_EDGE ( 'NONE', *, *, #75903, .F. ) ;
#78920=CARTESIAN_POINT ( 'NONE',  ( 0.5314960629920851831, 2.677165354330708791, 3.900966923095595451 ) ) ;
#78935=VECTOR ( 'NONE', #12073, 39.37007874015748143 ) ;
#78938=VECTOR ( 'NONE', #27062, 39.37007874015748143 ) ;
#78956=ORIENTED_EDGE ( 'NONE', *, *, #72867, .F. ) ;
#78980=VERTEX_POINT ( 'NONE', #58111 ) ;
#78981=ORIENTED_EDGE ( 'NONE', *, *, #15919, .F. ) ;
#78984=EDGE_CURVE ( 'NONE', #49485, #43641, #32872, .T. ) ;
#78988=DIRECTION ( 'NONE',  ( -1.000000000000000000, -8.673617379884021667E-16, 0.000000000000000000 ) ) ;
#78998=VERTEX_POINT ( 'NONE', #19834 ) ;
#79000=ORIENTED_EDGE ( 'NONE', *, *, #54265, .T. ) ;
#79001=CARTESIAN_POINT ( 'NONE',  ( -1.551230140488696119, 1.386514373439803327, 0.4497748127911043725 ) ) ;
#79002=VECTOR ( 'NONE', #13535, 39.37007874015748143 ) ;
#79023=( CONVERSION_BASED_UNIT ( 'INCH', #15454 ) LENGTH_UNIT ( ) NAMED_UNIT ( #5085 ) );
#79032=FACE_OUTER_BOUND ( 'NONE', #37954, .T. ) ;
#79045=EDGE_CURVE ( 'NONE', #60812, #55552, #78342, .T. ) ;
#79061=ADVANCED_FACE ( 'NONE', ( #79182 ), #31449, .F. ) ;
#79064=AXIS2_PLACEMENT_3D ( 'NONE', #11762, #57163, #18070 ) ;
#79067=CARTESIAN_POINT ( 'NONE',  ( 2.630268417803937719, 1.724409448818898127, 0.4359958488159723644 ) ) ;
#79073=CARTESIAN_POINT ( 'NONE',  ( -3.831845081856512181, 2.755400581649067426, -0.5314960629921259283 ) ) ;
#79082=FACE_OUTER_BOUND ( 'NONE', #4954, .T. ) ;
#79084=VERTEX_POINT ( 'NONE', #40032 ) ;
#79102=ORIENTED_EDGE ( 'NONE', *, *, #9376, .T. ) ;
#79105=CARTESIAN_POINT ( 'NONE',  ( 2.856580783922613609, 1.081851677178490068, 0.1334749385307572034 ) ) ;
#79109=ADVANCED_FACE ( 'NONE', ( #1733 ), #53880, .F. ) ;
#79145=CARTESIAN_POINT ( 'NONE',  ( -1.852066570651491384, 1.064797240280318080, 0.04222672046130301199 ) ) ;
#79151=B_SPLINE_CURVE_WITH_KNOTS ( 'NONE', 3,
 ( #4348, #30015, #55678, #77552 ),
 .UNSPECIFIED., .F., .F.,
 ( 4, 4 ),
 ( 2.888536477662776634E-07, 0.001436607511248048788 ),
 .UNSPECIFIED. ) ;
#79163=CARTESIAN_POINT ( 'NONE',  ( 0.000000000000000000, 0.000000000000000000, -1.250000000000000000 ) ) ;
#79169=FACE_OUTER_BOUND ( 'NONE', #23910, .T. ) ;
#79170=EDGE_LOOP ( 'NONE', ( #43041, #72358 ) ) ;
#79177=CARTESIAN_POINT ( 'NONE',  ( 1.141392835773559211, 0.3937007874015748254, 1.456353465694822491 ) ) ;
#79181=FACE_OUTER_BOUND ( 'NONE', #2443, .T. ) ;
#79182=FACE_OUTER_BOUND ( 'NONE', #45819, .T. ) ;
#79185=ORIENTED_EDGE ( 'NONE', *, *, #47021, .T. ) ;
#79200=FACE_OUTER_BOUND ( 'NONE', #18108, .T. ) ;
#79218=CARTESIAN_POINT ( 'NONE',  ( 3.937007874015748143, 2.755905511811024056, -0.5314960629921260393 ) ) ;
#79223=CARTESIAN_POINT ( 'NONE',  ( 3.931500874951350255, 1.110937023017455783, 0.2101396702808374650 ) ) ;
#79226=CARTESIAN_POINT ( 'NONE',  ( 1.141392835773559211, 0.4110443821404751730, 1.141392835773562764 ) ) ;
#79240=CARTESIAN_POINT ( 'NONE',  ( -0.4744094488188934089, 1.537401574803149984, -1.016821367227985551 ) ) ;
#79256=CARTESIAN_POINT ( 'NONE',  ( -0.9285414500055708675, 0.000000000000000000, -0.6299212598425202314 ) ) ;
#79259=CARTESIAN_POINT ( 'NONE',  ( 0.4262708303801458487, 1.326867047802282373, 3.913881452109020831 ) ) ;
#79281=VERTEX_POINT ( 'NONE', #60213 ) ;
#79291=EDGE_CURVE ( 'NONE', #41808, #29808, #46234, .T. ) ;
#79293=CYLINDRICAL_SURFACE ( 'NONE', #26003, 0.5118110236220472231 ) ;
#79312=ORIENTED_EDGE ( 'NONE', *, *, #41641, .T. ) ;
#79315=CARTESIAN_POINT ( 'NONE',  ( 3.264097702071373064, 2.755905511811024056, -0.5314960629921260393 ) ) ;
#79322=ORIENTED_EDGE ( 'NONE', *, *, #76828, .F. ) ;
#79326=DIRECTION ( 'NONE',  ( 0.000000000000000000, -0.000000000000000000, 1.000000000000000000 ) ) ;
#79327=DIRECTION ( 'NONE',  ( 0.000000000000000000, -1.734723475976808327E-16, 1.000000000000000000 ) ) ;
#79389=LINE ( 'NONE', #33513, #77479 ) ;
#79391=EDGE_LOOP ( 'NONE', ( #22148, #44129, #50695, #7396, #77720, #40858, #5448 ) ) ;
#79397=DIRECTION ( 'NONE',  ( 0.000000000000000000, 0.000000000000000000, 1.000000000000000000 ) ) ;
#79402=AXIS2_PLACEMENT_3D ( 'NONE', #31446, #44473, #70164 ) ;
#79408=ORIENTED_EDGE ( 'NONE', *, *, #58809, .F. ) ;
#79411=CARTESIAN_POINT ( 'NONE',  ( -1.568139075118781589, 1.385950145841912118, 0.4495859454777829112 ) ) ;
#79425=EDGE_LOOP ( 'NONE', ( #19558, #3624, #51114, #67499 ) ) ;
#79431=CARTESIAN_POINT ( 'NONE',  ( 2.139067083128515900, 1.422987107291906694, -0.4606739315415588898 ) ) ;
#79432=EDGE_CURVE ( 'NONE', #14187, #5989, #31857, .T. ) ;
#79439=CARTESIAN_POINT ( 'NONE',  ( 0.000000000000000000, 0.000000000000000000, 0.000000000000000000 ) ) ;
#79452=EDGE_CURVE ( 'NONE', #39742, #80735, #13343, .T. ) ;
#79456=EDGE_CURVE ( 'NONE', #57006, #41276, #78159, .T. ) ;
#79457=DIRECTION ( 'NONE',  ( -0.000000000000000000, 1.000000000000000000, -0.000000000000000000 ) ) ;
#79459=FACE_BOUND ( 'NONE', #69943, .T. ) ;
#79495=ORIENTED_EDGE ( 'NONE', *, *, #10296, .F. ) ;
#79510=ORIENTED_EDGE ( 'NONE', *, *, #8432, .T. ) ;
#79514=ADVANCED_BREP_SHAPE_REPRESENTATION ( '', ( #33697, #22098 ), #5981 ) ;
#79531=ORIENTED_EDGE ( 'NONE', *, *, #25250, .F. ) ;
#79536=EDGE_CURVE ( 'NONE', #40470, #32861, #64423, .T. ) ;
#79552=DIRECTION ( 'NONE',  ( 0.000000000000000000, 0.000000000000000000, 1.000000000000000000 ) ) ;
#79558=CARTESIAN_POINT ( 'NONE',  ( 0.5314960629920852941, 2.716724272663528783, 3.890406373195420375 ) ) ;
#79583=CARTESIAN_POINT ( 'NONE',  ( -0.9881811337016640495, 0.000000000000000000, -0.5314960629921260393 ) ) ;
#79587=AXIS2_PLACEMENT_3D ( 'NONE', #49322, #48491, #56044 ) ;
#79591=DIRECTION ( 'NONE',  ( 0.000000000000000000, -1.000000000000000000, 0.000000000000000000 ) ) ;
#79602=ORIENTED_EDGE ( 'NONE', *, *, #41314, .T. ) ;
#79621=EDGE_LOOP ( 'NONE', ( #34046, #40672, #56675, #51798 ) ) ;
#79638=CARTESIAN_POINT ( 'NONE',  ( 3.926431222168898838, 1.160582578298199108, 0.2886442948464663094 ) ) ;
#79642=FACE_OUTER_BOUND ( 'NONE', #98, .T. ) ;
#79648=DIRECTION ( 'NONE',  ( 1.000000000000000000, -0.000000000000000000, 3.491481338843132961E-15 ) ) ;
#79654=AXIS2_PLACEMENT_3D ( 'NONE', #59059, #40538, #28315 ) ;
#79658=CYLINDRICAL_SURFACE ( 'NONE', #73986, 0.2165354330708660624 ) ;
#79690=DIRECTION ( 'NONE',  ( 0.000000000000000000, 0.000000000000000000, 1.000000000000000000 ) ) ;
#79702=CYLINDRICAL_SURFACE ( 'NONE', #66851, 0.4744094488188972947 ) ;
#79711=DIRECTION ( 'NONE',  ( 0.000000000000000000, 1.000000000000000000, -0.000000000000000000 ) ) ;
#79725=CARTESIAN_POINT ( 'NONE',  ( -0.2887997841774402885, 1.160717306711473107, -2.785006778007305783 ) ) ;
#79729=EDGE_LOOP ( 'NONE', ( #805, #17938, #34346, #53798, #46161, #34898, #17871, #41613, #31008, #66865, #30527, #20275, #65026, #51801, #25967, #59176, #24695, #77415, #81176, #81851, #24641, #22990, #78898, #66148, #24924, #294, #26892, #22166, #37657, #27411, #12944, #1866, #8790, #24726, #35091, #60649 ) ) ;
#79730=VERTEX_POINT ( 'NONE', #16267 ) ;
#79733=DIRECTION ( 'NONE',  ( 0.000000000000000000, 1.000000000000000000, -0.000000000000000000 ) ) ;
#79742=ORIENTED_EDGE ( 'NONE', *, *, #81513, .F. ) ;
#79744=CARTESIAN_POINT ( 'NONE',  ( -1.016821367227983774, 1.505793896356053096, 0.4744094488188971281 ) ) ;
#79746=LINE ( 'NONE', #59113, #47932 ) ;
#79749=CARTESIAN_POINT ( 'NONE',  ( 0.4177787735907000366, 0.3937007874015748254, -1.559171609364239375 ) ) ;
#79757=CONICAL_SURFACE ( 'NONE', #27277, 0.09842519685039351207, 1.029744258676651647 ) ;
#79768=EDGE_CURVE ( 'NONE', #40586, #78998, #28766, .T. ) ;
#79813=VERTEX_POINT ( 'NONE', #41912 ) ;
#79814=ORIENTED_EDGE ( 'NONE', *, *, #7406, .T. ) ;
#79816=CONICAL_SURFACE ( 'NONE', #8550, 1.889763779527559251, 0.7853981633974500554 ) ;
#79834=CARTESIAN_POINT ( 'NONE',  ( -2.142213561789869658, 0.02617651024168207372, -0.4623158380715769455 ) ) ;
#79838=CARTESIAN_POINT ( 'NONE',  ( 1.033875059083676717, 1.724409448818897905, -0.4359958488159719758 ) ) ;
#79848=CARTESIAN_POINT ( 'NONE',  ( 0.5314960629921395840, 2.677165354330708791, -3.900966923095588346 ) ) ;
#79861=CARTESIAN_POINT ( 'NONE',  ( -0.4744094488189058989, 1.554943921348593161, 2.554262525012261253 ) ) ;
#79867=CIRCLE ( 'NONE', #18020, 2.204724409448819422 ) ;
#79879=CONICAL_SURFACE ( 'NONE', #34134, 2.559055118110236560, 0.7853981633974500554 ) ;
#79901=B_SPLINE_CURVE_WITH_KNOTS ( 'NONE', 3,
 ( #7412, #32656, #64235, #26341, #71385, #13734, #7836, #52002 ),
 .UNSPECIFIED., .F., .F.,
 ( 4, 2, 2, 4 ),
 ( 0.07134069304684192980, 0.07377942048615132586, 0.07499878420580601002, 0.07621814792546070805 ),
 .UNSPECIFIED. ) ;
#79905=EDGE_CURVE ( 'NONE', #31620, #3191, #40673, .T. ) ;
#79914=ORIENTED_EDGE ( 'NONE', *, *, #15570, .F. ) ;
#79927=EDGE_CURVE ( 'NONE', #70474, #27584, #53290, .T. ) ;
#79930=ORIENTED_EDGE ( 'NONE', *, *, #68219, .F. ) ;
#79932=ORIENTED_EDGE ( 'NONE', *, *, #46613, .F. ) ;
#79935=DIRECTION ( 'NONE',  ( 0.000000000000000000, 0.000000000000000000, 1.000000000000000000 ) ) ;
#79948=ORIENTED_EDGE ( 'NONE', *, *, #56687, .F. ) ;
#79951=ORIENTED_EDGE ( 'NONE', *, *, #77984, .T. ) ;
#79972=LINE ( 'NONE', #47946, #50653 ) ;
#79977=CARTESIAN_POINT ( 'NONE',  ( -1.939486441909048509, 1.160811571118562702, -0.2889173282905337925 ) ) ;
#80001=AXIS2_PLACEMENT_3D ( 'NONE', #31767, #623, #64589 ) ;
#80005=ORIENTED_EDGE ( 'NONE', *, *, #22645, .T. ) ;
#80018=ORIENTED_EDGE ( 'NONE', *, *, #71612, .T. ) ;
#80024=CARTESIAN_POINT ( 'NONE',  ( 0.04801148344178311073, 1.065401592510863971, -1.490017649659075571 ) ) ;
#80032=ORIENTED_EDGE ( 'NONE', *, *, #79536, .F. ) ;
#80035=ORIENTED_EDGE ( 'NONE', *, *, #59891, .F. ) ;
#80056=VECTOR ( 'NONE', #5108, 39.37007874015748143 ) ;
#80061=EDGE_CURVE ( 'NONE', #64262, #6368, #62345, .T. ) ;
#80065=CARTESIAN_POINT ( 'NONE',  ( 0.3149606299212737159, 2.165354330708661568, -3.924389226575467404 ) ) ;
#80068=EDGE_CURVE ( 'NONE', #78176, #27965, #36410, .T. ) ;
#80073=CARTESIAN_POINT ( 'NONE',  ( -0.2120393137889660107, 1.111861684530155658, -1.102218936792509485 ) ) ;
#80088=DIRECTION ( 'NONE',  ( 1.000000000000000000, -0.000000000000000000, -0.000000000000000000 ) ) ;
#80092=LINE ( 'NONE', #9368, #54765 ) ;
#80096=EDGE_CURVE ( 'NONE', #67621, #57422, #42735, .T. ) ;
#80105=FACE_BOUND ( 'NONE', #4225, .T. ) ;
#80109=AXIS2_PLACEMENT_3D ( 'NONE', #66682, #79733, #27113 ) ;
#80141=CARTESIAN_POINT ( 'NONE',  ( -0.08529443231573714812, 1.070420337342310235, -2.867136178046102657 ) ) ;
#80151=AXIS2_PLACEMENT_3D ( 'NONE', #68366, #35956, #10704 ) ;
#80153=DIRECTION ( 'NONE',  ( 0.000000000000000000, 0.000000000000000000, -1.000000000000000000 ) ) ;
#80154=CARTESIAN_POINT ( 'NONE',  ( 0.4177787735907000921, 0.3937007874015748254, -1.244210979442979648 ) ) ;
#80165=PLANE ( 'NONE',  #43886 ) ;
#80171=AXIS2_PLACEMENT_3D ( 'NONE', #48143, #9437, #9854 ) ;
#80198=CARTESIAN_POINT ( 'NONE',  ( 0.4257672537616556951, 1.326168777627702244, 2.077356831852779528 ) ) ;
#80203=ORIENTED_EDGE ( 'NONE', *, *, #10428, .T. ) ;
#80218=DIRECTION ( 'NONE',  ( -0.000000000000000000, 1.000000000000000000, -0.000000000000000000 ) ) ;
#80249=ORIENTED_EDGE ( 'NONE', *, *, #38804, .F. ) ;
#80251=VERTEX_POINT ( 'NONE', #12006 ) ;
#80252=CARTESIAN_POINT ( 'NONE',  ( -1.708538945418524024, 1.316053703249684625, 0.4200579243588399292 ) ) ;
#80265=CARTESIAN_POINT ( 'NONE',  ( 0.5314960629921394730, 2.745602313593968891, -3.861135848600277143 ) ) ;
#80273=CIRCLE ( 'NONE', #13075, 0.5118110236220472231 ) ;
#80309=DIRECTION ( 'NONE',  ( -3.491481338843132961E-15, -0.000000000000000000, 1.000000000000000000 ) ) ;
#80325=AXIS2_PLACEMENT_3D ( 'NONE', #62709, #74942, #62286 ) ;
#80328=ORIENTED_EDGE ( 'NONE', *, *, #55345, .F. ) ;
#80330=VERTEX_POINT ( 'NONE', #55364 ) ;
#80344=VERTEX_POINT ( 'NONE', #68431 ) ;
#80346=ORIENTED_EDGE ( 'NONE', *, *, #28821, .T. ) ;
#80349=LINE ( 'NONE', #42010, #40802 ) ;
#80360=ORIENTED_EDGE ( 'NONE', *, *, #5158, .T. ) ;
#80362=CARTESIAN_POINT ( 'NONE',  ( -0.9285414500055713116, 2.165354330708661568, 0.6299212598425196763 ) ) ;
#80389=CIRCLE ( 'NONE', #30603, 3.444881889763779625 ) ;
#80391=CARTESIAN_POINT ( 'NONE',  ( -1.877095671717788683, 1.091897865355345720, -0.1662078246829333805 ) ) ;
#80421=CARTESIAN_POINT ( 'NONE',  ( 0.2628095437103130094, 1.142422500371641059, -1.473052246231814744 ) ) ;
#80424=DIRECTION ( 'NONE',  ( 0.000000000000000000, 0.000000000000000000, -1.000000000000000000 ) ) ;
#80427=CARTESIAN_POINT ( 'NONE',  ( 0.3149606299212641680, 5.463695987328538763E-17, -1.076935383196056195 ) ) ;
#80434=EDGE_LOOP ( 'NONE', ( #49052, #61693, #81261, #82999 ) ) ;
#80440=CARTESIAN_POINT ( 'NONE',  ( 0.000000000000000000, 0.000000000000000000, -2.362204724409448620 ) ) ;
#80445=CARTESIAN_POINT ( 'NONE',  ( 0.3005662378122966882, 1.170051713876984811, -2.776705245712382641 ) ) ;
#80448=ORIENTED_EDGE ( 'NONE', *, *, #62891, .T. ) ;
#80451=ORIENTED_EDGE ( 'NONE', *, *, #51722, .T. ) ;
#80484=CARTESIAN_POINT ( 'NONE',  ( -0.4497599300473023587, 1.383355012730091538, -1.028042735862942259 ) ) ;
#80504=EDGE_CURVE ( 'NONE', #45375, #53039, #37660, .T. ) ;
#80516=DIRECTION ( 'NONE',  ( 0.000000000000000000, -8.326672684688674053E-16, 1.000000000000000000 ) ) ;
#80556=CARTESIAN_POINT ( 'NONE',  ( -0.4744094488188880243, 1.528817788452848880, -2.554262525012306551 ) ) ;
#80559=EDGE_CURVE ( 'NONE', #74865, #27710, #23416, .T. ) ;
#80561=EDGE_LOOP ( 'NONE', ( #2982, #8773 ) ) ;
#80566=PLANE ( 'NONE',  #4856 ) ;
#80568=LINE ( 'NONE', #22879, #74639 ) ;
#80569=FACE_OUTER_BOUND ( 'NONE', #70488, .T. ) ;
#80571=ADVANCED_FACE ( 'NONE', ( #55774 ), #81481, .F. ) ;
#80578=CARTESIAN_POINT ( 'NONE',  ( -1.063838992779605919, 1.224418437586606290, 0.3568528392778475000 ) ) ;
#80583=EDGE_CURVE ( 'NONE', #33327, #62412, #73118, .T. ) ;
#80593=CARTESIAN_POINT ( 'NONE',  ( -0.5314960629921127166, 2.755905511811024056, -3.821484228344195433 ) ) ;
#80611=CARTESIAN_POINT ( 'NONE',  ( 0.08520949344211689591, 1.070405622666593226, 1.857259653016817280 ) ) ;
#80616=EDGE_LOOP ( 'NONE', ( #13430, #24382, #47994, #27396 ) ) ;
#80620=CARTESIAN_POINT ( 'NONE',  ( -2.165487897237678538, 1.580736828574222264, -0.4725026149319441759 ) ) ;
#80626=EDGE_CURVE ( 'NONE', #58460, #41616, #81231, .T. ) ;
#80648=FACE_OUTER_BOUND ( 'NONE', #47762, .T. ) ;
#80667=CARTESIAN_POINT ( 'NONE',  ( -0.4744094488189058989, 1.537401574803149984, 2.554262525012261253 ) ) ;
#80678=DIRECTION ( 'NONE',  ( 0.000000000000000000, 0.000000000000000000, -1.000000000000000000 ) ) ;
#80680=CARTESIAN_POINT ( 'NONE',  ( 2.170146923806635098, 1.528780496884629025, -0.4744094488188970171 ) ) ;
#80686=DIRECTION ( 'NONE',  ( 0.000000000000000000, -1.000000000000000000, 0.000000000000000000 ) ) ;
#80687=B_SPLINE_CURVE_WITH_KNOTS ( 'NONE', 3,
 ( #46288, #59338, #53012, #78726, #46710, #37182, #30862, #47120, #15158, #40816, #21462, #34928, #66500, #14751 ),
 .UNSPECIFIED., .F., .F.,
 ( 4, 2, 2, 2, 2, 2, 4 ),
 ( 0.000000000000000000, 0.0003923887041693433029, 0.0007847774083386866058, 0.001177166112508029909, 0.001569554816677373212, 0.002354332225016059817, 0.003139109633354746423 ),
 .UNSPECIFIED. ) ;
#80719=ADVANCED_FACE ( 'NONE', ( #63748 ), #7772, .F. ) ;
#80735=VERTEX_POINT ( 'NONE', #77216 ) ;
#80751=VERTEX_POINT ( 'NONE', #6087 ) ;
#80754=DIRECTION ( 'NONE',  ( 0.000000000000000000, 0.000000000000000000, -1.000000000000000000 ) ) ;
#80760=CARTESIAN_POINT ( 'NONE',  ( 0.4613966517175972504, 1.648900267337816139, 1.022797972794818655 ) ) ;
#80765=ORIENTED_EDGE ( 'NONE', *, *, #77818, .F. ) ;
#80789=DIRECTION ( 'NONE',  ( 0.8660254037844361541, 0.000000000000000000, 0.5000000000000043299 ) ) ;
#80794=CARTESIAN_POINT ( 'NONE',  ( -1.851299440327907941, 1.063968899401423140, -0.03484477857459079841 ) ) ;
#80821=DIRECTION ( 'NONE',  ( -0.000000000000000000, -1.000000000000000000, -0.000000000000000000 ) ) ;
#80833=B_SPLINE_CURVE_WITH_KNOTS ( 'NONE', 3,
 ( #54416, #48515, #60739, #36308, #17390, #48932, #29578, #61574 ),
 .UNSPECIFIED., .F., .F.,
 ( 4, 2, 2, 4 ),
 ( 0.07055950480717279594, 0.07177139162174094034, 0.07298327843630908474, 0.07540705206544540129 ),
 .UNSPECIFIED. ) ;
#80838=ORIENTED_EDGE ( 'NONE', *, *, #48541, .T. ) ;
#80846=AXIS2_PLACEMENT_3D ( 'NONE', #11768, #31511, #58004 ) ;
#80850=PLANE ( 'NONE',  #51917 ) ;
#80854=ORIENTED_EDGE ( 'NONE', *, *, #80976, .T. ) ;
#80905=VECTOR ( 'NONE', #69155, 39.37007874015748143 ) ;
#80908=LINE ( 'NONE', #54797, #22227 ) ;
#80923=CARTESIAN_POINT ( 'NONE',  ( -1.720695750894368548, 1.210707077873740767, 0.3442465688542959978 ) ) ;
#80925=DIRECTION ( 'NONE',  ( 0.000000000000000000, 0.000000000000000000, -1.000000000000000000 ) ) ;
#80926=DIRECTION ( 'NONE',  ( 0.000000000000000000, 0.000000000000000000, 1.000000000000000000 ) ) ;
#80938=CARTESIAN_POINT ( 'NONE',  ( 0.4359958488159758616, 1.724409448818897905, -1.033875059083675163 ) ) ;
#80939=EDGE_CURVE ( 'NONE', #27190, #80251, #79867, .T. ) ;
#80947=EDGE_CURVE ( 'NONE', #46125, #46648, #54431, .T. ) ;
#80965=LINE ( 'NONE', #22044, #11698 ) ;
#80969=EDGE_CURVE ( 'NONE', #29808, #41808, #54289, .T. ) ;
#80970=VERTEX_POINT ( 'NONE', #30001 ) ;
#80976=EDGE_CURVE ( 'NONE', #36503, #41297, #61588, .T. ) ;
#80978=LINE ( 'NONE', #4757, #80905 ) ;
#80985=CARTESIAN_POINT ( 'NONE',  ( -1.024202178938476981, 1.413766264023041730, 0.4582849312594932667 ) ) ;
#80990=DIRECTION ( 'NONE',  ( -0.8660254037844431485, 0.000000000000000000, 0.4999999999999918954 ) ) ;
#80993=CARTESIAN_POINT ( 'NONE',  ( -3.908806514029711021, 1.601083746178882938, -0.4703884258841616872 ) ) ;
#81007=DIRECTION ( 'NONE',  ( 0.000000000000000000, 0.000000000000000000, -1.000000000000000000 ) ) ;
#81020=VECTOR ( 'NONE', #64814, 39.37007874015748143 ) ;
#81022=CARTESIAN_POINT ( 'NONE',  ( 0.4744094488188898562, 1.528788477448867811, 2.170146923806596462 ) ) ;
#81028=EDGE_CURVE ( 'NONE', #32917, #44550, #61454, .T. ) ;
#81031=CARTESIAN_POINT ( 'NONE',  ( -1.313877454013331780, 0.2755905511811023723, 0.7983292792091805090 ) ) ;
#81040=DIRECTION ( 'NONE',  ( 0.000000000000000000, 0.000000000000000000, 1.000000000000000000 ) ) ;
#81056=CARTESIAN_POINT ( 'NONE',  ( 0.3149606299212736604, 2.559055118110236560, -3.937007874015761022 ) ) ;
#81074=DIRECTION ( 'NONE',  ( -3.491481338843132961E-15, -0.000000000000000000, 1.000000000000000000 ) ) ;
#81075=DIRECTION ( 'NONE',  ( 0.000000000000000000, -1.000000000000000000, 0.000000000000000000 ) ) ;
#81092=CARTESIAN_POINT ( 'NONE',  ( 0.5314960629921061663, 2.755905511811024056, 1.895394334970797345 ) ) ;
#81099=EDGE_CURVE ( 'NONE', #26979, #45807, #39579, .T. ) ;
#81176=ORIENTED_EDGE ( 'NONE', *, *, #59446, .T. ) ;
#81178=CARTESIAN_POINT ( 'NONE',  ( -0.5314960629921170465, 2.729656594508716783, -2.556891439663424581 ) ) ;
#81185=FACE_OUTER_BOUND ( 'NONE', #19206, .T. ) ;
#81194=EDGE_CURVE ( 'NONE', #24806, #34044, #37558, .T. ) ;
#81195=AXIS2_PLACEMENT_3D ( 'NONE', #55887, #4145, #36132 ) ;
#81206=CARTESIAN_POINT ( 'NONE',  ( -2.104898677616466429, 1.365902157108392245, 0.4425616331406720394 ) ) ;
#81214=CARTESIAN_POINT ( 'NONE',  ( 0.000000000000000000, 0.4374015748031496176, -1.178877988035069047 ) ) ;
#81223=CYLINDRICAL_SURFACE ( 'NONE', #22569, 0.3149606299212598381 ) ;
#81231=CIRCLE ( 'NONE', #58303, 3.937007874015748143 ) ;
#81239=DIRECTION ( 'NONE',  ( 9.381338752702732014E-17, -0.6427876096865392519, 0.7660444431189781245 ) ) ;
#81257=CARTESIAN_POINT ( 'NONE',  ( 0.4177787735907000366, 0.000000000000000000, -1.559171609364239375 ) ) ;
#81261=ORIENTED_EDGE ( 'NONE', *, *, #22702, .T. ) ;
#81294=DIRECTION ( 'NONE',  ( 1.000000000000000000, 1.601283208593976204E-15, 0.000000000000000000 ) ) ;
#81295=AXIS2_PLACEMENT_3D ( 'NONE', #57311, #69141, #50585 ) ;
#81302=CARTESIAN_POINT ( 'NONE',  ( -2.800715669567006127, 1.143166703770576387, 0.2643333500026571192 ) ) ;
#81312=VECTOR ( 'NONE', #3530, 39.37007874015748143 ) ;
#81319=CARTESIAN_POINT ( 'NONE',  ( 0.3230994083235798064, 1.189706270649605768, -1.965018580821014993 ) ) ;
#81343=ORIENTED_EDGE ( 'NONE', *, *, #59409, .T. ) ;
#81360=DIRECTION ( 'NONE',  ( -0.000000000000000000, -1.000000000000000000, -0.000000000000000000 ) ) ;
#81374=CARTESIAN_POINT ( 'NONE',  ( 0.000000000000000000, 0.03937007874015747977, 0.000000000000000000 ) ) ;
#81376=CARTESIAN_POINT ( 'NONE',  ( -1.313877454013331780, 1.062992125984252079, 0.7983292792091805090 ) ) ;
#81379=VERTEX_POINT ( 'NONE', #59411 ) ;
#81383=CARTESIAN_POINT ( 'NONE',  ( 2.154527559055120278, 0.03937007874015747977, -0.4677827689124846589 ) ) ;
#81384=DIRECTION ( 'NONE',  ( -0.000000000000000000, -1.000000000000000000, -0.000000000000000000 ) ) ;
#81403=DIRECTION ( 'NONE',  ( 0.000000000000000000, 0.000000000000000000, 1.000000000000000000 ) ) ;
#81410=DIRECTION ( 'NONE',  ( -0.000000000000000000, 1.000000000000000000, -0.000000000000000000 ) ) ;
#81419=CARTESIAN_POINT ( 'NONE',  ( 0.4324858057354169505, 1.341834121656384715, -1.665041785426940368 ) ) ;
#81437=ORIENTED_EDGE ( 'NONE', *, *, #80583, .F. ) ;
#81450=CARTESIAN_POINT ( 'NONE',  ( -0.4744094488189005143, 1.537401574803149984, 1.016821367227982220 ) ) ;
#81480=ORIENTED_EDGE ( 'NONE', *, *, #22453, .F. ) ;
#81481=PLANE ( 'NONE',  #70444 ) ;
#81487=PLANE ( 'NONE',  #30211 ) ;
#81496=ORIENTED_EDGE ( 'NONE', *, *, #16301, .T. ) ;
#81500=CARTESIAN_POINT ( 'NONE',  ( 2.103514684735005247, 1.710972922415816999, 0.4417590601942928408 ) ) ;
#81513=EDGE_CURVE ( 'NONE', #49988, #34953, #14412, .T. ) ;
#81518=CIRCLE ( 'NONE', #39801, 3.937007874015748143 ) ;
#81528=CARTESIAN_POINT ( 'NONE',  ( -3.896872718254346779, 2.702643891907236640, 0.5314960629921260393 ) ) ;
#81544=B_SPLINE_CURVE_WITH_KNOTS ( 'NONE', 3,
 ( #41170, #33612, #8771, #59688, #72746, #60114, #66861, #20574, #2043, #2874, #39932, #72338, #60525, #8360, #34027, #21399 ),
 .UNSPECIFIED., .F., .F.,
 ( 4, 2, 2, 2, 2, 2, 2, 4 ),
 ( 0.000000000000000000, 0.0003923911760484627724, 0.0007847823520969255447, 0.001177173528145388209, 0.001569564704193851089, 0.001961955880242313970, 0.002354347056290776417, 0.003139129408387686133 ),
 .UNSPECIFIED. ) ;
#81560=EDGE_LOOP ( 'NONE', ( #76876, #79102, #44256, #5786 ) ) ;
#81578=AXIS2_PLACEMENT_3D ( 'NONE', #41404, #15750, #67086 ) ;
#81579=CIRCLE ( 'NONE', #13012, 0.01968503937007875723 ) ;
#81585=DIRECTION ( 'NONE',  ( -0.000000000000000000, -1.000000000000000000, -0.000000000000000000 ) ) ;
#81587=CARTESIAN_POINT ( 'NONE',  ( 3.224202737261815166, 2.716535433070866645, 0.5314960629921260393 ) ) ;
#81591=CARTESIAN_POINT ( 'NONE',  ( 3.920840774341704638, 1.223555610140524941, 0.3571001360657545254 ) ) ;
#81593=ORIENTED_EDGE ( 'NONE', *, *, #81194, .T. ) ;
#81596=ORIENTED_EDGE ( 'NONE', *, *, #66936, .F. ) ;
#81598=CARTESIAN_POINT ( 'NONE',  ( 5.333846858410640380E-15, 1.062992125984252079, -1.444810848096780953 ) ) ;
#81602=EDGE_CURVE ( 'NONE', #46245, #11181, #48415, .T. ) ;
#81635=CONICAL_SURFACE ( 'NONE', #77597, 0.1190944881889763746, 0.8726646259971653219 ) ;
#81638=AXIS2_PLACEMENT_3D ( 'NONE', #18049, #29829, #80789 ) ;
#81650=ORIENTED_EDGE ( 'NONE', *, *, #32101, .F. ) ;
#81659=CARTESIAN_POINT ( 'NONE',  ( 0.5314960629920989499, 2.755905511811024056, 2.583694225513486042 ) ) ;
#81664=ORIENTED_EDGE ( 'NONE', *, *, #49134, .F. ) ;
#81667=ORIENTED_EDGE ( 'NONE', *, *, #30238, .F. ) ;
#81681=ORIENTED_EDGE ( 'NONE', *, *, #302, .T. ) ;
#81684=ORIENTED_EDGE ( 'NONE', *, *, #47141, .F. ) ;
#81702=CIRCLE ( 'NONE', #9118, 0.5118110236220471121 ) ;
#81711=CARTESIAN_POINT ( 'NONE',  ( -3.224202737261815166, 2.716535433070866645, -0.5314960629921260393 ) ) ;
#81714=CARTESIAN_POINT ( 'NONE',  ( -3.937007874015748143, 2.755905511811024056, 0.5314960629921260393 ) ) ;
#81717=CARTESIAN_POINT ( 'NONE',  ( -2.571327113428939715, 1.453547212638086172, 0.4672029448317639444 ) ) ;
#81720=CARTESIAN_POINT ( 'NONE',  ( -0.08327261094992825796, 1.070339138594046835, -1.465778323607621392 ) ) ;
#81725=CARTESIAN_POINT ( 'NONE',  ( -1.313877454013331780, 1.062992125984252079, 0.6999040823587869831 ) ) ;
#81730=CARTESIAN_POINT ( 'NONE',  ( 0.2895113455958823745, 1.161258846611464834, -1.084123980916873231 ) ) ;
#81734=CARTESIAN_POINT ( 'NONE',  ( 0.4744094488189052328, 1.537401574803149984, -2.170146923806634653 ) ) ;
#81751=PLANE ( 'NONE',  #31176 ) ;
#81755=VECTOR ( 'NONE', #64746, 39.37007874015748143 ) ;
#81775=DIRECTION ( 'NONE',  ( -0.000000000000000000, 1.000000000000000000, -0.000000000000000000 ) ) ;
#81792=CARTESIAN_POINT ( 'NONE',  ( 3.908418136489574923, 1.569398530225769139, -0.4736046740121441778 ) ) ;
#81795=ORIENTED_EDGE ( 'NONE', *, *, #13007, .F. ) ;
#81800=DIRECTION ( 'NONE',  ( 1.047444401652940007E-14, -0.000000000000000000, -1.000000000000000000 ) ) ;
#81815=B_SPLINE_CURVE_WITH_KNOTS ( 'NONE', 3,
 ( #10697, #24129, #67112, #80993, #54881, #11104, #49798, #49391 ),
 .UNSPECIFIED., .F., .F.,
 ( 4, 2, 2, 4 ),
 ( 0.04257512569008879699, 0.04378708032589691268, 0.04499903496170502837, 0.04742294423332127362 ),
 .UNSPECIFIED. ) ;
#81847=CARTESIAN_POINT ( 'NONE',  ( 0.06850640440391080055, 1.067651707476381606, 1.854710246793788819 ) ) ;
#81851=ORIENTED_EDGE ( 'NONE', *, *, #59902, .T. ) ;
#81864=CARTESIAN_POINT ( 'NONE',  ( -1.840815010931731832, 2.729664643556220849, -0.5314960629921260393 ) ) ;
#81882=CARTESIAN_POINT ( 'NONE',  ( -3.924389226575468737, 2.165354330708661568, -0.3149606299212600047 ) ) ;
#81892=ORIENTED_EDGE ( 'NONE', *, *, #79905, .F. ) ;
#81894=ORIENTED_EDGE ( 'NONE', *, *, #18320, .F. ) ;
#81918=ORIENTED_EDGE ( 'NONE', *, *, #33182, .F. ) ;
#81949=DIRECTION ( 'NONE',  ( 0.000000000000000000, 0.000000000000000000, -1.000000000000000000 ) ) ;
#81954=CARTESIAN_POINT ( 'NONE',  ( 0.2472359589189098705, 1.132503624486270066, -1.510687062895181398 ) ) ;
#81969=ORIENTED_EDGE ( 'NONE', *, *, #16168, .F. ) ;
#81989=DIRECTION ( 'NONE',  ( 0.000000000000000000, 1.000000000000000000, 0.000000000000000000 ) ) ;
#81993=CARTESIAN_POINT ( 'NONE',  ( -0.4712111919743346422, 1.601159491416950242, -3.908712531853713479 ) ) ;
#81999=CARTESIAN_POINT ( 'NONE',  ( 3.937010599584712001, 1.062969507148802562, 0.03102431951651077324 ) ) ;
#82010=CARTESIAN_POINT ( 'NONE',  ( -0.07763727620476214286, 1.069130918477190662, 3.936271712427351854 ) ) ;
#82019=EDGE_CURVE ( 'NONE', #2910, #6386, #71852, .T. ) ;
#82030=CARTESIAN_POINT ( 'NONE',  ( 0.5314960629920990609, 2.742780008954323279, 2.570293882282747688 ) ) ;
#82038=CARTESIAN_POINT ( 'NONE',  ( 0.000000000000000000, 2.559055118110236560, 0.000000000000000000 ) ) ;
#82050=CARTESIAN_POINT ( 'NONE',  ( -3.927314176868121898, 1.151522056532830796, -0.2764061900857891496 ) ) ;
#82055=ORIENTED_EDGE ( 'NONE', *, *, #77836, .T. ) ;
#82069=VERTEX_POINT ( 'NONE', #12436 ) ;
#82082=EDGE_CURVE ( 'NONE', #11714, #34573, #82597, .T. ) ;
#82117=VECTOR ( 'NONE', #59785, 39.37007874015748143 ) ;
#82124=CARTESIAN_POINT ( 'NONE',  ( -0.5314960629921324786, 2.716535433070866645, 1.854472803289050509 ) ) ;
#82137=EDGE_CURVE ( 'NONE', #53393, #72873, #23826, .T. ) ;
#82139=CARTESIAN_POINT ( 'NONE',  ( 0.4744094488189051773, 1.528817788452848880, -2.170146923806634209 ) ) ;
#82144=DIRECTION ( 'NONE',  ( 0.000000000000000000, -1.000000000000000000, 0.000000000000000000 ) ) ;
#82149=DIRECTION ( 'NONE',  ( 0.000000000000000000, 1.000000000000000000, 0.000000000000000000 ) ) ;
#82166=ORIENTED_EDGE ( 'NONE', *, *, #46764, .F. ) ;
#82173=AXIS2_PLACEMENT_3D ( 'NONE', #8926, #9752, #34603 ) ;
#82182=CARTESIAN_POINT ( 'NONE',  ( -0.2248141966262267588, 1.118402650174327384, -1.901317244778563342 ) ) ;
#82186=ORIENTED_EDGE ( 'NONE', *, *, #45702, .T. ) ;
#82198=CARTESIAN_POINT ( 'NONE',  ( 0.000000000000000000, 1.724409448818897461, 0.000000000000000000 ) ) ;
#82202=ORIENTED_EDGE ( 'NONE', *, *, #73105, .F. ) ;
#82205=LINE ( 'NONE', #10677, #14876 ) ;
#82206=CARTESIAN_POINT ( 'NONE',  ( -0.4744094488189045666, 1.537401574803149984, 2.170146923806632877 ) ) ;
#82215=CIRCLE ( 'NONE', #78014, 2.598425196850393970 ) ;
#82225=CARTESIAN_POINT ( 'NONE',  ( -0.4698424923132972220, 1.469648236684816256, 2.159177592673387824 ) ) ;
#82229=EDGE_CURVE ( 'NONE', #38768, #312, #16765, .T. ) ;
#82240=CARTESIAN_POINT ( 'NONE',  ( 1.115278074387389351, 1.079212911816122888, -0.1239772976664039461 ) ) ;
#82287=LINE ( 'NONE', #81056, #41037 ) ;
#82297=ORIENTED_EDGE ( 'NONE', *, *, #58451, .F. ) ;
#82300=DIRECTION ( 'NONE',  ( 0.000000000000000000, -1.000000000000000000, 1.408710688920637755E-15 ) ) ;
#82304=DIRECTION ( 'NONE',  ( -0.000000000000000000, -1.000000000000000000, -0.000000000000000000 ) ) ;
#82305=CARTESIAN_POINT ( 'NONE',  ( 0.000000000000000000, 2.559055118110236560, 0.000000000000000000 ) ) ;
#82306=CARTESIAN_POINT ( 'NONE',  ( 1.076935383196057749, 2.165354330708661568, -0.3149606299212595606 ) ) ;
#82315=DIRECTION ( 'NONE',  ( -0.000000000000000000, 1.000000000000000000, -0.000000000000000000 ) ) ;
#82317=CARTESIAN_POINT ( 'NONE',  ( 3.924389226575468737, 2.165354330708661568, 0.3149606299212600047 ) ) ;
#82323=DIRECTION ( 'NONE',  ( 1.000000000000000000, 1.460819769243627131E-15, 0.000000000000000000 ) ) ;
#82357=CIRCLE ( 'NONE', #46045, 0.3149606299212597826 ) ;
#82362=CARTESIAN_POINT ( 'NONE',  ( 0.2492877267040487788, 1.133758322672524743, -1.503986617498455303 ) ) ;
#82375=VERTEX_POINT ( 'NONE', #81092 ) ;
#82416=CARTESIAN_POINT ( 'NONE',  ( -0.4501900775161314372, 1.384563962073082966, 3.911202265604141193 ) ) ;
#82449=EDGE_CURVE ( 'NONE', #13017, #82375, #59453, .T. ) ;
#82455=CARTESIAN_POINT ( 'NONE',  ( -3.909771271330827691, 1.429805566235350378, 0.4623082157241558687 ) ) ;
#82460=ORIENTED_EDGE ( 'NONE', *, *, #41491, .T. ) ;
#82461=DIRECTION ( 'NONE',  ( -0.000000000000000000, 1.000000000000000000, -0.000000000000000000 ) ) ;
#82466=DIRECTION ( 'NONE',  ( 0.000000000000000000, 0.000000000000000000, -1.000000000000000000 ) ) ;
#82476=VERTEX_POINT ( 'NONE', #25874 ) ;
#82481=CIRCLE ( 'NONE', #47503, 3.937007874015748143 ) ;
#82524=CARTESIAN_POINT ( 'NONE',  ( -2.860656214895221261, 1.077434660671925393, -0.1173752429317476975 ) ) ;
#82537=CARTESIAN_POINT ( 'NONE',  ( 1.403614904275686858E-14, 1.537401574803149984, -3.937007874015761910 ) ) ;
#82539=CIRCLE ( 'NONE', #48944, 1.122047244094488194 ) ;
#82541=CARTESIAN_POINT ( 'NONE',  ( 0.000000000000000000, 2.755905511811024056, 0.000000000000000000 ) ) ;
#82546=DIRECTION ( 'NONE',  ( 0.000000000000000000, 0.000000000000000000, -1.000000000000000000 ) ) ;
#82550=AXIS2_PLACEMENT_3D ( 'NONE', #21871, #74060, #10082 ) ;
#82563=DIRECTION ( 'NONE',  ( -0.000000000000000000, -1.000000000000000000, -0.000000000000000000 ) ) ;
#82582=CARTESIAN_POINT ( 'NONE',  ( -1.016821367227983997, 1.537401574803149984, 0.4744094488188970171 ) ) ;
#82583=CARTESIAN_POINT ( 'NONE',  ( -0.06818963398611965765, 1.067605756753705393, -1.854667707163995871 ) ) ;
#82584=ORIENTED_EDGE ( 'NONE', *, *, #56851, .F. ) ;
#82590=ADVANCED_FACE ( 'NONE', ( #52373 ), #63778, .F. ) ;
#82597=CIRCLE ( 'NONE', #57038, 1.929133858267716661 ) ;
#82602=CARTESIAN_POINT ( 'NONE',  ( 0.000000000000000000, 2.716535433070866645, 0.000000000000000000 ) ) ;
#82606=ORIENTED_EDGE ( 'NONE', *, *, #32173, .T. ) ;
#82610=DIRECTION ( 'NONE',  ( -0.000000000000000000, -1.000000000000000000, -0.000000000000000000 ) ) ;
#82613=AXIS2_PLACEMENT_3D ( 'NONE', #10536, #30281, #36192 ) ;
#82624=EDGE_CURVE ( 'NONE', #67465, #37133, #77663, .T. ) ;
#82629=CARTESIAN_POINT ( 'NONE',  ( -0.03412294937774069253, 1.063915752041794782, 1.851250178557425130 ) ) ;
#82633=EDGE_CURVE ( 'NONE', #12200, #66338, #4601, .T. ) ;
#82644=CARTESIAN_POINT ( 'NONE',  ( 2.620897244026417994, 1.710976477253048023, 0.4417575354491489747 ) ) ;
#82661=VERTEX_POINT ( 'NONE', #76819 ) ;
#82673=DIRECTION ( 'NONE',  ( -0.000000000000000000, -1.000000000000000000, -0.000000000000000000 ) ) ;
#82674=CARTESIAN_POINT ( 'NONE',  ( 3.909863570149732848, 1.648352784150537875, 0.4615281897282089152 ) ) ;
#82691=CARTESIAN_POINT ( 'NONE',  ( -0.5314960629921349211, 2.716535433070866645, 2.543486866223387377 ) ) ;
#82716=VERTEX_POINT ( 'NONE', #77239 ) ;
#82717=LINE ( 'NONE', #68853, #67614 ) ;
#82720=PLANE ( 'NONE',  #22356 ) ;
#82724=VECTOR ( 'NONE', #22773, 39.37007874015748143 ) ;
#82725=VERTEX_POINT ( 'NONE', #32200 ) ;
#82727=CYLINDRICAL_SURFACE ( 'NONE', #62693, 0.4744094488188972947 ) ;
#82757=CIRCLE ( 'NONE', #2145, 0.01968503937007875723 ) ;
#82765=DIRECTION ( 'NONE',  ( 0.000000000000000000, 0.000000000000000000, -1.000000000000000000 ) ) ;
#82772=EDGE_CURVE ( 'NONE', #33187, #82725, #12722, .T. ) ;
#82792=ORIENTED_EDGE ( 'NONE', *, *, #78455, .F. ) ;
#82801=CARTESIAN_POINT ( 'NONE',  ( 2.503252890251015828, 2.755905511811024056, -0.5314960629921260393 ) ) ;
#82822=AXIS2_PLACEMENT_3D ( 'NONE', #67634, #80686, #48665 ) ;
#82826=CIRCLE ( 'NONE', #10260, 3.405511811023621771 ) ;
#82827=AXIS2_PLACEMENT_3D ( 'NONE', #39253, #59448, #71670 ) ;
#82843=CARTESIAN_POINT ( 'NONE',  ( 2.583694225513480713, 2.755905511811024056, 0.5314960629921260393 ) ) ;
#82847=DIRECTION ( 'NONE',  ( 0.000000000000000000, -1.000000000000000000, 0.000000000000000000 ) ) ;
#82862=CARTESIAN_POINT ( 'NONE',  ( -3.936634651216008418, 1.066061182819163955, 0.06215626018321074309 ) ) ;
#82868=ORIENTED_EDGE ( 'NONE', *, *, #57258, .T. ) ;
#82874=EDGE_CURVE ( 'NONE', #26552, #24203, #14314, .T. ) ;
#82879=CIRCLE ( 'NONE', #60058, 0.09842519685039351207 ) ;
#82886=ORIENTED_EDGE ( 'NONE', *, *, #63426, .F. ) ;
#82903=CARTESIAN_POINT ( 'NONE',  ( 2.593372381816078764, 1.408244132531268011, -0.4567322424080935139 ) ) ;
#82913=EDGE_CURVE ( 'NONE', #49776, #25136, #70504, .T. ) ;
#82934=FACE_OUTER_BOUND ( 'NONE', #53056, .T. ) ;
#82941=CIRCLE ( 'NONE', #14418, 1.929133858267716661 ) ;
#82942=AXIS2_PLACEMENT_3D ( 'NONE', #70455, #12813, #51492 ) ;
#82953=CARTESIAN_POINT ( 'NONE',  ( 0.4741766535082888590, 1.520234135998520753, -2.169568943720849852 ) ) ;
#82970=LINE ( 'NONE', #1318, #82117 ) ;
#82971=FACE_OUTER_BOUND ( 'NONE', #74428, .T. ) ;
#82984=DIRECTION ( 'NONE',  ( 0.000000000000000000, 1.000000000000000000, 0.000000000000000000 ) ) ;
#82996=ORIENTED_EDGE ( 'NONE', *, *, #50355, .T. ) ;
#82999=ORIENTED_EDGE ( 'NONE', *, *, #78384, .F. ) ;
#83011=DIRECTION ( 'NONE',  ( 0.000000000000000000, -0.000000000000000000, 1.000000000000000000 ) ) ;
#83022=CARTESIAN_POINT ( 'NONE',  ( 2.154527559055120278, 0.03937007874015747977, -0.4677827689124846589 ) ) ;
#83038=EDGE_CURVE ( 'NONE', #58442, #16468, #83138, .T. ) ;
#83040=LINE ( 'NONE', #77143, #78877 ) ;
#83045=CYLINDRICAL_SURFACE ( 'NONE', #66681, 0.4744094488188972947 ) ;
#83055=AXIS2_PLACEMENT_3D ( 'NONE', #56848, #44621, #82546 ) ;
#83060=EDGE_CURVE ( 'NONE', #74617, #36894, #63478, .T. ) ;
#83070=EDGE_CURVE ( 'NONE', #65458, #9504, #18076, .T. ) ;
#83084=CARTESIAN_POINT ( 'NONE',  ( 1.579022939845507243E-16, 0.000000000000000000, 1.289370078740159409 ) ) ;
#83089=EDGE_CURVE ( 'NONE', #52887, #65211, #74258, .T. ) ;
#83098=EDGE_CURVE ( 'NONE', #72978, #8695, #43582, .T. ) ;
#83121=CARTESIAN_POINT ( 'NONE',  ( -0.5314960629921147151, 2.716535433070866645, -3.224202737261816942 ) ) ;
#83122=CARTESIAN_POINT ( 'NONE',  ( -0.5314960629921148261, 2.755905511811024056, -3.184294706754632109 ) ) ;
#83129=ORIENTED_EDGE ( 'NONE', *, *, #50047, .F. ) ;
#83130=CARTESIAN_POINT ( 'NONE',  ( 0.000000000000000000, 2.755905511811024056, 0.000000000000000000 ) ) ;
#83133=CARTESIAN_POINT ( 'NONE',  ( 0.000000000000000000, 0.04488074079120789317, 0.000000000000000000 ) ) ;
#83138=LINE ( 'NONE', #46064, #54354 ) ;
#83139=DIRECTION ( 'NONE',  ( 0.000000000000000000, 1.000000000000000000, 0.000000000000000000 ) ) ;
#83165=ORIENTED_EDGE ( 'NONE', *, *, #6973, .F. ) ;
#83179=CARTESIAN_POINT ( 'NONE',  ( 0.3812543623607845822, 1.253662731238191830, 2.704545108238443962 ) ) ;
#83189=FACE_OUTER_BOUND ( 'NONE', #33113, .T. ) ;
#83209=DIRECTION ( 'NONE',  ( -0.000000000000000000, 1.000000000000000000, -0.000000000000000000 ) ) ;
#83217=DIRECTION ( 'NONE',  ( 0.000000000000000000, 0.000000000000000000, -1.000000000000000000 ) ) ;
#83225=DIRECTION ( 'NONE',  ( -0.8660254037844432595, 0.000000000000000000, 0.4999999999999918954 ) ) ;
#83226=ORIENTED_EDGE ( 'NONE', *, *, #7150, .F. ) ;
#83233=CARTESIAN_POINT ( 'NONE',  ( 1.916165371950980356, 1.134815007188461289, 0.2514610820057225360 ) ) ;
#83235=CARTESIAN_POINT ( 'NONE',  ( -1.895394334970792016, 2.755905511811024056, 0.5314960629921260393 ) ) ;
#83272=CARTESIAN_POINT ( 'NONE',  ( 0.000000000000000000, 1.724409448818897461, 0.000000000000000000 ) ) ;
#83288=CARTESIAN_POINT ( 'NONE',  ( 6.267877318470705905E-17, 1.929133858267716661, 2.874015748031495843 ) ) ;
#83294=ORIENTED_EDGE ( 'NONE', *, *, #11630, .T. ) ;
#83295=B_SPLINE_CURVE_WITH_KNOTS ( 'NONE', 3,
 ( #23699, #49370, #37158, #61597 ),
 .UNSPECIFIED., .F., .F.,
 ( 4, 4 ),
 ( 0.05078239113848885544, 0.05222574548756819812 ),
 .UNSPECIFIED. ) ;
ENDSEC;
END-ISO-10303-21;
